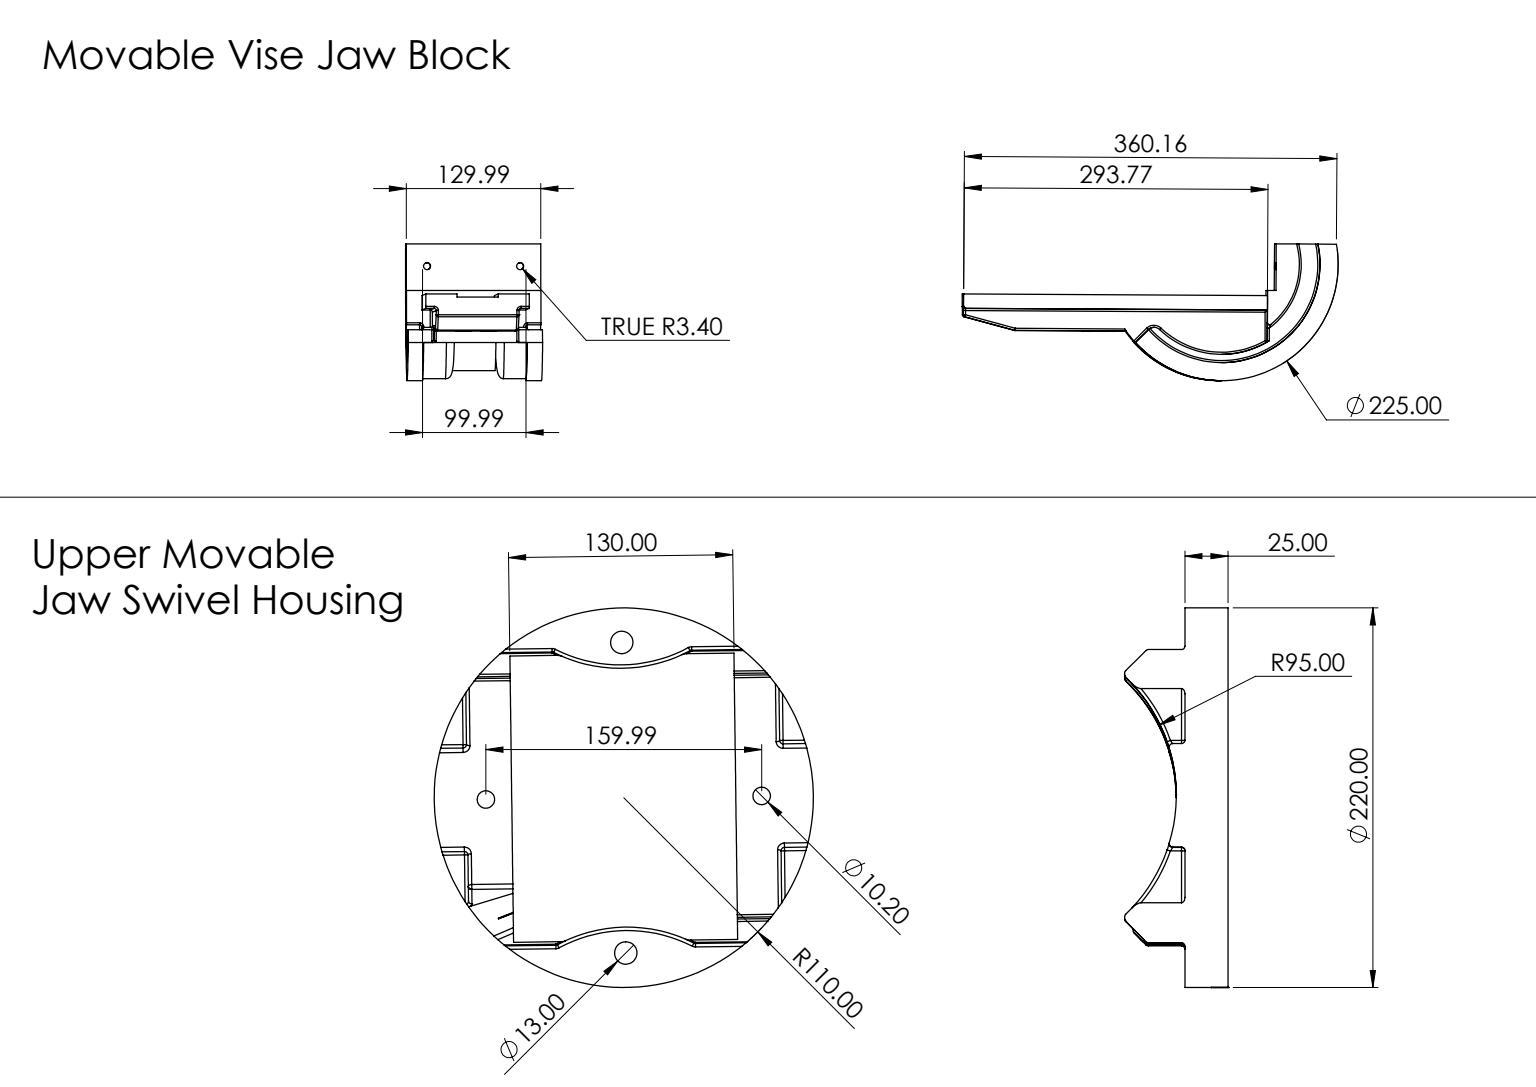
ISO-10303-21;
HEADER;
FILE_DESCRIPTION (('STEP AP214'),
    '1' );
FILE_NAME ('Upper Movable Jaw Swivel Housing.step',
    '2026-10-09T10:51:02',
    ( '' ),
    ( '' ),
    'SwSTEP 2.0',
    'SolidWorks 2026',
    '' );
FILE_SCHEMA (( 'AUTOMOTIVE_DESIGN' ));
ENDSEC;

DATA;
#10=CARTESIAN_POINT ( 'NONE',  ( -89.78468759032787716, 88.98018858692468314, 52.07678711320818365 ) ) ;
#12=VERTEX_POINT ( 'NONE', #2655 ) ;
#19=CARTESIAN_POINT ( 'NONE',  ( 83.88156715903123484, 75.05939835648034375, 2.283427986461537440 ) ) ;
#21=EDGE_LOOP ( 'NONE', ( #14279, #17712, #11551, #2632 ) ) ;
#25=CARTESIAN_POINT ( 'NONE',  ( -76.57490387278154742, 75.07748563434969924, 4.833641046600559044 ) ) ;
#28=CARTESIAN_POINT ( 'NONE',  ( -105.7487010638476619, 78.91327849199103639, 30.28586431387788380 ) ) ;
#37=DIRECTION ( 'NONE',  ( 6.641024085592512675E-15, -1.000000000000000000, 3.383900228611897455E-15 ) ) ;
#42=AXIS2_PLACEMENT_3D ( 'NONE', #16731, #4517, #8084 ) ;
#44=VERTEX_POINT ( 'NONE', #20325 ) ;
#50=AXIS2_PLACEMENT_3D ( 'NONE', #20682, #18849, #13474 ) ;
#51=CARTESIAN_POINT ( 'NONE',  ( -93.23587179807654479, 72.00000000000000000, -30.79757858250320979 ) ) ;
#57=CARTESIAN_POINT ( 'NONE',  ( 1.364373935098378649E-14, 105.0000000000000000, -9.836450281572198869E-15 ) ) ;
#58=EDGE_CURVE ( 'NONE', #6274, #3568, #1285, .T. ) ;
#59=CARTESIAN_POINT ( 'NONE',  ( 93.17671387018316409, 79.04398536104964990, 26.22064129356684958 ) ) ;
#65=EDGE_LOOP ( 'NONE', ( #10795, #9717, #10945, #15498 ) ) ;
#67=CARTESIAN_POINT ( 'NONE',  ( -92.91045972105430906, 79.04398536109844997, -26.22408268756080929 ) ) ;
#70=VECTOR ( 'NONE', #5389, 1000.000000000000000 ) ;
#71=CARTESIAN_POINT ( 'NONE',  ( -69.75324274910623501, 70.27959272172267902, -85.05633583411399457 ) ) ;
#84=VECTOR ( 'NONE', #2049, 1000.000000000000114 ) ;
#86=CARTESIAN_POINT ( 'NONE',  ( 70.93357090261925180, 91.46354453597338363, 84.07396062241133450 ) ) ;
#94=CARTESIAN_POINT ( 'NONE',  ( 87.98413419613014241, 100.6041916471018851, -66.02114910964037620 ) ) ;
#106=EDGE_CURVE ( 'NONE', #7605, #5654, #6985, .T. ) ;
#112=DIRECTION ( 'NONE',  ( 2.025474946048326158E-22, -1.000000000000000000, 1.876735158486679638E-22 ) ) ;
#114=DIRECTION ( 'NONE',  ( -0.9999164797902015955, -2.001050586450178695E-22, 0.01292414190464131335 ) ) ;
#133=CARTESIAN_POINT ( 'NONE',  ( -88.16866694100703228, 88.68864517119313007, 52.43947707082220688 ) ) ;
#142=CARTESIAN_POINT ( 'NONE',  ( 80.59620023633263486, 75.13519862315604314, -6.109066223056235145 ) ) ;
#146=ORIENTED_EDGE ( 'NONE', *, *, #11899, .T. ) ;
#157=PLANE ( 'NONE',  #21075 ) ;
#159=CARTESIAN_POINT ( 'NONE',  ( 105.4334892372614689, 71.72994009789539405, -31.36525700924963544 ) ) ;
#171=CARTESIAN_POINT ( 'NONE',  ( -90.06393689865117835, 72.00000000000000000, 59.85988923254397065 ) ) ;
#176=FACE_OUTER_BOUND ( 'NONE', #6477, .T. ) ;
#182=CARTESIAN_POINT ( 'NONE',  ( 92.53737097235195108, 79.85828562204582681, 28.87839056718317465 ) ) ;
#188=CARTESIAN_POINT ( 'NONE',  ( -92.67786813602107543, 77.16999450923083259, -28.87226322141232870 ) ) ;
#189=ORIENTED_EDGE ( 'NONE', *, *, #8901, .F. ) ;
#197=CARTESIAN_POINT ( 'NONE',  ( 1.163172771417732010, 44.99899999999999523, 89.99248318111813205 ) ) ;
#198=VERTEX_POINT ( 'NONE', #22578 ) ;
#202=CARTESIAN_POINT ( 'NONE',  ( -39.36913080622078809, 72.00000000000000000, 87.51612159803859470 ) ) ;
#204=CARTESIAN_POINT ( 'NONE',  ( -90.61229378181283778, 77.84360403296375353, 32.30868923918552582 ) ) ;
#214=EDGE_LOOP ( 'NONE', ( #14788, #8184, #10598, #16060, #20937 ) ) ;
#218=CARTESIAN_POINT ( 'NONE',  ( 36.24790013166018099, 94.37751527644310556, 82.16087381192814121 ) ) ;
#219=EDGE_CURVE ( 'NONE', #11742, #21224, #10193, .T. ) ;
#222=CYLINDRICAL_SURFACE ( 'NONE', #2944, 2.000000000000001776 ) ;
#226=CARTESIAN_POINT ( 'NONE',  ( -41.56623493000981284, 72.00000000000000000, -82.46967996629571473 ) ) ;
#230=CARTESIAN_POINT ( 'NONE',  ( 39.42082737383937996, 91.17157287525387233, -83.51645567887783272 ) ) ;
#231=ORIENTED_EDGE ( 'NONE', *, *, #5950, .F. ) ;
#232=CARTESIAN_POINT ( 'NONE',  ( 106.2491592972476298, 77.90302844854615216, 28.48020057081471279 ) ) ;
#235=EDGE_CURVE ( 'NONE', #9934, #22618, #12029, .T. ) ;
#236=EDGE_LOOP ( 'NONE', ( #19815, #2984, #795, #12420, #9588 ) ) ;
#240=EDGE_CURVE ( 'NONE', #22376, #21368, #5043, .T. ) ;
#243=CARTESIAN_POINT ( 'NONE',  ( -89.64611244253616462, 89.06139627483084098, 51.86061978640490366 ) ) ;
#247=EDGE_CURVE ( 'NONE', #11011, #13307, #20124, .T. ) ;
#253=CARTESIAN_POINT ( 'NONE',  ( -90.15100670864553933, 87.99029836822313655, 53.12346227685477373 ) ) ;
#265=CARTESIAN_POINT ( 'NONE',  ( 105.3069082217399597, 70.76149960027359498, -31.78775043357529739 ) ) ;
#271=EDGE_LOOP ( 'NONE', ( #6417, #19362, #17256, #12411 ) ) ;
#277=DIRECTION ( 'NONE',  ( 0.9999164797902017066, 2.001050586450178931E-22, -0.01292414190464131508 ) ) ;
#278=CARTESIAN_POINT ( 'NONE',  ( -91.88175745861167343, 69.99999999999998579, 60.48014731673399069 ) ) ;
#284=CARTESIAN_POINT ( 'NONE',  ( 90.70439626174579928, 79.29995750804924626, 27.08818539008225912 ) ) ;
#285=CARTESIAN_POINT ( 'NONE',  ( 90.15711184568685610, 79.46353706204938305, 27.61532001585838714 ) ) ;
#288=CIRCLE ( 'NONE', #22624, 0.009999999999999205705 ) ;
#289=ADVANCED_FACE ( 'NONE', ( #16063 ), #9015, .T. ) ;
#314=CARTESIAN_POINT ( 'NONE',  ( -91.08520856931303911, 77.44390114805533187, 31.69197020849769686 ) ) ;
#316=ORIENTED_EDGE ( 'NONE', *, *, #15570, .F. ) ;
#319=ADVANCED_FACE ( 'NONE', ( #17546 ), #8781, .T. ) ;
#325=DIRECTION ( 'NONE',  ( 0.01292414190464174703, 0.000000000000000000, 0.9999164797902015955 ) ) ;
#326=( BOUNDED_SURFACE ( )  B_SPLINE_SURFACE ( 3, 2, ( 
 ( #2487, #894, #11567 ),
 ( #1117, #14687, #22097 ),
 ( #11112, #18134, #9486 ),
 ( #2827, #8113, #7770 ),
 ( #14809, #13081, #4304 ),
 ( #11333, #16646, #14924 ),
 ( #998, #21864, #6160 ),
 ( #13185, #2385, #20151 ),
 ( #18461, #2723, #4540 ),
 ( #9377, #16853, #16751 ),
 ( #15145, #7985, #15025 ),
 ( #21979, #6279, #13305 ),
 ( #6398, #19810, #16411 ),
 ( #10404, #6504, #1347 ),
 ( #4752, #11794, #13518 ),
 ( #6725, #18893, #10288 ),
 ( #3156, #15697, #11911 ),
 ( #15366, #3390, #10171 ) ),
 .UNSPECIFIED., .F., .F., .T. ) 
 B_SPLINE_SURFACE_WITH_KNOTS ( ( 4, 2, 2, 2, 2, 2, 2, 2, 4 ),
 ( 3, 3 ),
 ( 0.002597246120634449582, 0.003399884678228176898, 0.004202523235821904214, 0.005005161793415631097, 0.005807800351009358847, 0.006610438908603086597, 0.007413077466196813479, 0.008215716023790540362, 0.009018354581384268112 ),
 ( 0.000000000000000000, 1.000000000000000000 ),
 .UNSPECIFIED. ) 
 GEOMETRIC_REPRESENTATION_ITEM ( )  RATIONAL_B_SPLINE_SURFACE ( (
 ( 1.000000000000000000, 0.5963808372950818448, 1.000000000000000000),
 ( 1.000000000000000000, 0.5963839598475944026, 1.000000000000000000),
 ( 1.000000000000000000, 0.5970886094881097117, 1.000000000000000000),
 ( 1.000000000000000000, 0.5998681984912884735, 1.000000000000000000),
 ( 1.000000000000000000, 0.6019790828716350406, 1.000000000000000000),
 ( 1.000000000000000000, 0.6074656362385489894, 1.000000000000000000),
 ( 1.000000000000000000, 0.6108290540004600588, 1.000000000000000000),
 ( 1.000000000000000000, 0.6188252630046860991, 1.000000000000000000),
 ( 1.000000000000000000, 0.6234423941984682527, 1.000000000000000000),
 ( 1.000000000000000000, 0.6335838931037546251, 1.000000000000000000),
 ( 1.000000000000000000, 0.6391861101558512503, 1.000000000000000000),
 ( 1.000000000000000000, 0.6512661799274815921, 1.000000000000000000),
 ( 1.000000000000000000, 0.6576333021889211317, 1.000000000000000000),
 ( 1.000000000000000000, 0.6710088154584188391, 1.000000000000000000),
 ( 1.000000000000000000, 0.6780884601156443869, 1.000000000000000000),
 ( 1.000000000000000000, 0.6924279500034885571, 1.000000000000000000),
 ( 1.000000000000000000, 0.6997125326201816264, 1.000000000000000000),
 ( 1.000000000000000000, 0.7071067811865476838, 1.000000000000000000) ) ) 
 REPRESENTATION_ITEM ( '' )  SURFACE ( )  );
#331=DIRECTION ( 'NONE',  ( 2.025474946048326158E-22, -1.000000000000000000, 1.876735158486679638E-22 ) ) ;
#334=ORIENTED_EDGE ( 'NONE', *, *, #20168, .F. ) ;
#354=CARTESIAN_POINT ( 'NONE',  ( -89.81089220510853011, 88.95379388444949598, 52.12444704693557895 ) ) ;
#356=ORIENTED_EDGE ( 'NONE', *, *, #20168, .T. ) ;
#367=VERTEX_POINT ( 'NONE', #15252 ) ;
#369=VERTEX_POINT ( 'NONE', #17174 ) ;
#371=CARTESIAN_POINT ( 'NONE',  ( -93.21002351426726307, 77.12912189496638860, -28.79774562292281104 ) ) ;
#387=ORIENTED_EDGE ( 'NONE', *, *, #12460, .T. ) ;
#390=DIRECTION ( 'NONE',  ( 0.01292414190464223969, 1.902755938799532355E-22, 0.9999164797902017066 ) ) ;
#392=CARTESIAN_POINT ( 'NONE',  ( 91.23603883849617091, 72.00000000000000000, 30.82342686631245243 ) ) ;
#393=CARTESIAN_POINT ( 'NONE',  ( -36.73936676148915126, 94.93197183469659706, -81.60001862646660697 ) ) ;
#396=EDGE_CURVE ( 'NONE', #4308, #9861, #9699, .T. ) ;
#397=CARTESIAN_POINT ( 'NONE',  ( 106.2089377515399065, 34.61572286322119396, 28.62973177816241588 ) ) ;
#400=CARTESIAN_POINT ( 'NONE',  ( 89.22767861003023881, 80.31838830481380853, 30.18953644180654550 ) ) ;
#403=CARTESIAN_POINT ( 'NONE',  ( 90.51972003054841309, 79.34791451281842001, 27.24428967784124822 ) ) ;
#405=CARTESIAN_POINT ( 'NONE',  ( -90.43474204040838060, 34.61572286322119396, 31.17139488067998343 ) ) ;
#412=CARTESIAN_POINT ( 'NONE',  ( -92.63973831233892042, 79.05196971970110553, -26.25410855708505409 ) ) ;
#419=DIRECTION ( 'NONE',  ( 0.01292414190464174703, 0.000000000000000000, 0.9999164797902015955 ) ) ;
#421=B_SPLINE_CURVE_WITH_KNOTS ( 'NONE', 3,
 ( #14409, #16130, #12222, #12679, #7032, #7150, #17960, #15907, #14177, #10490, #10589, #5523, #10835, #2094, #19205, #17501, #21045, #3916, #2196, #14060, #5402, #19548, #5298, #3815, #12338, #1753, #8731, #9199, #15785, #25, #12439, #17614, #19428, #19318, #3578, #7364, #16247, #488, #13932, #20926 ),
 .UNSPECIFIED., .F., .F.,
 ( 4, 2, 2, 2, 2, 2, 2, 2, 2, 2, 2, 2, 2, 2, 2, 2, 2, 2, 2, 4 ),
 ( 0.000000000000000000, 0.0009967370484891052360, 0.001495105572733637905, 0.001993474096978170573, 0.002990211145467237645, 0.003986948193956304717, 0.004983685242445371789, 0.005980422290934439729, 0.006977159339423508536, 0.007973896387912576475, 0.008970633436401644414, 0.009967370484890712354, 0.01046573900913524806, 0.01096410753337978203, 0.01196084458186887425, 0.01295758163035796821, 0.01345595015460251433, 0.01395431867884706391, 0.01495105572733619430, 0.01594779277582532642 ),
 .UNSPECIFIED. ) ;
#423=EDGE_CURVE ( 'NONE', #8239, #10113, #17733, .T. ) ;
#430=CARTESIAN_POINT ( 'NONE',  ( 67.52146002153375548, 70.28876377827108968, -86.83823687282567505 ) ) ;
#432=CARTESIAN_POINT ( 'NONE',  ( -91.92966151681214626, 79.05204536692272654, 28.63995821788555318 ) ) ;
#433=DIRECTION ( 'NONE',  ( -0.009138748381789112835, -0.7071067811865462405, -0.7070477234798343558 ) ) ;
#450=DIRECTION ( 'NONE',  ( 0.9999164797902015955, 2.001050586450177755E-22, -0.01292414190464177999 ) ) ;
#453=SPHERICAL_SURFACE ( 'NONE', #18447, 2.000000000000000000 ) ;
#462=CARTESIAN_POINT ( 'NONE',  ( 33.37693045445141138, 92.26126280267001789, 80.91304515629593652 ) ) ;
#464=( BOUNDED_CURVE ( )  B_SPLINE_CURVE ( 3, ( #5130, #22567, #8806, #20870 ),
 .UNSPECIFIED., .F., .T. ) 
 B_SPLINE_CURVE_WITH_KNOTS ( ( 4, 4 ),
 ( 0.4229686233981272414, 0.4841788640348457240 ),
 .UNSPECIFIED. ) 
 CURVE ( )  GEOMETRIC_REPRESENTATION_ITEM ( )  RATIONAL_B_SPLINE_CURVE ( ( 1.000000000000000000, 0.9996877999070342691, 0.9996877999070342691, 1.000000000000000000 ) ) 
 REPRESENTATION_ITEM ( '' )  );
#469=ORIENTED_EDGE ( 'NONE', *, *, #9836, .T. ) ;
#471=CARTESIAN_POINT ( 'NONE',  ( -88.41249021357108973, 88.83782181376912490, 50.51791556700484165 ) ) ;
#474=ORIENTED_EDGE ( 'NONE', *, *, #3932, .F. ) ;
#476=ORIENTED_EDGE ( 'NONE', *, *, #5316, .T. ) ;
#477=CARTESIAN_POINT ( 'NONE',  ( 1.079165849037564184, 44.99899999999999523, 83.49302606248181746 ) ) ;
#482=CARTESIAN_POINT ( 'NONE',  ( -91.45377919752192497, 96.73472523270000067, -61.12462174243600543 ) ) ;
#488=CARTESIAN_POINT ( 'NONE',  ( -79.25692431500161206, 75.13518351147564545, 6.091477897721252255 ) ) ;
#491=ORIENTED_EDGE ( 'NONE', *, *, #17530, .T. ) ;
#493=CARTESIAN_POINT ( 'NONE',  ( -14.05322407132952733, 63.29827626019820741, -14.85614898258057082 ) ) ;
#495=VERTEX_POINT ( 'NONE', #14623 ) ;
#496=EDGE_CURVE ( 'NONE', #21893, #14619, #12233, .T. ) ;
#503=CARTESIAN_POINT ( 'NONE',  ( -105.3515605809558195, 70.97896074530378030, 31.63944816216639211 ) ) ;
#507=CARTESIAN_POINT ( 'NONE',  ( 64.99457118636311748, 105.0000000000000000, -0.8400692238016954638 ) ) ;
#510=EDGE_CURVE ( 'NONE', #4157, #19786, #3544, .T. ) ;
#521=CIRCLE ( 'NONE', #1629, 1.999999999999999112 ) ;
#527=EDGE_LOOP ( 'NONE', ( #22645, #19170, #20971, #3651 ) ) ;
#529=FACE_OUTER_BOUND ( 'NONE', #7929, .T. ) ;
#531=CARTESIAN_POINT ( 'NONE',  ( -70.91392079944854743, 72.00000000000000000, -84.09052168258642723 ) ) ;
#541=EDGE_CURVE ( 'NONE', #17177, #9516, #1391, .T. ) ;
#542=ORIENTED_EDGE ( 'NONE', *, *, #423, .F. ) ;
#550=CARTESIAN_POINT ( 'NONE',  ( -90.51365344713411787, 78.00107869518899406, 32.54507930669932847 ) ) ;
#554=CIRCLE ( 'NONE', #5300, 2.000000000000001332 ) ;
#562=ORIENTED_EDGE ( 'NONE', *, *, #13386, .T. ) ;
#567=VERTEX_POINT ( 'NONE', #9777 ) ;
#571=B_SPLINE_CURVE_WITH_KNOTS ( 'NONE', 3,
 ( #10519, #14093, #4058, #7523, #13059, #2579, #6135, #8528, #22192, #20710, #11994, #22553 ),
 .UNSPECIFIED., .F., .F.,
 ( 4, 2, 2, 2, 2, 4 ),
 ( 0.000000000000000000, 0.0007983727002588449344, 0.001596745400517689869, 0.003193490801035376702, 0.004790236201553063969, 0.006386981602070762078 ),
 .UNSPECIFIED. ) ;
#572=ORIENTED_EDGE ( 'NONE', *, *, #22537, .F. ) ;
#575=DIRECTION ( 'NONE',  ( 0.01292414190464179213, 0.000000000000000000, 0.9999164797902017066 ) ) ;
#577=DIRECTION ( 'NONE',  ( 0.8585559824929073214, 0.4417096956421488474, -0.2603347262686231400 ) ) ;
#578=AXIS2_PLACEMENT_3D ( 'NONE', #9864, #20311, #8020 ) ;
#580=CARTESIAN_POINT ( 'NONE',  ( 92.43457499998882554, 79.86121811340028387, -31.19724316448930423 ) ) ;
#586=ORIENTED_EDGE ( 'NONE', *, *, #9607, .F. ) ;
#588=CARTESIAN_POINT ( 'NONE',  ( -88.17180307448359144, 88.85327758763604322, 52.12627907722180254 ) ) ;
#591=VERTEX_POINT ( 'NONE', #17124 ) ;
#600=ORIENTED_EDGE ( 'NONE', *, *, #3820, .F. ) ;
#601=CARTESIAN_POINT ( 'NONE',  ( 92.13597290369317250, 77.31823782845360427, 29.12178019517720884 ) ) ;
#602=ORIENTED_EDGE ( 'NONE', *, *, #541, .F. ) ;
#613=FACE_OUTER_BOUND ( 'NONE', #11627, .T. ) ;
#615=ORIENTED_EDGE ( 'NONE', *, *, #11170, .T. ) ;
#616=CARTESIAN_POINT ( 'NONE',  ( -84.91224671543740499, 75.00866199770878495, 2.421235374481680136 ) ) ;
#618=CARTESIAN_POINT ( 'NONE',  ( -88.16310690832857233, 88.22405785602812500, 52.94336900718522543 ) ) ;
#623=CARTESIAN_POINT ( 'NONE',  ( 41.56623493000984126, 69.99999999999998579, 82.46967996629570052 ) ) ;
#624=CARTESIAN_POINT ( 'NONE',  ( -41.01898768785987670, 92.04141378167193466, -84.43550307159648582 ) ) ;
#626=CARTESIAN_POINT ( 'NONE',  ( 93.23587179807657321, 69.99999999999998579, 30.79757858250317781 ) ) ;
#627=LINE ( 'NONE', #11303, #11518 ) ;
#629=CARTESIAN_POINT ( 'NONE',  ( 81.70668847916368804, 104.4142135623730780, -73.64792636435126383 ) ) ;
#644=CARTESIAN_POINT ( 'NONE',  ( -88.92875819446121000, 70.43566758519529003, 63.01298426280252585 ) ) ;
#647=ADVANCED_FACE ( 'NONE', ( #18837 ), #13561, .F. ) ;
#657=DIRECTION ( 'NONE',  ( 0.9999164797902015955, 2.001050586450178695E-22, -0.01292414190464131335 ) ) ;
#659=CARTESIAN_POINT ( 'NONE',  ( -90.46145803317399725, 80.27058204906346361, 32.37524683357860056 ) ) ;
#661=ORIENTED_EDGE ( 'NONE', *, *, #9836, .F. ) ;
#668=CARTESIAN_POINT ( 'NONE',  ( -90.40889375659909888, 78.43035437438882695, 33.17122784026039994 ) ) ;
#672=EDGE_CURVE ( 'NONE', #7269, #15892, #7114, .T. ) ;
#677=CARTESIAN_POINT ( 'NONE',  ( -85.63433794141032251, 105.0000000000000000, -69.04172771111927887 ) ) ;
#685=ORIENTED_EDGE ( 'NONE', *, *, #18084, .T. ) ;
#686=PLANE ( 'NONE',  #15863 ) ;
#689=CARTESIAN_POINT ( 'NONE',  ( 35.95309506732430549, 93.50464841319750064, 82.03286182426640494 ) ) ;
#692=DIRECTION ( 'NONE',  ( -0.9999164797902015955, -2.001050586450178695E-22, 0.01292414190464131335 ) ) ;
#694=ORIENTED_EDGE ( 'NONE', *, *, #2604, .T. ) ;
#696=DIRECTION ( 'NONE',  ( 0.9999164797902017066, 0.000000000000000000, -0.01292414190464174703 ) ) ;
#697=CARTESIAN_POINT ( 'NONE',  ( -88.29917401736820182, 88.77742970155978242, 50.41907810135165846 ) ) ;
#699=AXIS2_PLACEMENT_3D ( 'NONE', #1518, #3671, #16004 ) ;
#702=CARTESIAN_POINT ( 'NONE',  ( -91.00106904273528130, 70.29040131071506892, 61.79648398638329354 ) ) ;
#708=CARTESIAN_POINT ( 'NONE',  ( 69.24448582912822303, 92.41827837429551096, -85.47053766693686327 ) ) ;
#709=ORIENTED_EDGE ( 'NONE', *, *, #772, .F. ) ;
#711=DIRECTION ( 'NONE',  ( -0.01292414190464269072, 0.000000000000000000, -0.9999164797902017066 ) ) ;
#722=FACE_OUTER_BOUND ( 'NONE', #6782, .T. ) ;
#723=DIRECTION ( 'NONE',  ( 0.9999164797902015955, 2.001050586450178695E-22, -0.01292414190464131335 ) ) ;
#729=CARTESIAN_POINT ( 'NONE',  ( -85.06887357168608332, 75.00176710950381676, 0.4346775517040236680 ) ) ;
#732=ORIENTED_EDGE ( 'NONE', *, *, #9607, .T. ) ;
#733=ORIENTED_EDGE ( 'NONE', *, *, #1086, .F. ) ;
#736=DIRECTION ( 'NONE',  ( 0.01292414190463832269, 0.000000000000000000, 0.9999164797902017066 ) ) ;
#739=DIRECTION ( 'NONE',  ( -0.9999164797902017066, -2.001050586450178931E-22, 0.01292414190464131508 ) ) ;
#740=CARTESIAN_POINT ( 'NONE',  ( -38.37734285177536009, 94.19957547782772167, -82.31130495469157893 ) ) ;
#750=AXIS2_PLACEMENT_3D ( 'NONE', #20210, #20433, #18609 ) ;
#755=ORIENTED_EDGE ( 'NONE', *, *, #16128, .F. ) ;
#758=ORIENTED_EDGE ( 'NONE', *, *, #13735, .T. ) ;
#760=CARTESIAN_POINT ( 'NONE',  ( 77.23768650000880598, 75.09868225356437677, -5.328640597094168818 ) ) ;
#762=CIRCLE ( 'NONE', #16898, 109.9999999999999858 ) ;
#767=CARTESIAN_POINT ( 'NONE',  ( -68.86686855361774917, 91.87224768293378929, 85.77506393453893452 ) ) ;
#769=CARTESIAN_POINT ( 'NONE',  ( 36.55288090549195346, 94.02752048664900997, -83.45186405039071076 ) ) ;
#770=PRODUCT_DEFINITION_FORMATION_WITH_SPECIFIED_SOURCE ( 'ANY', '', #21141, .NOT_KNOWN. ) ;
#772=EDGE_CURVE ( 'NONE', #9297, #6510, #5371, .T. ) ;
#776=AXIS2_PLACEMENT_3D ( 'NONE', #10622, #7405, #14094 ) ;
#778=EDGE_LOOP ( 'NONE', ( #21060, #476, #15475, #9549 ) ) ;
#781=LINE ( 'NONE', #13421, #11777 ) ;
#784=VERTEX_POINT ( 'NONE', #16095 ) ;
#786=CARTESIAN_POINT ( 'NONE',  ( -73.02363241441464936, 95.86457595575431867, 79.19170252361408302 ) ) ;
#795=ORIENTED_EDGE ( 'NONE', *, *, #6607, .F. ) ;
#806=CARTESIAN_POINT ( 'NONE',  ( -6.720435043957357024, 86.44819594746830660, 75.42837923485861040 ) ) ;
#807=ORIENTED_EDGE ( 'NONE', *, *, #20974, .F. ) ;
#815=SPHERICAL_SURFACE ( 'NONE', #10974, 2.000000000000000000 ) ;
#817=CARTESIAN_POINT ( 'NONE',  ( -89.31453485712998486, 89.12573045752694156, 51.42325317176502608 ) ) ;
#829=CARTESIAN_POINT ( 'NONE',  ( 1.117803423002105445, 45.00000000000000000, 109.6947150755565161 ) ) ;
#831=ORIENTED_EDGE ( 'NONE', *, *, #22112, .T. ) ;
#833=CARTESIAN_POINT ( 'NONE',  ( 33.79255210837673928, 93.51775827232350480, -82.92153020431163668 ) ) ;
#836=CARTESIAN_POINT ( 'NONE',  ( -91.27111462898957939, 78.10400798472785766, -30.35002675991158938 ) ) ;
#843=CARTESIAN_POINT ( 'NONE',  ( -64.99457118636308905, 169.9999999999999716, 0.8400692238016759239 ) ) ;
#847=CIRCLE ( 'NONE', #19145, 2.000000000000004441 ) ;
#851=CARTESIAN_POINT ( 'NONE',  ( -105.3069082217399455, 70.76149960027362340, 31.78775043357526187 ) ) ;
#852=CARTESIAN_POINT ( 'NONE',  ( -90.15962223546766552, 87.22510259077962758, 51.26146238794839149 ) ) ;
#860=CARTESIAN_POINT ( 'NONE',  ( -75.37743570715805674, 94.88086180942337933, 80.20674419475355421 ) ) ;
#861=DIRECTION ( 'NONE',  ( 0.01292414190464174703, 0.000000000000000000, 0.9999164797902015955 ) ) ;
#862=CARTESIAN_POINT ( 'NONE',  ( -37.86419661077498944, 93.64690829566940522, -82.87065082828767970 ) ) ;
#873=VECTOR ( 'NONE', #11813, 1000.000000000000227 ) ;
#875=DIRECTION ( 'NONE',  ( -2.025474946048326158E-22, 1.000000000000000000, -1.876735158486679638E-22 ) ) ;
#878=EDGE_LOOP ( 'NONE', ( #10525, #21495, #15616, #936 ) ) ;
#880=EDGE_CURVE ( 'NONE', #13498, #2805, #21780, .T. ) ;
#885=CARTESIAN_POINT ( 'NONE',  ( -40.63089462960165577, 93.08398165842315564, -83.39786430079456636 ) ) ;
#886=DIRECTION ( 'NONE',  ( -0.01292414190463830014, 0.000000000000000000, -0.9999164797902017066 ) ) ;
#894=CARTESIAN_POINT ( 'NONE',  ( 92.43457499998879712, 79.82103140525723006, -31.19724316448930779 ) ) ;
#899=VERTEX_POINT ( 'NONE', #14373 ) ;
#903=ORIENTED_EDGE ( 'NONE', *, *, #7212, .F. ) ;
#906=AXIS2_PLACEMENT_3D ( 'NONE', #11247, #15610, #15544 ) ;
#913=ORIENTED_EDGE ( 'NONE', *, *, #21546, .T. ) ;
#930=CARTESIAN_POINT ( 'NONE',  ( 39.75021781620444727, 72.00000000000000000, 86.03367798009509215 ) ) ;
#931=CARTESIAN_POINT ( 'NONE',  ( -88.18132310388985218, 88.98978577205728868, 51.06603758169391227 ) ) ;
#936=ORIENTED_EDGE ( 'NONE', *, *, #3583, .F. ) ;
#943=CARTESIAN_POINT ( 'NONE',  ( -91.62437796271720458, 95.71196945526502020, -60.86849236629026905 ) ) ;
#947=ORIENTED_EDGE ( 'NONE', *, *, #2604, .F. ) ;
#949=CARTESIAN_POINT ( 'NONE',  ( 86.44937305384745230, 104.7459436402722446, 68.01917747034273987 ) ) ;
#952=EDGE_CURVE ( 'NONE', #10157, #10387, #19843, .T. ) ;
#954=CARTESIAN_POINT ( 'NONE',  ( 41.56623493000984126, 72.00000000000000000, 82.46967996629570052 ) ) ;
#959=VERTEX_POINT ( 'NONE', #18359 ) ;
#962=CARTESIAN_POINT ( 'NONE',  ( -90.17329558876596707, 87.04737729605604102, 51.36928819417873626 ) ) ;
#971=CARTESIAN_POINT ( 'NONE',  ( 40.65822637310714782, 72.00000000000000000, 84.25167897319538213 ) ) ;
#983=DIRECTION ( 'NONE',  ( 0.9999164797902017066, 0.000000000000000000, -0.01292414190464174703 ) ) ;
#984=VERTEX_POINT ( 'NONE', #6723 ) ;
#988=ORIENTED_EDGE ( 'NONE', *, *, #2448, .F. ) ;
#989=CARTESIAN_POINT ( 'NONE',  ( 75.19375158121341940, 75.01682528584527176, -2.766602073185969957 ) ) ;
#998=CARTESIAN_POINT ( 'NONE',  ( 91.40888322292899204, 77.29711350638434908, -31.45985873596572446 ) ) ;
#1008=EDGE_LOOP ( 'NONE', ( #15966, #9563, #11679, #21258, #21126, #1572 ) ) ;
#1017=EDGE_CURVE ( 'NONE', #1815, #3120, #15233, .T. ) ;
#1019=CARTESIAN_POINT ( 'NONE',  ( -106.2880716433168828, 78.18499655656300718, -28.33463432393061154 ) ) ;
#1026=EDGE_LOOP ( 'NONE', ( #2409, #12741, #5552, #13266 ) ) ;
#1033=ORIENTED_EDGE ( 'NONE', *, *, #10803, .F. ) ;
#1038=CARTESIAN_POINT ( 'NONE',  ( -110.8786557059970477, 104.3814432989690602, -67.26907703621752432 ) ) ;
#1041=DIRECTION ( 'NONE',  ( 2.025474946048326158E-22, -1.000000000000000000, 1.876735158486679638E-22 ) ) ;
#1046=CARTESIAN_POINT ( 'NONE',  ( 36.23709397917762942, 94.19957547783377549, -83.27571307199191608 ) ) ;
#1048=ORIENTED_EDGE ( 'NONE', *, *, #2448, .T. ) ;
#1049=DIRECTION ( 'NONE',  ( 1.387778780781444413E-14, -1.000000000000000000, 0.000000000000000000 ) ) ;
#1051=CARTESIAN_POINT ( 'NONE',  ( 1.364374644014609697E-14, 69.99999999999998579, -9.836443712999143722E-15 ) ) ;
#1057=AXIS2_PLACEMENT_3D ( 'NONE', #17259, #18859, #15329 ) ;
#1061=VECTOR ( 'NONE', #1259, 1000.000000000000114 ) ;
#1065=CARTESIAN_POINT ( 'NONE',  ( -88.16170457043438091, 88.05983001323437520, 53.05667506944086398 ) ) ;
#1066=( BOUNDED_CURVE ( )  B_SPLINE_CURVE ( 3, ( #22591, #1958, #12314, #3328 ),
 .UNSPECIFIED., .F., .T. ) 
 B_SPLINE_CURVE_WITH_KNOTS ( ( 4, 4 ),
 ( 5.799006443144740786, 5.860216683781459324 ),
 .UNSPECIFIED. ) 
 CURVE ( )  GEOMETRIC_REPRESENTATION_ITEM ( )  RATIONAL_B_SPLINE_CURVE ( ( 1.000000000000000000, 0.9996877999070342691, 0.9996877999070342691, 1.000000000000000000 ) ) 
 REPRESENTATION_ITEM ( '' )  );
#1070=DIRECTION ( 'NONE',  ( -0.9999164797902015955, -2.001050586450178695E-22, 0.01292414190464131335 ) ) ;
#1076=CARTESIAN_POINT ( 'NONE',  ( -91.41602376139164221, 79.08283919787463390, 28.73514828341261662 ) ) ;
#1086=EDGE_CURVE ( 'NONE', #15798, #10332, #4842, .T. ) ;
#1091=CARTESIAN_POINT ( 'NONE',  ( -63.99205529224568068, 99.43075776215394512, 78.40283286226222970 ) ) ;
#1096=EDGE_LOOP ( 'NONE', ( #20372, #6109, #189, #21429 ) ) ;
#1097=MECHANICAL_DESIGN_GEOMETRIC_PRESENTATION_REPRESENTATION('',(#11729),#3275);
#1099=LINE ( 'NONE', #8092, #15599 ) ;
#1100=CIRCLE ( 'NONE', #16873, 5.099999999999994316 ) ;
#1104=DIRECTION ( 'NONE',  ( 0.8585559824929073214, 0.4417096956421488474, -0.2603347262686231400 ) ) ;
#1105=CARTESIAN_POINT ( 'NONE',  ( 79.92740525950247843, 75.13699351169599083, -6.133505399301336425 ) ) ;
#1107=CARTESIAN_POINT ( 'NONE',  ( -109.5443584724615960, 75.69229587323862063, -10.26624083857044134 ) ) ;
#1117=CARTESIAN_POINT ( 'NONE',  ( 92.29888966083395019, 77.12912189587973444, -31.19548940143703675 ) ) ;
#1122=ORIENTED_EDGE ( 'NONE', *, *, #20034, .F. ) ;
#1127=ORIENTED_EDGE ( 'NONE', *, *, #21240, .T. ) ;
#1129=VECTOR ( 'NONE', #21193, 1000.000000000000114 ) ;
#1131=EDGE_CURVE ( 'NONE', #6487, #11658, #18763, .T. ) ;
#1141=CARTESIAN_POINT ( 'NONE',  ( 38.89810712971356566, 69.99999999999998579, -85.50986645835283184 ) ) ;
#1146=LINE ( 'NONE', #22234, #5899 ) ;
#1148=FACE_OUTER_BOUND ( 'NONE', #16881, .T. ) ;
#1149=CARTESIAN_POINT ( 'NONE',  ( -80.05923150692979107, 55.00000000000000000, -4.065642694558677661 ) ) ;
#1150=VECTOR ( 'NONE', #15189, 1000.000000000000000 ) ;
#1155=FACE_OUTER_BOUND ( 'NONE', #14073, .T. ) ;
#1156=ADVANCED_FACE ( 'NONE', ( #10257 ), #10710, .T. ) ;
#1165=CARTESIAN_POINT ( 'NONE',  ( 79.99331838321614896, 54.99999999999999289, -1.033931352371314949 ) ) ;
#1171=EDGE_LOOP ( 'NONE', ( #14955, #831, #12321, #20178 ) ) ;
#1172=CARTESIAN_POINT ( 'NONE',  ( 38.46706438352715196, 91.17157287525387233, -85.27439087629285552 ) ) ;
#1173=CARTESIAN_POINT ( 'NONE',  ( 1.079165849037564184, 45.00000000000000000, 83.49302606248181746 ) ) ;
#1175=ORIENTED_EDGE ( 'NONE', *, *, #15574, .T. ) ;
#1176=DIRECTION ( 'NONE',  ( 0.9999164797902015955, 2.001050586450178695E-22, -0.01292414190464131335 ) ) ;
#1177=CARTESIAN_POINT ( 'NONE',  ( -90.00466877033377955, 70.05991977044968166, 63.23890890537643372 ) ) ;
#1178=CYLINDRICAL_SURFACE ( 'NONE', #8706, 2.000000000000001332 ) ;
#1190=CARTESIAN_POINT ( 'NONE',  ( -88.16543564968796431, 88.44947730819713172, 52.74183542837116789 ) ) ;
#1193=ORIENTED_EDGE ( 'NONE', *, *, #10277, .F. ) ;
#1195=CARTESIAN_POINT ( 'NONE',  ( -75.01996951961029936, 95.34343679383250958, 80.44883674393967965 ) ) ;
#1197=CARTESIAN_POINT ( 'NONE',  ( -7.151472223503956727, 86.33655068423909995, -75.12481784635232884 ) ) ;
#1223=EDGE_CURVE ( 'NONE', #14542, #16639, #421, .T. ) ;
#1227=VECTOR ( 'NONE', #114, 1000.000000000000114 ) ;
#1240=DIRECTION ( 'NONE',  ( -2.025474946048326158E-22, 1.000000000000000000, -1.876735158486679638E-22 ) ) ;
#1252=AXIS2_PLACEMENT_3D ( 'NONE', #51, #5550, #19227 ) ;
#1259=DIRECTION ( 'NONE',  ( 0.9999164797902015955, 4.653667080246435885E-16, -0.01292414190464177999 ) ) ;
#1263=DIRECTION ( 'NONE',  ( 3.469446951953611033E-15, 1.000000000000000000, 0.000000000000000000 ) ) ;
#1272=DIRECTION ( 'NONE',  ( -2.025474946048326158E-22, 1.000000000000000000, -1.876735158486679638E-22 ) ) ;
#1274=DIRECTION ( 'NONE',  ( 2.025474946048326158E-22, -1.000000000000000000, 1.876735158486679638E-22 ) ) ;
#1279=PRODUCT_CONTEXT ( 'NONE', #19520, 'mechanical' ) ;
#1280=AXIS2_PLACEMENT_3D ( 'NONE', #1801, #20431, #6334 ) ;
#1283=CIRCLE ( 'NONE', #19225, 1.999999999999997780 ) ;
#1285=LINE ( 'NONE', #4679, #5607 ) ;
#1292=CARTESIAN_POINT ( 'NONE',  ( 33.82085273160093664, 93.50464841319750064, -82.93470554904388337 ) ) ;
#1293=EDGE_LOOP ( 'NONE', ( #8266, #22233 ) ) ;
#1294=DIRECTION ( 'NONE',  ( -0.01292414190464022741, 0.000000000000000000, -0.9999164797902017066 ) ) ;
#1297=CARTESIAN_POINT ( 'NONE',  ( 106.1909711380429542, 71.47214965576931434, 28.69631340039671841 ) ) ;
#1301=EDGE_CURVE ( 'NONE', #17005, #20235, #11278, .T. ) ;
#1308=CARTESIAN_POINT ( 'NONE',  ( -89.99197688737933731, 88.74347365508511132, 52.47095576274720941 ) ) ;
#1315=CARTESIAN_POINT ( 'NONE',  ( -89.22767861003021039, 80.31838830481383695, -30.18953644180660234 ) ) ;
#1332=CARTESIAN_POINT ( 'NONE',  ( -64.34562386414329183, 87.00751446224754204, 51.04789940634336887 ) ) ;
#1338=CARTESIAN_POINT ( 'NONE',  ( -106.8724933792760652, 79.04398536104956463, -26.04362031086678897 ) ) ;
#1347=CARTESIAN_POINT ( 'NONE',  ( 88.62677304471942819, 79.89796367043616954, -31.25921585370831224 ) ) ;
#1351=CARTESIAN_POINT ( 'NONE',  ( 1.364374644014609697E-14, 69.99999999999998579, -9.836443712999143722E-15 ) ) ;
#1366=DIRECTION ( 'NONE',  ( -0.01292414190464132896, 0.000000000000000000, -0.9999164797902015955 ) ) ;
#1373=VERTEX_POINT ( 'NONE', #6775 ) ;
#1383=EDGE_CURVE ( 'NONE', #3455, #12065, #5163, .T. ) ;
#1388=ORIENTED_EDGE ( 'NONE', *, *, #17750, .F. ) ;
#1390=DIRECTION ( 'NONE',  ( -0.01292414190464218071, -1.902755938799532120E-22, -0.9999164797902017066 ) ) ;
#1391=LINE ( 'NONE', #11847, #17880 ) ;
#1394=VERTEX_POINT ( 'NONE', #8043 ) ;
#1395=DIRECTION ( 'NONE',  ( 1.000000000000000000, 0.000000000000000000, 0.000000000000000000 ) ) ;
#1403=AXIS2_PLACEMENT_3D ( 'NONE', #9251, #7191, #14220 ) ;
#1410=CARTESIAN_POINT ( 'NONE',  ( -90.10913265094163194, 87.45414967491383607, 51.12188757306625320 ) ) ;
#1415=CARTESIAN_POINT ( 'NONE',  ( -73.83063990018285949, 96.00169183596570122, 81.54214722377805913 ) ) ;
#1419=CARTESIAN_POINT ( 'NONE',  ( -88.17578298076553267, 88.98131632899244892, 51.70423481999122828 ) ) ;
#1425=CARTESIAN_POINT ( 'NONE',  ( -64.03197570747913403, 99.62212517233105302, 75.31426563926737572 ) ) ;
#1426=CARTESIAN_POINT ( 'NONE',  ( -88.18368518054532501, 87.00751446224754204, 51.35601162712541168 ) ) ;
#1427=CARTESIAN_POINT ( 'NONE',  ( 90.66698955146013361, 79.16774870435551748, -29.00429242512963768 ) ) ;
#1436=ORIENTED_EDGE ( 'NONE', *, *, #18757, .T. ) ;
#1444=ADVANCED_FACE ( 'NONE', ( #3203 ), #1178, .F. ) ;
#1461=DIRECTION ( 'NONE',  ( -0.5121193912974635332, 0.6668151060996380108, -0.5413791123920870252 ) ) ;
#1465=AXIS2_PLACEMENT_3D ( 'NONE', #17677, #2257, #5695 ) ;
#1467=AXIS2_PLACEMENT_3D ( 'NONE', #15140, #20727, #11671 ) ;
#1469=DIRECTION ( 'NONE',  ( 0.008205354412248750534, -0.7726059781012502015, 0.6348327927582032570 ) ) ;
#1471=AXIS2_PLACEMENT_3D ( 'NONE', #3974, #14819, #14586 ) ;
#1476=ORIENTED_EDGE ( 'NONE', *, *, #3480, .T. ) ;
#1481=CARTESIAN_POINT ( 'NONE',  ( 68.71681667565954399, 72.00000000000000000, -85.89527988174788220 ) ) ;
#1489=EDGE_CURVE ( 'NONE', #21811, #4404, #4303, .T. ) ;
#1496=AXIS2_PLACEMENT_3D ( 'NONE', #10517, #5668, #10619 ) ;
#1499=DIRECTION ( 'NONE',  ( -0.01292414190463832269, 0.000000000000000000, -0.9999164797902017066 ) ) ;
#1506=CARTESIAN_POINT ( 'NONE',  ( -86.79222083800951282, 104.3814432989690602, -67.58039954014913064 ) ) ;
#1510=DIRECTION ( 'NONE',  ( 0.9999164797902017066, 2.001050586450178695E-22, -0.01292414190464131508 ) ) ;
#1512=AXIS2_PLACEMENT_3D ( 'NONE', #12811, #16166, #19461 ) ;
#1515=ADVANCED_FACE ( 'NONE', ( #5036 ), #19055, .T. ) ;
#1518=CARTESIAN_POINT ( 'NONE',  ( 39.42082737383937996, 91.17157287525388654, -83.51645567887783272 ) ) ;
#1520=CARTESIAN_POINT ( 'NONE',  ( -88.16443613784075239, 88.35912761021998563, 52.83007831909758067 ) ) ;
#1521=VECTOR ( 'NONE', #6569, 1000.000000000000000 ) ;
#1528=CARTESIAN_POINT ( 'NONE',  ( -20.68543912716607736, 88.27010240781663697, -77.04715649662465182 ) ) ;
#1529=ORIENTED_EDGE ( 'NONE', *, *, #21240, .F. ) ;
#1530=CARTESIAN_POINT ( 'NONE',  ( 83.79153344593285624, 75.05951099091890910, -4.453614549308245962 ) ) ;
#1531=CARTESIAN_POINT ( 'NONE',  ( -70.91392079944854743, 91.32005360614647316, -84.09052168258642723 ) ) ;
#1534=FACE_OUTER_BOUND ( 'NONE', #12231, .T. ) ;
#1542=EDGE_CURVE ( 'NONE', #8847, #14836, #288, .T. ) ;
#1543=VECTOR ( 'NONE', #20457, 1000.000000000000000 ) ;
#1553=CARTESIAN_POINT ( 'NONE',  ( -90.06393689865117835, 72.00000000000000000, 59.85988923254397776 ) ) ;
#1555=CARTESIAN_POINT ( 'NONE',  ( -91.62437796271723300, 71.80839515725416788, -60.86849236629029036 ) ) ;
#1561=LINE ( 'NONE', #13631, #6036 ) ;
#1562=DIRECTION ( 'NONE',  ( -0.01292414190464022741, 0.000000000000000000, -0.9999164797902017066 ) ) ;
#1563=AXIS2_PLACEMENT_3D ( 'NONE', #15805, #5850, #3494 ) ;
#1570=CARTESIAN_POINT ( 'NONE',  ( -89.22443767324087105, 80.23075532867244419, -29.93879111800710646 ) ) ;
#1572=ORIENTED_EDGE ( 'NONE', *, *, #3820, .T. ) ;
#1581=VERTEX_POINT ( 'NONE', #10459 ) ;
#1588=CARTESIAN_POINT ( 'NONE',  ( 39.66847363096314893, 93.56461422141673268, 82.92963109642391828 ) ) ;
#1602=VECTOR ( 'NONE', #19277, 1000.000000000000114 ) ;
#1603=AXIS2_PLACEMENT_3D ( 'NONE', #9229, #4388, #14895 ) ;
#1613=CARTESIAN_POINT ( 'NONE',  ( 91.62437796271727564, 34.61572286322119396, 60.86849236629024773 ) ) ;
#1615=CARTESIAN_POINT ( 'NONE',  ( -89.50333764702355666, 88.30151482414257202, 50.59770125036460797 ) ) ;
#1616=EDGE_LOOP ( 'NONE', ( #15461, #11092, #3428 ) ) ;
#1618=PLANE ( 'NONE',  #19237 ) ;
#1623=VECTOR ( 'NONE', #1863, 1000.000000000000114 ) ;
#1629=AXIS2_PLACEMENT_3D ( 'NONE', #3300, #13778, #10441 ) ;
#1630=CARTESIAN_POINT ( 'NONE',  ( 90.07355500607899046, 71.53834005368396731, -63.14076745314238792 ) ) ;
#1631=CARTESIAN_POINT ( 'NONE',  ( -88.16398599203232322, 88.31536494695383510, 52.86903560245924183 ) ) ;
#1638=CARTESIAN_POINT ( 'NONE',  ( 1.717753310876221295, 45.00000000000000000, 109.6869605904137330 ) ) ;
#1641=B_SPLINE_CURVE_WITH_KNOTS ( 'NONE', 3,
 ( #11508, #20333, #14964, #2985, #2774, #14862, #19984, #1292 ),
 .UNSPECIFIED., .F., .F.,
 ( 4, 2, 2, 4 ),
 ( 6.938893903907228378E-18, 0.001422831528841437491, 0.002134247293262152984, 0.002845663057682868043 ),
 .UNSPECIFIED. ) ;
#1655=DIRECTION ( 'NONE',  ( 0.01220060921879500236, -0.3298969072164960603, 0.9439381207174974975 ) ) ;
#1656=CARTESIAN_POINT ( 'NONE',  ( 105.4170939775132894, 71.46263312473240603, -31.42050039360495006 ) ) ;
#1667=FACE_OUTER_BOUND ( 'NONE', #18510, .T. ) ;
#1668=ORIENTED_EDGE ( 'NONE', *, *, #1017, .F. ) ;
#1676=VECTOR ( 'NONE', #17134, 1000.000000000000114 ) ;
#1679=CARTESIAN_POINT ( 'NONE',  ( 33.82085273160093664, 93.50464841319750064, -82.93470554904388337 ) ) ;
#1683=EDGE_CURVE ( 'NONE', #11404, #11011, #10571, .T. ) ;
#1724=CARTESIAN_POINT ( 'NONE',  ( -89.68778923927422397, 88.14345933540539590, 50.69680520791115441 ) ) ;
#1726=CARTESIAN_POINT ( 'NONE',  ( 106.6839260360358992, 79.12661604778581648, 26.80604816241556065 ) ) ;
#1728=DIRECTION ( 'NONE',  ( 0.9999164797902015955, 0.000000000000000000, -0.01292414190464174703 ) ) ;
#1729=ORIENTED_EDGE ( 'NONE', *, *, #10659, .T. ) ;
#1731=CARTESIAN_POINT ( 'NONE',  ( 91.23603883849617091, 69.99999999999998579, 30.82342686631245954 ) ) ;
#1736=ORIENTED_EDGE ( 'NONE', *, *, #10040, .F. ) ;
#1738=CARTESIAN_POINT ( 'NONE',  ( -88.17040607254148199, 88.78744216278629153, 52.26814626353031912 ) ) ;
#1739=DIRECTION ( 'NONE',  ( 0.009138748381789079875, 0.7071067811865487940, 0.7070477234798316912 ) ) ;
#1747=CARTESIAN_POINT ( 'NONE',  ( 83.41173289365072208, 75.07748563434969924, 2.765778341857892730 ) ) ;
#1751=EDGE_LOOP ( 'NONE', ( #22660, #6335, #2230, #5340 ) ) ;
#1752=CARTESIAN_POINT ( 'NONE',  ( -88.41758806590422637, 80.31838830481380853, 32.48564084813592956 ) ) ;
#1753=CARTESIAN_POINT ( 'NONE',  ( -75.54218441871489631, 75.03417954463952810, 3.529018660298018695 ) ) ;
#1755=CARTESIAN_POINT ( 'NONE',  ( 90.02055463237803679, 72.00000000000000000, -63.21629334023821656 ) ) ;
#1756=ORIENTED_EDGE ( 'NONE', *, *, #14559, .T. ) ;
#1757=CARTESIAN_POINT ( 'NONE',  ( -93.21002351426726307, 72.00000000000000000, -28.79774562292281104 ) ) ;
#1759=CARTESIAN_POINT ( 'NONE',  ( 104.9011368644396782, 70.01236949047483904, -33.10239539927077601 ) ) ;
#1766=DIRECTION ( 'NONE',  ( 0.01292414190464174703, 0.000000000000000000, 0.9999164797902015955 ) ) ;
#1768=ORIENTED_EDGE ( 'NONE', *, *, #22239, .T. ) ;
#1770=CARTESIAN_POINT ( 'NONE',  ( -90.58204872677625019, 70.40262524007013667, 62.40924858436775935 ) ) ;
#1772=CIRCLE ( 'NONE', #5048, 6.499999999999998224 ) ;
#1777=ORIENTED_EDGE ( 'NONE', *, *, #3040, .T. ) ;
#1781=CARTESIAN_POINT ( 'NONE',  ( 91.97397837737798909, 77.39048292941922114, 29.24031187446957958 ) ) ;
#1783=DIRECTION ( 'NONE',  ( 2.025474946048326158E-22, -1.000000000000000000, 1.876735158486679638E-22 ) ) ;
#1788=CARTESIAN_POINT ( 'NONE',  ( -91.61331032192597945, 77.62808270880877615, -29.62115891282511271 ) ) ;
#1789=AXIS2_PLACEMENT_3D ( 'NONE', #20008, #21607, #6011 ) ;
#1792=CYLINDRICAL_SURFACE ( 'NONE', #22008, 6.499999999999998224 ) ;
#1801=CARTESIAN_POINT ( 'NONE',  ( 2.067862704742617463, 69.99999999999998579, 159.9866367664322979 ) ) ;
#1807=CARTESIAN_POINT ( 'NONE',  ( -38.69757710431294839, 94.02752048664900997, -82.47923521851862461 ) ) ;
#1812=CARTESIAN_POINT ( 'NONE',  ( -90.42246537646651916, 78.26562148642790362, 32.93420195958645280 ) ) ;
#1815=VERTEX_POINT ( 'NONE', #7417 ) ;
#1818=LINE ( 'NONE', #531, #4187 ) ;
#1820=LINE ( 'NONE', #8809, #21334 ) ;
#1823=CARTESIAN_POINT ( 'NONE',  ( -65.91440269377939387, 103.0000000000000000, -70.32555938675406537 ) ) ;
#1847=CARTESIAN_POINT ( 'NONE',  ( -88.16594588878987793, 88.49255433320315944, 52.69555038922003121 ) ) ;
#1851=ORIENTED_EDGE ( 'NONE', *, *, #8400, .T. ) ;
#1853=VECTOR ( 'NONE', #4021, 1000.000000000000114 ) ;
#1854=CARTESIAN_POINT ( 'NONE',  ( -34.23497593041177112, 93.68146586044639434, 83.10373569841586061 ) ) ;
#1855=EDGE_LOOP ( 'NONE', ( #18541, #5060, #3702, #11003 ) ) ;
#1857=CARTESIAN_POINT ( 'NONE',  ( 84.81034445695703994, 75.01375443481772720, -2.741737533029477092 ) ) ;
#1862=EDGE_LOOP ( 'NONE', ( #12568, #13314, #10724, #19997 ) ) ;
#1863=DIRECTION ( 'NONE',  ( 0.01292414190464131335, 1.902755938799530239E-22, 0.9999164797902015955 ) ) ;
#1868=EDGE_LOOP ( 'NONE', ( #6719, #9572, #17708, #474 ) ) ;
#1869=DIRECTION ( 'NONE',  ( -0.9999164797902015955, -2.001050586450178695E-22, 0.01292414190464131335 ) ) ;
#1871=CIRCLE ( 'NONE', #2959, 1.989999999999997105 ) ;
#1883=ORIENTED_EDGE ( 'NONE', *, *, #18342, .T. ) ;
#1888=DIRECTION ( 'NONE',  ( -2.025474946048326158E-22, 1.000000000000000000, -1.876735158486678933E-22 ) ) ;
#1897=CARTESIAN_POINT ( 'NONE',  ( 84.57230515545197136, 105.0000000000000000, 70.33944174062776256 ) ) ;
#1898=CARTESIAN_POINT ( 'NONE',  ( 1.364374644014609697E-14, 69.99999999999998579, -9.836443712999143722E-15 ) ) ;
#1906=CARTESIAN_POINT ( 'NONE',  ( -92.11236706770199589, 79.08401524093159196, -26.36688770261625336 ) ) ;
#1912=CARTESIAN_POINT ( 'NONE',  ( 1.117803423002110774, 45.00000000000000000, 109.6947150755565161 ) ) ;
#1920=EDGE_CURVE ( 'NONE', #12267, #12564, #7508, .T. ) ;
#1922=DIRECTION ( 'NONE',  ( 0.01292414190463830014, 0.000000000000000000, 0.9999164797902017066 ) ) ;
#1933=VECTOR ( 'NONE', #14856, 1000.000000000000000 ) ;
#1938=EDGE_CURVE ( 'NONE', #19786, #13316, #13517, .T. ) ;
#1944=PLANE ( 'NONE',  #2313 ) ;
#1945=PLANE ( 'NONE',  #14360 ) ;
#1946=DIRECTION ( 'NONE',  ( -2.459148776294495979E-24, 1.000000000000000000, -1.902597020224326827E-22 ) ) ;
#1948=EDGE_CURVE ( 'NONE', #20716, #899, #20793, .T. ) ;
#1955=CARTESIAN_POINT ( 'NONE',  ( 106.3959516824313596, 78.65697569891375451, 27.92701496092258040 ) ) ;
#1958=CARTESIAN_POINT ( 'NONE',  ( 39.11273342774209283, 91.99797716581187501, 83.46418088055293083 ) ) ;
#1963=CARTESIAN_POINT ( 'NONE',  ( 85.01653497985981289, 104.3814432989690602, -69.80106575130697877 ) ) ;
#1964=CARTESIAN_POINT ( 'NONE',  ( 36.36981073755603688, 93.68077716319862702, 82.19051635825725555 ) ) ;
#1970=CARTESIAN_POINT ( 'NONE',  ( -88.16914282057626906, 88.71763460176525484, 52.39312110959539837 ) ) ;
#1977=CARTESIAN_POINT ( 'NONE',  ( 80.39208672325557359, 75.13699351169599083, 4.061340467186282943 ) ) ;
#1981=CARTESIAN_POINT ( 'NONE',  ( 91.23296681615025250, 78.26422321607692822, 30.58575029229923459 ) ) ;
#1995=DIRECTION ( 'NONE',  ( -0.9999164797902017066, -2.001050586450178931E-22, 0.01292414190464131508 ) ) ;
#2009=CARTESIAN_POINT ( 'NONE',  ( -64.28883878761490678, 83.29019440189556178, 55.44125366118054643 ) ) ;
#2014=CARTESIAN_POINT ( 'NONE',  ( 91.26841073957255901, 80.27011201451718136, 30.02500290034332053 ) ) ;
#2015=CARTESIAN_POINT ( 'NONE',  ( 89.40819020483024815, 79.89452498912716294, 28.94780723987645388 ) ) ;
#2018=CARTESIAN_POINT ( 'NONE',  ( 64.99457118636311748, 177.0000000000003695, -0.8400692238016915780 ) ) ;
#2020=ORIENTED_EDGE ( 'NONE', *, *, #235, .T. ) ;
#2021=CARTESIAN_POINT ( 'NONE',  ( -92.18978923775263468, 77.29775901949990669, -29.08785173819802594 ) ) ;
#2023=EDGE_LOOP ( 'NONE', ( #2142, #11774, #15367, #15903 ) ) ;
#2029=DIRECTION ( 'NONE',  ( -2.025474946048326158E-22, 1.000000000000000000, -1.876735158486678933E-22 ) ) ;
#2035=CARTESIAN_POINT ( 'NONE',  ( 71.51920288841776596, 92.50622980579329635, 83.57642618781942190 ) ) ;
#2037=CARTESIAN_POINT ( 'NONE',  ( -92.27487665212996149, 79.82259189700857860, 31.19759217298344822 ) ) ;
#2039=CARTESIAN_POINT ( 'NONE',  ( 396.0414077195426898, 177.0000000000003695, -5.118922886994747401 ) ) ;
#2045=VECTOR ( 'NONE', #16778, 1000.000000000000227 ) ;
#2049=DIRECTION ( 'NONE',  ( 0.01292414190464131335, 1.902755938799530239E-22, 0.9999164797902015955 ) ) ;
#2051=FACE_OUTER_BOUND ( 'NONE', #14958, .T. ) ;
#2053=FACE_OUTER_BOUND ( 'NONE', #8199, .T. ) ;
#2055=AXIS2_PLACEMENT_3D ( 'NONE', #10342, #14142, #5029 ) ;
#2062=CARTESIAN_POINT ( 'NONE',  ( 39.42082737383937996, 72.00000000000000000, -83.51645567887783272 ) ) ;
#2071=EDGE_LOOP ( 'NONE', ( #21343, #20643, #4649 ) ) ;
#2073=( BOUNDED_CURVE ( )  B_SPLINE_CURVE ( 3, ( #15853, #13880, #22563, #20867 ),
 .UNSPECIFIED., .F., .T. ) 
 B_SPLINE_CURVE_WITH_KNOTS ( ( 4, 4 ),
 ( 5.433035758877964305, 5.587168164874065646 ),
 .UNSPECIFIED. ) 
 CURVE ( )  GEOMETRIC_REPRESENTATION_ITEM ( )  RATIONAL_B_SPLINE_CURVE ( ( 1.000000000000000000, 0.9980212464270939998, 0.9980212464270939998, 1.000000000000000000 ) ) 
 REPRESENTATION_ITEM ( '' )  );
#2075=ADVANCED_FACE ( 'NONE', ( #17761 ), #10508, .F. ) ;
#2077=ORIENTED_EDGE ( 'NONE', *, *, #16606, .T. ) ;
#2078=DIRECTION ( 'NONE',  ( -0.01292414190464044946, -1.902755938799528593E-22, -0.9999164797902015955 ) ) ;
#2079=CARTESIAN_POINT ( 'NONE',  ( -88.16613847108702373, 88.50822752828271689, 52.67809515463711989 ) ) ;
#2083=EDGE_LOOP ( 'NONE', ( #11750, #18115, #4859, #7474 ) ) ;
#2084=DIRECTION ( 'NONE',  ( 0.01292414190464131508, 0.000000000000000000, 0.9999164797902017066 ) ) ;
#2085=CARTESIAN_POINT ( 'NONE',  ( 88.40906079701872500, 78.43035437438885538, -33.14537955645114664 ) ) ;
#2087=DIRECTION ( 'NONE',  ( -0.9999164797902015955, -2.001050586450180341E-22, 0.01292414190464038874 ) ) ;
#2090=CARTESIAN_POINT ( 'NONE',  ( 92.50752184771765485, 77.20349362929610493, 28.92971669647237576 ) ) ;
#2094=CARTESIAN_POINT ( 'NONE',  ( -75.60071948563958699, 75.03398072390713480, -1.579025930907502318 ) ) ;
#2104=CARTESIAN_POINT ( 'NONE',  ( -41.56623493000981284, 91.17157287525390075, -82.46967996629571473 ) ) ;
#2107=VECTOR ( 'NONE', #22509, 1000.000000000000000 ) ;
#2108=DIRECTION ( 'NONE',  ( 0.9999164797902015955, 2.001050586450177050E-22, -0.01292414190464223796 ) ) ;
#2117=CARTESIAN_POINT ( 'NONE',  ( 91.38403781951994631, 79.16811561863680424, 26.65243986599108794 ) ) ;
#2127=AXIS2_PLACEMENT_3D ( 'NONE', #22218, #2941, #10413 ) ;
#2132=ORIENTED_EDGE ( 'NONE', *, *, #423, .T. ) ;
#2138=CARTESIAN_POINT ( 'NONE',  ( 67.13053572995309537, 70.13637825286164684, -87.14080137989780894 ) ) ;
#2141=CARTESIAN_POINT ( 'NONE',  ( -80.05923150692979107, 54.99999999999999289, -4.065642694558677661 ) ) ;
#2142=ORIENTED_EDGE ( 'NONE', *, *, #6607, .T. ) ;
#2149=ORIENTED_EDGE ( 'NONE', *, *, #18426, .T. ) ;
#2154=DIRECTION ( 'NONE',  ( -2.025474946048326158E-22, 1.000000000000000000, -1.876735158486678933E-22 ) ) ;
#2159=AXIS2_PLACEMENT_3D ( 'NONE', #8263, #9869, #18495 ) ;
#2169=CARTESIAN_POINT ( 'NONE',  ( 4.092765588129412713, 86.14799269895429745, 74.95397050060127242 ) ) ;
#2177=EDGE_CURVE ( 'NONE', #4506, #8789, #15389, .T. ) ;
#2179=EDGE_CURVE ( 'NONE', #15481, #22379, #18418, .T. ) ;
#2187=DIRECTION ( 'NONE',  ( -0.01292414190463827932, 0.000000000000000000, -0.9999164797902018176 ) ) ;
#2193=ORIENTED_EDGE ( 'NONE', *, *, #8950, .F. ) ;
#2196=CARTESIAN_POINT ( 'NONE',  ( -74.89818681777818199, 75.00000638978997358, 0.6335213639023836718 ) ) ;
#2201=FACE_OUTER_BOUND ( 'NONE', #15350, .T. ) ;
#2205=CYLINDRICAL_SURFACE ( 'NONE', #10574, 2.000000000000001776 ) ;
#2210=CARTESIAN_POINT ( 'NONE',  ( -105.1935855565139946, 70.39579207655377502, 32.16088115703475125 ) ) ;
#2211=TOROIDAL_SURFACE ( 'NONE', #5860, 97.00000000000004263, 2.000000000000000000 ) ;
#2222=PLANE ( 'NONE',  #9686 ) ;
#2226=CARTESIAN_POINT ( 'NONE',  ( 83.58290648752347352, 104.4142135623730638, 71.51152175067952044 ) ) ;
#2230=ORIENTED_EDGE ( 'NONE', *, *, #2786, .F. ) ;
#2236=CARTESIAN_POINT ( 'NONE',  ( -93.07689643980960170, 77.12912189501443549, -28.79946631983742833 ) ) ;
#2245=DIRECTION ( 'NONE',  ( 0.01292414190464486780, 0.000000000000000000, 0.9999164797902014845 ) ) ;
#2250=FACE_OUTER_BOUND ( 'NONE', #15518, .T. ) ;
#2251=AXIS2_PLACEMENT_3D ( 'NONE', #18922, #20754, #18816 ) ;
#2257=DIRECTION ( 'NONE',  ( 2.025474946048326158E-22, -1.000000000000000000, 1.876735158486679638E-22 ) ) ;
#2258=EDGE_CURVE ( 'NONE', #20198, #11876, #3388, .T. ) ;
#2259=EDGE_CURVE ( 'NONE', #16639, #14542, #2295, .T. ) ;
#2260=CARTESIAN_POINT ( 'NONE',  ( -90.90343663577488087, 80.03933989046798558, 31.72203358726061495 ) ) ;
#2278=CARTESIAN_POINT ( 'NONE',  ( 83.58290648752347352, 104.4142135623730638, 71.51152175067952044 ) ) ;
#2280=AXIS2_PLACEMENT_3D ( 'NONE', #10183, #2943, #9965 ) ;
#2294=LINE ( 'NONE', #580, #18421 ) ;
#2295=B_SPLINE_CURVE_WITH_KNOTS ( 'NONE', 3,
 ( #21718, #12692, #20000, #21598, #10946, #4039, #21823, #9439, #9566, #9092, #16262, #19660, #16600, #14534, #616, #18199, #14645, #16144, #729, #6004, #5880, #11066, #13137, #4266, #21496, #3927, #18091, #6111, #5760, #11288, #20106, #7725, #2337, #16377, #12918, #19888, #4159, #14763 ),
 .UNSPECIFIED., .F., .F.,
 ( 4, 2, 2, 2, 2, 2, 2, 2, 2, 2, 2, 2, 2, 2, 2, 2, 2, 2, 4 ),
 ( 0.01594779277582532642, 0.01694430233486377002, 0.01794081189390221015, 0.01893732145294065375, 0.01993383101197909388, 0.02093034057101753748, 0.02192685013005597761, 0.02292335968909442120, 0.02391986924813286480, 0.02491637880717130493, 0.02541463358669052500, 0.02591288836620974159, 0.02690939792524816090, 0.02790590748428658369, 0.02890241704332500300, 0.02940067182284419878, 0.02989892660236338762, 0.03089543616140177917, 0.03189194572044016379 ),
 .UNSPECIFIED. ) ;
#2301=VERTEX_POINT ( 'NONE', #13701 ) ;
#2303=CARTESIAN_POINT ( 'NONE',  ( -88.63691684753834465, 88.68770448415855867, 50.34781501682353877 ) ) ;
#2313=AXIS2_PLACEMENT_3D ( 'NONE', #5602, #8936, #450 ) ;
#2314=CARTESIAN_POINT ( 'NONE',  ( -105.8297815006158089, 70.09865364193532855, -30.00121230636252889 ) ) ;
#2319=CARTESIAN_POINT ( 'NONE',  ( 92.63999567227413934, 77.17622496481537553, 28.88303657775549738 ) ) ;
#2325=EDGE_CURVE ( 'NONE', #2805, #1815, #22272, .T. ) ;
#2332=DIRECTION ( 'NONE',  ( 0.000000000000000000, -1.000000000000000000, 0.000000000000000000 ) ) ;
#2333=CARTESIAN_POINT ( 'NONE',  ( -79.92740525950245001, 75.13699351169597662, 6.133505399301365735 ) ) ;
#2337=CARTESIAN_POINT ( 'NONE',  ( -82.16334690560557874, 75.11365078037778176, -3.584353236733231807 ) ) ;
#2339=CARTESIAN_POINT ( 'NONE',  ( -90.16740408589069489, 87.15736368158233915, 51.30261084162481922 ) ) ;
#2340=VERTEX_POINT ( 'NONE', #16922 ) ;
#2344=CARTESIAN_POINT ( 'NONE',  ( -92.11907261954638670, 79.08352528315394636, -26.36518256425475570 ) ) ;
#2349=VECTOR ( 'NONE', #2087, 1000.000000000000114 ) ;
#2355=ORIENTED_EDGE ( 'NONE', *, *, #10784, .T. ) ;
#2364=ORIENTED_EDGE ( 'NONE', *, *, #7835, .F. ) ;
#2367=AXIS2_PLACEMENT_3D ( 'NONE', #9258, #17674, #1922 ) ;
#2371=CARTESIAN_POINT ( 'NONE',  ( 77.79560129287671089, 75.11063986505354251, 3.580215209361726103 ) ) ;
#2372=CARTESIAN_POINT ( 'NONE',  ( -90.10530173132328002, 71.17149643761379707, 62.61299491375256565 ) ) ;
#2379=EDGE_LOOP ( 'NONE', ( #11678, #14418, #11240, #21916 ) ) ;
#2385=CARTESIAN_POINT ( 'NONE',  ( 91.57356387979847057, 79.88289403010834633, -31.31484984389050297 ) ) ;
#2387=CARTESIAN_POINT ( 'NONE',  ( -88.62677304472126139, 79.89796367043616954, 31.25921585370828382 ) ) ;
#2392=ORIENTED_EDGE ( 'NONE', *, *, #22130, .F. ) ;
#2395=ORIENTED_EDGE ( 'NONE', *, *, #11338, .F. ) ;
#2404=LINE ( 'NONE', #9393, #8791 ) ;
#2406=CARTESIAN_POINT ( 'NONE',  ( 81.70668847916368804, 104.4142135623730780, -73.64792636435126383 ) ) ;
#2409=ORIENTED_EDGE ( 'NONE', *, *, #5411, .F. ) ;
#2410=DIRECTION ( 'NONE',  ( 0.01292414190464085018, 1.902755938799529534E-22, 0.9999164797902017066 ) ) ;
#2414=DIRECTION ( 'NONE',  ( 0.01292414190464131335, 1.902755938799530239E-22, 0.9999164797902015955 ) ) ;
#2421=CARTESIAN_POINT ( 'NONE',  ( -89.66172535072847438, 88.16874122514732903, 50.68101772321399778 ) ) ;
#2434=CARTESIAN_POINT ( 'NONE',  ( 91.65137210734579298, 77.59584042966187667, 29.57018005965448637 ) ) ;
#2438=DIRECTION ( 'NONE',  ( -0.9999164797902015955, -2.001050586450176109E-22, 0.01292414190464270113 ) ) ;
#2440=DIRECTION ( 'NONE',  ( -2.459148776293844314E-24, 1.000000000000000000, -1.902597020224326827E-22 ) ) ;
#2445=B_SPLINE_CURVE_WITH_KNOTS ( 'NONE', 3,
 ( #21074, #14320, #5327, #16050, #7280, #21291 ),
 .UNSPECIFIED., .F., .F.,
 ( 4, 2, 4 ),
 ( 0.000000000000000000, 0.0009922935535326105842, 0.001984587107065221168 ),
 .UNSPECIFIED. ) ;
#2448=EDGE_CURVE ( 'NONE', #6510, #14770, #19800, .T. ) ;
#2449=CARTESIAN_POINT ( 'NONE',  ( -90.12718263878197433, 88.36484941033451435, 52.86583380306038293 ) ) ;
#2450=ADVANCED_FACE ( 'NONE', ( #3340 ), #8714, .F. ) ;
#2451=EDGE_LOOP ( 'NONE', ( #6970, #1193, #8517, #6199 ) ) ;
#2454=CARTESIAN_POINT ( 'NONE',  ( -90.39518254297831845, 70.66155102244781006, 61.37085238946110621 ) ) ;
#2459=CARTESIAN_POINT ( 'NONE',  ( 24.46733851482524713, 89.80213272332517249, -79.22137216471709564 ) ) ;
#2460=EDGE_CURVE ( 'NONE', #12053, #5608, #15014, .T. ) ;
#2462=ORIENTED_EDGE ( 'NONE', *, *, #21109, .T. ) ;
#2476=CARTESIAN_POINT ( 'NONE',  ( 75.53224276191924957, 75.03386225069934312, -3.527861427633645075 ) ) ;
#2487=CARTESIAN_POINT ( 'NONE',  ( 92.43457499998881133, 77.12912189496640281, -31.19724316448931134 ) ) ;
#2490=DIRECTION ( 'NONE',  ( 0.9999164797902017066, 0.000000000000000000, -0.01292414190463832269 ) ) ;
#2493=EDGE_CURVE ( 'NONE', #44, #9371, #10596, .T. ) ;
#2500=CARTESIAN_POINT ( 'NONE',  ( -40.65822637310711940, 91.17157287525390075, -84.25167897319539634 ) ) ;
#2509=EDGE_LOOP ( 'NONE', ( #11803, #11301, #10423, #14602 ) ) ;
#2517=CARTESIAN_POINT ( 'NONE',  ( 1.079165849037564184, 69.99999999999998579, 83.49302606248181746 ) ) ;
#2523=ORIENTED_EDGE ( 'NONE', *, *, #6144, .F. ) ;
#2524=AXIS2_PLACEMENT_3D ( 'NONE', #3123, #22606, #2896 ) ;
#2527=CARTESIAN_POINT ( 'NONE',  ( -89.41589774379013988, 89.12196685564443044, 51.54718285326051586 ) ) ;
#2541=CARTESIAN_POINT ( 'NONE',  ( 68.71681667565954399, 91.17157287525390075, -85.89527988174788220 ) ) ;
#2543=FACE_OUTER_BOUND ( 'NONE', #1026, .T. ) ;
#2554=CARTESIAN_POINT ( 'NONE',  ( 1.364373935098378649E-14, 105.0000000000000000, -9.836450281572198869E-15 ) ) ;
#2559=CARTESIAN_POINT ( 'NONE',  ( -105.4170939775132325, 71.46263312473237761, 31.42050039360489677 ) ) ;
#2560=CARTESIAN_POINT ( 'NONE',  ( -90.16191779797397032, 87.20776688749543837, 51.27200115743783471 ) ) ;
#2561=CARTESIAN_POINT ( 'NONE',  ( 41.01898768785991933, 92.04141378167193466, 84.43550307159648582 ) ) ;
#2563=ORIENTED_EDGE ( 'NONE', *, *, #14323, .F. ) ;
#2579=CARTESIAN_POINT ( 'NONE',  ( 91.26258897903525735, 97.45270810253440175, 61.41003422490156538 ) ) ;
#2587=ORIENTED_EDGE ( 'NONE', *, *, #5950, .T. ) ;
#2588=CARTESIAN_POINT ( 'NONE',  ( 105.4334892372614405, 34.61572286322119396, -31.36525700924962834 ) ) ;
#2590=ORIENTED_EDGE ( 'NONE', *, *, #13450, .T. ) ;
#2600=ORIENTED_EDGE ( 'NONE', *, *, #22300, .F. ) ;
#2604=EDGE_CURVE ( 'NONE', #21164, #9279, #14390, .T. ) ;
#2607=DIRECTION ( 'NONE',  ( 2.025474946048326158E-22, -1.000000000000000000, 1.876735158486679638E-22 ) ) ;
#2612=CARTESIAN_POINT ( 'NONE',  ( -110.3452273899772962, 79.04398536104956463, -25.99873445483930823 ) ) ;
#2615=ORIENTED_EDGE ( 'NONE', *, *, #14765, .T. ) ;
#2617=CARTESIAN_POINT ( 'NONE',  ( -66.64819547803482180, 98.52889235517193356, 76.44243005894450960 ) ) ;
#2625=EDGE_CURVE ( 'NONE', #12598, #3397, #14729, .T. ) ;
#2626=CARTESIAN_POINT ( 'NONE',  ( -2.067862704742604141, 72.00000000000000000, -159.9866367664322979 ) ) ;
#2629=AXIS2_PLACEMENT_3D ( 'NONE', #8985, #37, #17512 ) ;
#2632=ORIENTED_EDGE ( 'NONE', *, *, #20291, .F. ) ;
#2635=AXIS2_PLACEMENT_3D ( 'NONE', #10926, #21244, #2084 ) ;
#2636=CARTESIAN_POINT ( 'NONE',  ( -20.87382170032465822, 88.79701099988842827, 78.13772802898489545 ) ) ;
#2639=ADVANCED_FACE ( 'NONE', ( #9302 ), #815, .F. ) ;
#2647=CARTESIAN_POINT ( 'NONE',  ( -88.82223701108780745, 89.02496384438940424, 50.89451478405366203 ) ) ;
#2655=CARTESIAN_POINT ( 'NONE',  ( -36.55288090549052527, 94.02752048664899576, 83.45186405039063970 ) ) ;
#2660=CARTESIAN_POINT ( 'NONE',  ( 88.72067713466825012, 101.8298110126635976, 65.04826529396210333 ) ) ;
#2664=CARTESIAN_POINT ( 'NONE',  ( 39.40254987707580625, 92.58578643762696458, -84.93055112583746791 ) ) ;
#2666=CYLINDRICAL_SURFACE ( 'NONE', #4070, 2.000000000000004885 ) ;
#2667=FACE_OUTER_BOUND ( 'NONE', #9097, .T. ) ;
#2671=AXIS2_PLACEMENT_3D ( 'NONE', #6063, #20058, #4320 ) ;
#2680=ORIENTED_EDGE ( 'NONE', *, *, #16991, .F. ) ;
#2682=CARTESIAN_POINT ( 'NONE',  ( -90.17347746657063112, 87.02151967056039439, 51.38494212375915993 ) ) ;
#2686=EDGE_LOOP ( 'NONE', ( #15685, #2775, #7795, #11862 ) ) ;
#2691=CARTESIAN_POINT ( 'NONE',  ( -91.00106904273528130, 70.29040131071506892, 61.79648398638329354 ) ) ;
#2692=CARTESIAN_POINT ( 'NONE',  ( -88.63197286364696481, 79.89291707602599502, 31.24418567530317503 ) ) ;
#2703=LINE ( 'NONE', #13277, #3699 ) ;
#2706=ORIENTED_EDGE ( 'NONE', *, *, #20034, .T. ) ;
#2709=ORIENTED_EDGE ( 'NONE', *, *, #7404, .F. ) ;
#2713=CARTESIAN_POINT ( 'NONE',  ( 80.05923150692980528, 75.13699351169597662, 4.065642694558706083 ) ) ;
#2716=VECTOR ( 'NONE', #15104, 1000.000000000000000 ) ;
#2722=CARTESIAN_POINT ( 'NONE',  ( 1.717753310876221295, 45.00000000000000000, 109.6869605904137330 ) ) ;
#2723=CARTESIAN_POINT ( 'NONE',  ( 91.47655718793819801, 79.89818662653911474, -31.35069918968699199 ) ) ;
#2732=ORIENTED_EDGE ( 'NONE', *, *, #17846, .F. ) ;
#2738=ADVANCED_FACE ( 'NONE', ( #4673 ), #18378, .F. ) ;
#2753=CARTESIAN_POINT ( 'NONE',  ( -64.33646993259900171, 89.82223348669205620, 51.75612182246453585 ) ) ;
#2754=DIRECTION ( 'NONE',  ( 2.025474946048326158E-22, -1.000000000000000000, 1.876735158486679638E-22 ) ) ;
#2755=ADVANCED_FACE ( 'NONE', ( #2757, #16781 ), #8151, .F. ) ;
#2756=ORIENTED_EDGE ( 'NONE', *, *, #14504, .F. ) ;
#2757=FACE_BOUND ( 'NONE', #2975, .T. ) ;
#2758=CARTESIAN_POINT ( 'NONE',  ( 92.40872671617952960, 72.00000000000000000, -33.19707612406970298 ) ) ;
#2769=DIRECTION ( 'NONE',  ( 0.01292414190464179213, 0.000000000000000000, 0.9999164797902017066 ) ) ;
#2774=CARTESIAN_POINT ( 'NONE',  ( 34.67902741341890760, 93.81357993601811529, -83.23127688097689258 ) ) ;
#2775=ORIENTED_EDGE ( 'NONE', *, *, #22047, .F. ) ;
#2777=CARTESIAN_POINT ( 'NONE',  ( 86.79222083800954124, 104.3814432989690602, 67.58039954014910222 ) ) ;
#2782=CARTESIAN_POINT ( 'NONE',  ( 84.03923162725097029, 104.9999999999999858, -70.97549463945256321 ) ) ;
#2784=ORIENTED_EDGE ( 'NONE', *, *, #18556, .F. ) ;
#2786=EDGE_CURVE ( 'NONE', #22376, #17867, #11350, .T. ) ;
#2791=CARTESIAN_POINT ( 'NONE',  ( -90.12564631705923546, 88.34868647126225483, 52.87392178893500727 ) ) ;
#2800=ORIENTED_EDGE ( 'NONE', *, *, #15005, .F. ) ;
#2801=DIRECTION ( 'NONE',  ( 0.01292414190464044946, 1.902755938799528593E-22, 0.9999164797902015955 ) ) ;
#2805=VERTEX_POINT ( 'NONE', #4793 ) ;
#2809=( BOUNDED_SURFACE ( )  B_SPLINE_SURFACE ( 3, 2, ( 
 ( #6226, #16378, #11402 ),
 ( #9568, #6005, #2682 ),
 ( #1065, #4267, #18414 ),
 ( #11067, #18092, #962 ),
 ( #6113, #11290, #4495 ),
 ( #13138, #7948, #21824 ),
 ( #13255, #5882, #11526 ),
 ( #14979, #13044, #9690 ),
 ( #19889, #20107, #20231 ),
 ( #4374, #7727, #8055 ),
 ( #16714, #4160, #21599 ),
 ( #18529, #5761, #21931 ),
 ( #12792, #21497, #2339 ),
 ( #12919, #2791, #11184 ),
 ( #18200, #2449, #9440 ),
 ( #618, #16481, #20002 ),
 ( #18298, #7609, #2560 ),
 ( #9796, #16601, #852 ),
 ( #16812, #14880, #17371 ),
 ( #15095, #6354, #20565 ),
 ( #3342, #18738, #15323 ),
 ( #22273, #8500, #13703 ),
 ( #20350, #10022, #4940 ),
 ( #1631, #22495, #18957 ),
 ( #5050, #13477, #20451 ),
 ( #4608, #17251, #20794 ),
 ( #4825, #12081, #11740 ),
 ( #1520, #15433, #11863 ),
 ( #22171, #19069, #10362 ),
 ( #8291, #3216, #17142 ),
 ( #22383, #6784, #11633 ),
 ( #18626, #4706, #6566 ),
 ( #22052, #6465, #13582 ),
 ( #18854, #13374, #6676 ),
 ( #10241, #1308, #3117 ),
 ( #16924, #2888, #9902 ),
 ( #1190, #8186, #1410 ),
 ( #15217, #10135, #3001 ),
 ( #17045, #8389, #20687 ),
 ( #11976, #15543, #13809 ),
 ( #5282, #10920, #17941 ),
 ( #9059, #21139, #8960 ),
 ( #1847, #12662, #19301 ),
 ( #2079, #7237, #19531 ),
 ( #16006, #8614, #3797 ),
 ( #10576, #17600, #8843 ),
 ( #15889, #14043, #12424 ),
 ( #8716, #5385, #16112 ),
 ( #10473, #354, #19188 ),
 ( #10693, #10, #7015 ),
 ( #14266, #21028, #3672 ),
 ( #19633, #3565, #14392 ),
 ( #3460, #12536, #12324 ),
 ( #15655, #17722, #3900 ),
 ( #133, #7345, #21241 ),
 ( #13915, #243, #22600 ),
 ( #1970, #7134, #14160 ),
 ( #20907, #19410, #5506 ),
 ( #10822, #15769, #17841 ),
 ( #6893, #17487, #21356 ),
 ( #5628, #5164, #12204 ),
 ( #1738, #16449, #5845 ),
 ( #7470, #13222, #19852 ),
 ( #18379, #9531, #11152 ),
 ( #13109, #14953, #9656 ),
 ( #14845, #2527, #13006 ),
 ( #6083, #4004, #21902 ),
 ( #588, #18270, #4343 ),
 ( #4465, #16566, #12875 ),
 ( #6194, #20079, #19971 ),
 ( #18170, #817, #4237 ),
 ( #20195, #11370, #2421 ),
 ( #11261, #7581, #7813 ),
 ( #21468, #21793, #9410 ),
 ( #21567, #2647, #14613 ),
 ( #18056, #5969, #16682 ),
 ( #931, #4121, #9179 ),
 ( #16232, #471, #2303 ),
 ( #9303, #697, #7691 ),
 ( #14730, #19734, #12762 ) ),
 .UNSPECIFIED., .F., .F., .T. ) 
 B_SPLINE_SURFACE_WITH_KNOTS ( ( 4, 2, 2, 2, 2, 2, 2, 2, 2, 2, 2, 2, 2, 2, 2, 2, 2, 2, 2, 2, 2, 2, 2, 2, 2, 2, 2, 2, 2, 2, 2, 2, 2, 2, 2, 2, 2, 2, 2, 4 ),
 ( 3, 3 ),
 ( 1.949022811632145080E-18, 1.486245462785398132E-07, 2.972490925551306036E-07, 4.458736388317213675E-07, 5.944981851083121843E-07, 7.431227313849028953E-07, 8.917472776614937121E-07, 1.040371823938084529E-06, 1.188996370214675346E-06, 1.337620916491266163E-06, 1.486245462767856768E-06, 1.634870009044447585E-06, 1.783494555321038401E-06, 1.932119101597629430E-06, 2.080743647874220035E-06, 2.229368194150810640E-06, 2.377992740427401669E-06, 2.526617286703992697E-06, 2.675241832980583302E-06, 2.823866379257173908E-06, 2.898178652395469210E-06, 2.972490925533764513E-06, 3.269740018086946146E-06, 3.566989110640127780E-06, 3.864238203193308990E-06, 4.161487295746491047E-06, 4.458736388299673105E-06, 4.755985480852854315E-06, 5.053234573406035525E-06, 5.350483665959217582E-06, 5.647732758512399639E-06, 5.944981851065580850E-06, 6.242230943618762060E-06, 6.539480036171944117E-06, 6.836729128725126174E-06, 7.133978221278307384E-06, 9.511970961703760454E-06, 1.188996370212921352E-05, 1.426795644255466659E-05, 1.902394192340557273E-05 ),
 ( 0.000000000000000000, 1.000000000000000000 ),
 .UNSPECIFIED. ) 
 GEOMETRIC_REPRESENTATION_ITEM ( )  RATIONAL_B_SPLINE_SURFACE ( (
 ( 1.000000000000000000, 0.7071067811865135999, 1.000000000000000000),
 ( 1.000000000000000000, 0.7072381281680633069, 1.000000000000000000),
 ( 1.000000000000000000, 0.7069585476545049429, 1.000000000000000000),
 ( 1.000000000000000000, 0.7074155413819450677, 1.000000000000000000),
 ( 1.000000000000000000, 0.7071390384860228862, 1.000000000000000000),
 ( 1.000000000000000000, 0.7077150574724885290, 1.000000000000000000),
 ( 1.000000000000000000, 0.7074786063547826576, 1.000000000000000000),
 ( 1.000000000000000000, 0.7081708585959944902, 1.000000000000000000),
 ( 1.000000000000000000, 0.7079751951990761460, 1.000000000000000000),
 ( 1.000000000000000000, 0.7087807454553832764, 1.000000000000000000),
 ( 1.000000000000000000, 0.7086266733915456140, 1.000000000000000000),
 ( 1.000000000000000000, 0.7095424613801466496, 1.000000000000000000),
 ( 1.000000000000000000, 0.7094308370090658400, 1.000000000000000000),
 ( 1.000000000000000000, 0.7104536936552536819, 1.000000000000000000),
 ( 1.000000000000000000, 0.7103854132845832670, 1.000000000000000000),
 ( 1.000000000000000000, 0.7115120753684263111, 1.000000000000000000),
 ( 1.000000000000000000, 0.7114880643480506750, 1.000000000000000000),
 ( 1.000000000000000000, 0.7127151874304157309, 1.000000000000000000),
 ( 1.000000000000000000, 0.7127363908997321751, 1.000000000000000000),
 ( 1.000000000000000000, 0.7140605608518137970, 1.000000000000000000),
 ( 1.000000000000000000, 0.7141279362315575696, 1.000000000000000000),
 ( 1.000000000000000000, 0.7155456793979033669, 1.000000000000000000),
 ( 1.000000000000000000, 0.7156601900754941958, 1.000000000000000000),
 ( 1.000000000000000000, 0.7171679822068535159, 1.000000000000000000),
 ( 1.000000000000000000, 0.7173305926685255018, 1.000000000000000000),
 ( 1.000000000000000000, 0.7189248667156663553, 1.000000000000000000),
 ( 1.000000000000000000, 0.7191365387466063241, 1.000000000000000000),
 ( 1.000000000000000000, 0.7208136916140887029, 1.000000000000000000),
 ( 1.000000000000000000, 0.7210753815884107798, 1.000000000000000000),
 ( 1.000000000000000000, 0.7228317799310683966, 1.000000000000000000),
 ( 1.000000000000000000, 0.7231444369243380521, 1.000000000000000000),
 ( 1.000000000000000000, 0.7249764221348216076, 1.000000000000000000),
 ( 1.000000000000000000, 0.7253410135264871661, 1.000000000000000000),
 ( 1.000000000000000000, 0.7272448526125560031, 1.000000000000000000),
 ( 1.000000000000000000, 0.7276627513310924833, 1.000000000000000000),
 ( 1.000000000000000000, 0.7296339184630242780, 1.000000000000000000),
 ( 1.000000000000000000, 0.7301067830575730389, 1.000000000000000000),
 ( 1.000000000000000000, 0.7321408070295029047, 1.000000000000000000),
 ( 1.000000000000000000, 0.7326585513427095187, 1.000000000000000000),
 ( 1.000000000000000000, 0.7342303961178014982, 1.000000000000000000),
 ( 1.000000000000000000, 0.7345026836460134545, 1.000000000000000000),
 ( 1.000000000000000000, 0.7355652195318463926, 1.000000000000000000),
 ( 1.000000000000000000, 0.7359821834485184011, 1.000000000000000000),
 ( 1.000000000000000000, 0.7379952682253708707, 1.000000000000000000),
 ( 1.000000000000000000, 0.7402826106793318761, 1.000000000000000000),
 ( 1.000000000000000000, 0.7437381524183488413, 1.000000000000000000),
 ( 1.000000000000000000, 0.7461303745155040135, 1.000000000000000000),
 ( 1.000000000000000000, 0.7498005034201070673, 1.000000000000000000),
 ( 1.000000000000000000, 0.7522845452621365059, 1.000000000000000000),
 ( 1.000000000000000000, 0.7561493072734657428, 1.000000000000000000),
 ( 1.000000000000000000, 0.7587139551311251617, 1.000000000000000000),
 ( 1.000000000000000000, 0.7627534639691019303, 1.000000000000000000),
 ( 1.000000000000000000, 0.7653892180658008471, 1.000000000000000000),
 ( 1.000000000000000000, 0.7695836597282257330, 1.000000000000000000),
 ( 1.000000000000000000, 0.7722826061538781151, 1.000000000000000000),
 ( 1.000000000000000000, 0.7766122452106001273, 1.000000000000000000),
 ( 1.000000000000000000, 0.7793679326086000447, 1.000000000000000000),
 ( 1.000000000000000000, 0.7838131199424147599, 1.000000000000000000),
 ( 1.000000000000000000, 0.7866200293621847806, 1.000000000000000000),
 ( 1.000000000000000000, 0.7911602176995968794, 1.000000000000000000),
 ( 1.000000000000000000, 0.7939709014748255189, 1.000000000000000000),
 ( 1.000000000000000000, 0.7985820451014939980, 1.000000000000000000),
 ( 1.000000000000000000, 0.8013687969964130575, 1.000000000000000000),
 ( 1.000000000000000000, 0.8060341433133167977, 1.000000000000000000),
 ( 1.000000000000000000, 0.8087928835127498051, 1.000000000000000000),
 ( 1.000000000000000000, 0.8134970145047152323, 1.000000000000000000),
 ( 1.000000000000000000, 0.8162250625491064282, 1.000000000000000000),
 ( 1.000000000000000000, 0.8209521604033785946, 1.000000000000000000),
 ( 1.000000000000000000, 0.8236482853497503198, 1.000000000000000000),
 ( 1.000000000000000000, 0.8283833078820742601, 1.000000000000000000),
 ( 1.000000000000000000, 0.8309614497935257083, 1.000000000000000000),
 ( 1.000000000000000000, 0.8530099714809558087, 1.000000000000000000),
 ( 1.000000000000000000, 0.8723999263078645594, 1.000000000000000000),
 ( 1.000000000000000000, 0.9074054958599828691, 1.000000000000000000),
 ( 1.000000000000000000, 0.9231958273998440712, 1.000000000000000000),
 ( 1.000000000000000000, 0.9505426722021091956, 1.000000000000000000),
 ( 1.000000000000000000, 0.9622396665221361056, 1.000000000000000000),
 ( 1.000000000000000000, 0.9904446952675073357, 1.000000000000000000),
 ( 1.000000000000000000, 1.000033919101930513, 1.000000000000000000),
 ( 1.000000000000000000, 1.000000000000000000, 1.000000000000000000) ) ) 
 REPRESENTATION_ITEM ( '' )  SURFACE ( )  );
#2814=FACE_OUTER_BOUND ( 'NONE', #11527, .T. ) ;
#2816=ADVANCED_FACE ( 'NONE', ( #10210 ), #6577, .F. ) ;
#2819=CARTESIAN_POINT ( 'NONE',  ( 105.5195728421876140, 78.18109283220586292, -31.07451122637847973 ) ) ;
#2827=CARTESIAN_POINT ( 'NONE',  ( 91.90296438722727146, 77.16966923688237046, -31.25747399733695175 ) ) ;
#2828=CARTESIAN_POINT ( 'NONE',  ( 92.21925947168416826, 70.54513337289785113, 59.96440893983636755 ) ) ;
#2836=VERTEX_POINT ( 'NONE', #10327 ) ;
#2838=CARTESIAN_POINT ( 'NONE',  ( -67.52146002153369864, 70.28876377827108968, 86.83823687282564663 ) ) ;
#2841=VECTOR ( 'NONE', #2438, 1000.000000000000114 ) ;
#2847=CARTESIAN_POINT ( 'NONE',  ( -106.2089377515398780, 34.61572286322119396, -28.62973177816246206 ) ) ;
#2853=FACE_BOUND ( 'NONE', #15218, .T. ) ;
#2857=VERTEX_POINT ( 'NONE', #3537 ) ;
#2861=VECTOR ( 'NONE', #13577, 1000.000000000000114 ) ;
#2866=DIRECTION ( 'NONE',  ( 5.257943380984030796E-16, -1.000000000000000000, -6.795817950787834712E-18 ) ) ;
#2867=CARTESIAN_POINT ( 'NONE',  ( -1.421655609510530827, 69.99999999999998579, -109.9908127769221693 ) ) ;
#2868=FACE_OUTER_BOUND ( 'NONE', #7162, .T. ) ;
#2872=EDGE_LOOP ( 'NONE', ( #21707, #2149, #8412 ) ) ;
#2876=CARTESIAN_POINT ( 'NONE',  ( 86.63143169152132828, 104.5954341936825642, 67.78689798060398175 ) ) ;
#2877=CARTESIAN_POINT ( 'NONE',  ( 105.7217631510340965, 70.01235472379877933, 30.37969943364865699 ) ) ;
#2888=CARTESIAN_POINT ( 'NONE',  ( -89.97698801024371562, 88.76047946969235625, 52.44252181446705663 ) ) ;
#2889=CARTESIAN_POINT ( 'NONE',  ( 41.58451242677342918, 92.58578643762696458, 83.88377541325536413 ) ) ;
#2891=ORIENTED_EDGE ( 'NONE', *, *, #10175, .F. ) ;
#2895=CARTESIAN_POINT ( 'NONE',  ( -62.91398989571944611, 99.88146403284555674, 77.93815471138678674 ) ) ;
#2896=DIRECTION ( 'NONE',  ( -0.009138748381789079875, -0.7071067811865487940, -0.7070477234798316912 ) ) ;
#2914=CARTESIAN_POINT ( 'NONE',  ( -64.01352119751047098, 100.1860183968354931, 76.74205626399758273 ) ) ;
#2923=LINE ( 'NONE', #22202, #8150 ) ;
#2930=FACE_OUTER_BOUND ( 'NONE', #20042, .T. ) ;
#2934=CARTESIAN_POINT ( 'NONE',  ( 92.03665420188173130, 70.73625599351603910, 60.24390366714256118 ) ) ;
#2935=EDGE_CURVE ( 'NONE', #14542, #9306, #20648, .T. ) ;
#2938=AXIS2_PLACEMENT_3D ( 'NONE', #2626, #13203, #15166 ) ;
#2941=DIRECTION ( 'NONE',  ( -2.025474946048326158E-22, 1.000000000000000000, -1.876735158486679638E-22 ) ) ;
#2943=DIRECTION ( 'NONE',  ( 2.025474946048326158E-22, -1.000000000000000000, 1.876735158486679638E-22 ) ) ;
#2944=AXIS2_PLACEMENT_3D ( 'NONE', #14138, #17819, #21116 ) ;
#2959=AXIS2_PLACEMENT_3D ( 'NONE', #9201, #11699, #17963 ) ;
#2967=DIRECTION ( 'NONE',  ( 0.01292414190464131335, 0.000000000000000000, 0.9999164797902017066 ) ) ;
#2975=EDGE_LOOP ( 'NONE', ( #4485, #13627 ) ) ;
#2984=ORIENTED_EDGE ( 'NONE', *, *, #11262, .F. ) ;
#2985=CARTESIAN_POINT ( 'NONE',  ( 34.90859880014114935, 93.86605675683669858, -83.28248650840920675 ) ) ;
#2989=CARTESIAN_POINT ( 'NONE',  ( 106.2089377515399065, 72.00000000000000000, 28.62973177816241588 ) ) ;
#2993=AXIS2_PLACEMENT_3D ( 'NONE', #14151, #10570, #1728 ) ;
#2994=ORIENTED_EDGE ( 'NONE', *, *, #12455, .F. ) ;
#3001=CARTESIAN_POINT ( 'NONE',  ( -90.10407258434753430, 87.47042737825177028, 51.11193766723834386 ) ) ;
#3006=CARTESIAN_POINT ( 'NONE',  ( -74.75841872729287729, 95.60624342341641579, 80.69196661707292151 ) ) ;
#3010=DIRECTION ( 'NONE',  ( 0.9999164797902015955, 2.001050586450178695E-22, -0.01292414190464131335 ) ) ;
#3012=CARTESIAN_POINT ( 'NONE',  ( -92.19968689859017275, 79.04398536104956463, 28.61667231988787563 ) ) ;
#3018=CARTESIAN_POINT ( 'NONE',  ( 1.364374644014609697E-14, 69.99999999999998579, -9.836443712999143722E-15 ) ) ;
#3034=CARTESIAN_POINT ( 'NONE',  ( -0.9693106428480922077, 69.99999999999998579, -74.99373598426512899 ) ) ;
#3039=EDGE_CURVE ( 'NONE', #10639, #11300, #2073, .T. ) ;
#3040=EDGE_CURVE ( 'NONE', #495, #6274, #5477, .T. ) ;
#3041=CARTESIAN_POINT ( 'NONE',  ( 105.4334892372614405, 77.12912189496645965, -31.36525700924962834 ) ) ;
#3050=EDGE_CURVE ( 'NONE', #13705, #9861, #5097, .T. ) ;
#3060=AXIS2_PLACEMENT_3D ( 'NONE', #3257, #9946, #9831 ) ;
#3061=EDGE_CURVE ( 'NONE', #13946, #3588, #8681, .T. ) ;
#3065=AXIS2_PLACEMENT_3D ( 'NONE', #6930, #3841, #7054 ) ;
#3067=CARTESIAN_POINT ( 'NONE',  ( -68.01573619543681559, 70.58429683895616336, 86.45204278734176739 ) ) ;
#3078=ORIENTED_EDGE ( 'NONE', *, *, #5726, .F. ) ;
#3080=VECTOR ( 'NONE', #1739, 1000.000000000000000 ) ;
#3082=CARTESIAN_POINT ( 'NONE',  ( 86.02081024124220221, 103.0873963570200118, -68.57787521732684866 ) ) ;
#3088=LINE ( 'NONE', #13551, #19969 ) ;
#3098=CARTESIAN_POINT ( 'NONE',  ( 92.40872671617952960, 34.61572286322119396, -33.19707612406970298 ) ) ;
#3100=CARTESIAN_POINT ( 'NONE',  ( -89.76989948563728205, 88.05754991457587266, 50.75033462167537834 ) ) ;
#3101=ORIENTED_EDGE ( 'NONE', *, *, #20324, .F. ) ;
#3102=CARTESIAN_POINT ( 'NONE',  ( 0.000000000000000000, 0.000000000000000000, 0.000000000000000000 ) ) ;
#3103=CARTESIAN_POINT ( 'NONE',  ( -91.21019055468684655, 72.00000000000000000, -28.82359390673209631 ) ) ;
#3107=ORIENTED_EDGE ( 'NONE', *, *, #9033, .F. ) ;
#3110=ORIENTED_EDGE ( 'NONE', *, *, #12999, .T. ) ;
#3116=DIRECTION ( 'NONE',  ( -0.009985269297354625040, -0.6348858185549794975, -0.7725414498878574454 ) ) ;
#3117=CARTESIAN_POINT ( 'NONE',  ( -90.11629072746302427, 87.42992512273923467, 51.13668368328682590 ) ) ;
#3120=VERTEX_POINT ( 'NONE', #14725 ) ;
#3122=CARTESIAN_POINT ( 'NONE',  ( -34.90911429189236515, 93.86615990965727008, 83.28258796055321511 ) ) ;
#3123=CARTESIAN_POINT ( 'NONE',  ( 394.6585245357460963, 69.99999999999997158, -112.1099862245463896 ) ) ;
#3124=EDGE_LOOP ( 'NONE', ( #3780, #13835, #15612, #7870 ) ) ;
#3133=DIRECTION ( 'NONE',  ( 0.01292414190464131335, 1.902755938799530239E-22, 0.9999164797902015955 ) ) ;
#3134=CARTESIAN_POINT ( 'NONE',  ( -70.88807251563926570, 91.17157287525390075, -82.09068872300603914 ) ) ;
#3136=CARTESIAN_POINT ( 'NONE',  ( -38.46706438352712354, 72.00000000000000000, 85.27439087629284131 ) ) ;
#3144=ORIENTED_EDGE ( 'NONE', *, *, #4857, .F. ) ;
#3146=CARTESIAN_POINT ( 'NONE',  ( -88.05170339851980543, 72.97786998644572520, 61.56719313945617245 ) ) ;
#3147=VECTOR ( 'NONE', #4925, 1000.000000000000000 ) ;
#3156=CARTESIAN_POINT ( 'NONE',  ( 90.41053243085600855, 78.34173690304720594, -33.04444670410838825 ) ) ;
#3160=ORIENTED_EDGE ( 'NONE', *, *, #8301, .F. ) ;
#3162=EDGE_CURVE ( 'NONE', #17867, #12773, #9174, .T. ) ;
#3165=CARTESIAN_POINT ( 'NONE',  ( -67.13053572995303853, 70.13637825286163263, 87.14080137989778052 ) ) ;
#3167=CARTESIAN_POINT ( 'NONE',  ( 70.90635001240286783, 92.58578643762697880, 83.50478416996566011 ) ) ;
#3171=CARTESIAN_POINT ( 'NONE',  ( -39.40254987707573520, 92.58578643762697880, 84.93055112583743949 ) ) ;
#3184=EDGE_CURVE ( 'NONE', #22618, #21849, #21353, .T. ) ;
#3189=ORIENTED_EDGE ( 'NONE', *, *, #18250, .F. ) ;
#3197=ORIENTED_EDGE ( 'NONE', *, *, #16325, .T. ) ;
#3199=CARTESIAN_POINT ( 'NONE',  ( -88.71179014270776975, 88.67509488062695766, 50.35684176716525684 ) ) ;
#3203=FACE_OUTER_BOUND ( 'NONE', #2686, .T. ) ;
#3215=CARTESIAN_POINT ( 'NONE',  ( 91.02819465875460025, 70.25795030837511490, -61.75749006523108164 ) ) ;
#3216=CARTESIAN_POINT ( 'NONE',  ( -90.02893273579236677, 88.66443490277293904, 52.56386379439879875 ) ) ;
#3220=CARTESIAN_POINT ( 'NONE',  ( -75.17435380461473926, 95.13881385111719169, 80.30459320758008346 ) ) ;
#3238=AXIS2_PLACEMENT_3D ( 'NONE', #10361, #17370, #21138 ) ;
#3244=CARTESIAN_POINT ( 'NONE',  ( -90.04240250630805065, 70.00863645477431874, 63.19825073092409440 ) ) ;
#3249=CARTESIAN_POINT ( 'NONE',  ( -90.16402721638407058, 71.32383232314188604, 60.62233968236869686 ) ) ;
#3257=CARTESIAN_POINT ( 'NONE',  ( 91.62437796271727564, 34.61572286322119396, 60.86849236629024773 ) ) ;
#3261=CARTESIAN_POINT ( 'NONE',  ( 79.99331838321614896, 55.00000000000000000, -1.033931352371314949 ) ) ;
#3264=DIRECTION ( 'NONE',  ( 0.01292414190464131335, 1.902755938799530239E-22, 0.9999164797902015955 ) ) ;
#3265=DIRECTION ( 'NONE',  ( -2.025474946048326158E-22, 1.000000000000000000, -1.876735158486679638E-22 ) ) ;
#3266=AXIS2_PLACEMENT_3D ( 'NONE', #930, #22242, #11707 ) ;
#3268=CARTESIAN_POINT ( 'NONE',  ( -91.26841073957253059, 80.27011201452100408, -30.02500290034050323 ) ) ;
#3269=ORIENTED_EDGE ( 'NONE', *, *, #6493, .F. ) ;
#3270=CARTESIAN_POINT ( 'NONE',  ( -70.91392079944854743, 91.17157287525390075, -84.09052168258642723 ) ) ;
#3275=( GEOMETRIC_REPRESENTATION_CONTEXT ( 3 ) GLOBAL_UNCERTAINTY_ASSIGNED_CONTEXT ( ( #20316 ) ) GLOBAL_UNIT_ASSIGNED_CONTEXT ( ( #12330, #3354, #22394 ) ) REPRESENTATION_CONTEXT ( 'NONE', 'WORKASPACE' ) );
#3282=DIRECTION ( 'NONE',  ( 0.9999164797902017066, 2.001050586450178931E-22, -0.01292414190464131508 ) ) ;
#3286=CARTESIAN_POINT ( 'NONE',  ( 108.7507233931858082, 76.71731347669783929, 17.16766896971239120 ) ) ;
#3291=ORIENTED_EDGE ( 'NONE', *, *, #17774, .T. ) ;
#3300=CARTESIAN_POINT ( 'NONE',  ( -88.40906079701869658, 78.43035437438882695, 33.14537955645111822 ) ) ;
#3304=EDGE_CURVE ( 'NONE', #44, #19786, #15293, .T. ) ;
#3315=EDGE_CURVE ( 'NONE', #13764, #19083, #1100, .T. ) ;
#3324=( LENGTH_UNIT ( ) NAMED_UNIT ( * ) SI_UNIT ( .MILLI., .METRE. ) );
#3328=CARTESIAN_POINT ( 'NONE',  ( 35.95309506732430549, 93.50464841319750064, 82.03286182426640494 ) ) ;
#3335=ORIENTED_EDGE ( 'NONE', *, *, #10260, .T. ) ;
#3339=B_SPLINE_CURVE_WITH_KNOTS ( 'NONE', 3,
 ( #18520, #2782, #10463, #10352, #7124, #1963 ),
 .UNSPECIFIED., .F., .F.,
 ( 4, 2, 4 ),
 ( 0.000000000000000000, 0.0009977625019781909133, 0.001995525003956381827 ),
 .UNSPECIFIED. ) ;
#3340=FACE_OUTER_BOUND ( 'NONE', #8742, .T. ) ;
#3342=CARTESIAN_POINT ( 'NONE',  ( -88.16361364164851011, 88.27739129944409058, 52.90104011961382469 ) ) ;
#3351=CARTESIAN_POINT ( 'NONE',  ( -36.07200259421443889, 94.02752048664967788, 83.44564859173975435 ) ) ;
#3354=( NAMED_UNIT ( * ) PLANE_ANGLE_UNIT ( ) SI_UNIT ( $, .RADIAN. ) );
#3367=CARTESIAN_POINT ( 'NONE',  ( 105.0923722050658711, 70.19488773545521099, -32.49013605942705851 ) ) ;
#3369=CARTESIAN_POINT ( 'NONE',  ( -63.99768274785666478, 99.80253851968858214, 77.96744723695394441 ) ) ;
#3372=ORIENTED_EDGE ( 'NONE', *, *, #16567, .F. ) ;
#3375=ADVANCED_FACE ( 'NONE', ( #5128 ), #19379, .F. ) ;
#3380=CARTESIAN_POINT ( 'NONE',  ( -90.03465221005033925, 70.01281497139055432, 63.19621350536183968 ) ) ;
#3387=DIRECTION ( 'NONE',  ( 0.01292414190464131335, 1.902755938799530239E-22, 0.9999164797902015955 ) ) ;
#3388=B_SPLINE_CURVE_WITH_KNOTS ( 'NONE', 3,
 ( #8565, #6842, #20849, #5106, #19765, #7506, #12790, #2210, #14423, #7849, #851, #503, #9336, #2559, #21386, #14879 ),
 .UNSPECIFIED., .F., .F.,
 ( 4, 2, 2, 2, 2, 2, 2, 4 ),
 ( 0.000000000000000000, 0.0003989366781685712302, 0.0007978733563371424604, 0.001196810034505713582, 0.001595746712674284921, 0.001994683390842856476, 0.002393620069011427164, 0.003191493425348539484 ),
 .UNSPECIFIED. ) ;
#3390=CARTESIAN_POINT ( 'NONE',  ( 90.41742102548467130, 80.31838830481380853, -32.51148913194525392 ) ) ;
#3391=ORIENTED_EDGE ( 'NONE', *, *, #20902, .T. ) ;
#3397=VERTEX_POINT ( 'NONE', #15856 ) ;
#3398=CARTESIAN_POINT ( 'NONE',  ( -91.28977804672278751, 78.08428866167092508, -30.31923231637458471 ) ) ;
#3412=CARTESIAN_POINT ( 'NONE',  ( -89.66113247980429435, 100.6041916471018709, -63.72504470331098503 ) ) ;
#3414=DIRECTION ( 'NONE',  ( 0.9999164797902015955, 2.001050586450178695E-22, -0.01292414190464131335 ) ) ;
#3417=CARTESIAN_POINT ( 'NONE',  ( 85.01653497985981289, 104.3814432989690602, -69.80106575130697877 ) ) ;
#3419=CARTESIAN_POINT ( 'NONE',  ( -72.51438462527775641, 87.23323244114081376, 69.92599951943640235 ) ) ;
#3420=DIRECTION ( 'NONE',  ( -0.9999164797902017066, 1.387778780781447253E-14, 0.01292414190463832269 ) ) ;
#3427=LINE ( 'NONE', #12291, #3440 ) ;
#3428=ORIENTED_EDGE ( 'NONE', *, *, #6225, .T. ) ;
#3440=VECTOR ( 'NONE', #22463, 1000.000000000000000 ) ;
#3442=EDGE_CURVE ( 'NONE', #17368, #4929, #12632, .T. ) ;
#3446=CARTESIAN_POINT ( 'NONE',  ( 106.7989984338461653, 79.11557862755608994, 26.34385626240403511 ) ) ;
#3455=VERTEX_POINT ( 'NONE', #14698 ) ;
#3460=CARTESIAN_POINT ( 'NONE',  ( -88.16819192123389826, 88.65820917459086559, 52.48530130829333729 ) ) ;
#3461=EDGE_CURVE ( 'NONE', #15089, #19786, #21253, .T. ) ;
#3463=ORIENTED_EDGE ( 'NONE', *, *, #3461, .F. ) ;
#3464=VERTEX_POINT ( 'NONE', #18028 ) ;
#3466=CYLINDRICAL_SURFACE ( 'NONE', #18780, 2.000000000000001332 ) ;
#3470=CARTESIAN_POINT ( 'NONE',  ( 84.44445234771735898, 75.03417954463949968, 1.461155955555357044 ) ) ;
#3476=DIRECTION ( 'NONE',  ( 0.9999164797902017066, 2.001050586450178931E-22, -0.01292414190464131508 ) ) ;
#3479=CARTESIAN_POINT ( 'NONE',  ( -106.0833544754548114, 79.13355406794943292, 29.09322962842180615 ) ) ;
#3480=EDGE_CURVE ( 'NONE', #5690, #12459, #4380, .T. ) ;
#3481=VERTEX_POINT ( 'NONE', #668 ) ;
#3482=CARTESIAN_POINT ( 'NONE',  ( -110.8786557059970477, 104.3814432989690602, -67.26907703621752432 ) ) ;
#3494=DIRECTION ( 'NONE',  ( 0.01292414190464131508, 0.000000000000000000, 0.9999164797902017066 ) ) ;
#3498=CIRCLE ( 'NONE', #8987, 112.5000000000000284 ) ;
#3501=CARTESIAN_POINT ( 'NONE',  ( 91.23438425464441082, 78.34087653192547407, 30.69541483481418709 ) ) ;
#3502=CARTESIAN_POINT ( 'NONE',  ( 91.86780221137911440, 79.10677575599459033, 26.44518439498796880 ) ) ;
#3507=ORIENTED_EDGE ( 'NONE', *, *, #11084, .T. ) ;
#3508=CARTESIAN_POINT ( 'NONE',  ( -90.50635355031123197, 79.35163122866377705, -27.25632624756008937 ) ) ;
#3523=CARTESIAN_POINT ( 'NONE',  ( 70.91392079944854743, 91.17157287525388654, 84.09052168258639881 ) ) ;
#3537=CARTESIAN_POINT ( 'NONE',  ( 87.98413419613014241, 100.6041916471018851, -66.02114910964037620 ) ) ;
#3544=CIRCLE ( 'NONE', #6124, 1.999999999999997335 ) ;
#3550=EDGE_LOOP ( 'NONE', ( #12061, #4150, #15674, #19616 ) ) ;
#3555=DIRECTION ( 'NONE',  ( -0.01292414190463992904, -1.902755938799528123E-22, -0.9999164797902017066 ) ) ;
#3558=ORIENTED_EDGE ( 'NONE', *, *, #12537, .F. ) ;
#3564=EDGE_CURVE ( 'NONE', #9861, #17867, #21980, .T. ) ;
#3565=CARTESIAN_POINT ( 'NONE',  ( -89.73902452844515665, 89.01173883974765033, 52.00261209584472510 ) ) ;
#3568=VERTEX_POINT ( 'NONE', #2500 ) ;
#3573=CARTESIAN_POINT ( 'NONE',  ( -104.8202145123291018, 69.99999999999998579, 33.35749735200943178 ) ) ;
#3578=CARTESIAN_POINT ( 'NONE',  ( -77.82735487582385758, 75.11374352463818127, 5.654166264129496078 ) ) ;
#3579=B_SPLINE_CURVE_WITH_KNOTS ( 'NONE', 3,
 ( #6238, #15331, #9805, #8397, #2692, #20461, #4618, #6574, #22181, #9698, #18862, #13593, #11536, #15443, #1076, #22060, #3012, #20576 ),
 .UNSPECIFIED., .F., .F.,
 ( 4, 2, 2, 2, 2, 2, 2, 2, 4 ),
 ( 0.000000000000000000, 0.0007972436847030672444, 0.001594487369406134489, 0.002391731054109201733, 0.003188974738812268978, 0.003986218423515336222, 0.004783462108218403466, 0.005580705792921470711, 0.006377949477624537955 ),
 .UNSPECIFIED. ) ;
#3583=EDGE_CURVE ( 'NONE', #7781, #17835, #10471, .T. ) ;
#3585=CARTESIAN_POINT ( 'NONE',  ( -38.69757710431294839, 94.02752048664900997, -82.47923521851862461 ) ) ;
#3586=CARTESIAN_POINT ( 'NONE',  ( 89.23620587891578282, 78.43035437438882695, 30.84927515012174482 ) ) ;
#3587=CARTESIAN_POINT ( 'NONE',  ( 105.2816027134186498, 70.66149885336976411, -31.87151722101071272 ) ) ;
#3588=VERTEX_POINT ( 'NONE', #16655 ) ;
#3590=EDGE_LOOP ( 'NONE', ( #17791, #3335, #7224, #12989 ) ) ;
#3601=PLANE ( 'NONE',  #6733 ) ;
#3605=CARTESIAN_POINT ( 'NONE',  ( 91.69412133380886587, 80.03889463955920291, 29.36066737363380241 ) ) ;
#3606=ADVANCED_FACE ( 'NONE', ( #613 ), #2205, .T. ) ;
#3609=CARTESIAN_POINT ( 'NONE',  ( 89.99332827845005056, 79.52815953299851515, 27.82019389467122750 ) ) ;
#3614=CARTESIAN_POINT ( 'NONE',  ( -92.94153934368371495, 77.13727434530990479, -28.81475843614325782 ) ) ;
#3616=ORIENTED_EDGE ( 'NONE', *, *, #22300, .T. ) ;
#3619=CARTESIAN_POINT ( 'NONE',  ( -70.22615711568091967, 70.59893530615325119, -84.66585046671893622 ) ) ;
#3624=ORIENTED_EDGE ( 'NONE', *, *, #7185, .T. ) ;
#3625=CARTESIAN_POINT ( 'NONE',  ( 1.364374644014609697E-14, 69.99999999999998579, -9.836443712999143722E-15 ) ) ;
#3626=ORIENTED_EDGE ( 'NONE', *, *, #18645, .F. ) ;
#3638=DIRECTION ( 'NONE',  ( -0.01292414190464131508, -1.902755938799530474E-22, -0.9999164797902017066 ) ) ;
#3649=DIRECTION ( 'NONE',  ( -0.01292414190464131335, -1.902755938799530239E-22, -0.9999164797902015955 ) ) ;
#3650=AXIS2_PLACEMENT_3D ( 'NONE', #17809, #10436, #17913 ) ;
#3651=ORIENTED_EDGE ( 'NONE', *, *, #18976, .F. ) ;
#3663=VECTOR ( 'NONE', #3414, 1000.000000000000114 ) ;
#3665=ORIENTED_EDGE ( 'NONE', *, *, #4286, .T. ) ;
#3671=DIRECTION ( 'NONE',  ( 0.7968670734554454960, -0.4220031449644340849, -0.4323380770677970331 ) ) ;
#3672=CARTESIAN_POINT ( 'NONE',  ( -90.02167563947240581, 87.67692088304698927, 50.98541494077212377 ) ) ;
#3673=ORIENTED_EDGE ( 'NONE', *, *, #10099, .T. ) ;
#3678=VECTOR ( 'NONE', #22146, 1000.000000000000000 ) ;
#3681=CARTESIAN_POINT ( 'NONE',  ( 82.60421184180059129, 75.10273324658503213, 3.350270875632189505 ) ) ;
#3683=ORIENTED_EDGE ( 'NONE', *, *, #16815, .F. ) ;
#3687=DIRECTION ( 'NONE',  ( -0.9999164797902015955, -4.653667080246434899E-16, 0.01292414190464084844 ) ) ;
#3692=CARTESIAN_POINT ( 'NONE',  ( -105.6047345086702336, 78.54962563481552706, 30.78394349069507996 ) ) ;
#3694=CARTESIAN_POINT ( 'NONE',  ( 91.62437796271728985, 71.80839515725416788, 60.86849236629024062 ) ) ;
#3697=ORIENTED_EDGE ( 'NONE', *, *, #21017, .F. ) ;
#3699=VECTOR ( 'NONE', #875, 1000.000000000000000 ) ;
#3701=LINE ( 'NONE', #10722, #17684 ) ;
#3702=ORIENTED_EDGE ( 'NONE', *, *, #9562, .F. ) ;
#3711=CARTESIAN_POINT ( 'NONE',  ( -88.74294073166163344, 70.70905333810220839, 62.85632276041776123 ) ) ;
#3713=CARTESIAN_POINT ( 'NONE',  ( 395.1215762121263992, 103.0000000000000000, -76.28455149755049547 ) ) ;
#3717=ORIENTED_EDGE ( 'NONE', *, *, #8400, .F. ) ;
#3722=CARTESIAN_POINT ( 'NONE',  ( 92.67786813602299389, 77.16999450923081838, 28.87226322141187040 ) ) ;
#3727=B_SPLINE_CURVE_WITH_KNOTS ( 'NONE', 3,
 ( #8680, #3082, #20866, #94 ),
 .UNSPECIFIED., .F., .F.,
 ( 4, 4 ),
 ( 0.0009630630797684288464, 0.007033511846324326695 ),
 .UNSPECIFIED. ) ;
#3728=EDGE_CURVE ( 'NONE', #19631, #5033, #9561, .T. ) ;
#3733=CARTESIAN_POINT ( 'NONE',  ( -89.40485731804325553, 79.89806915697583634, -28.95844815008361905 ) ) ;
#3740=DIRECTION ( 'NONE',  ( -0.01292414190464131335, -1.902755938799530239E-22, -0.9999164797902015955 ) ) ;
#3752=AXIS2_PLACEMENT_3D ( 'NONE', #8932, #12492, #7213 ) ;
#3754=EDGE_CURVE ( 'NONE', #19631, #4929, #17172, .T. ) ;
#3757=CARTESIAN_POINT ( 'NONE',  ( -88.55041925572842842, 79.97987315375630146, 31.50236046386196165 ) ) ;
#3767=DIRECTION ( 'NONE',  ( -2.025474946048326393E-22, 1.000000000000000000, -1.876735158486679873E-22 ) ) ;
#3777=ORIENTED_EDGE ( 'NONE', *, *, #14978, .T. ) ;
#3780=ORIENTED_EDGE ( 'NONE', *, *, #17199, .T. ) ;
#3787=CARTESIAN_POINT ( 'NONE',  ( 88.82263333796723259, 169.9999999999999716, -1.148052203164690033 ) ) ;
#3792=CARTESIAN_POINT ( 'NONE',  ( 37.74318974735589904, 93.98903733564172569, 82.45639132626887147 ) ) ;
#3795=AXIS2_PLACEMENT_3D ( 'NONE', #226, #9614, #22431 ) ;
#3797=CARTESIAN_POINT ( 'NONE',  ( -90.07961787348274640, 87.54157812894763424, 51.06841591324713647 ) ) ;
#3799=B_SPLINE_CURVE_WITH_KNOTS ( 'NONE', 3,
 ( #6965, #5005, #15388, #10311, #12034, #20404, #15613, #6522, #6850, #19023, #13539, #3286, #13872, #11823 ),
 .UNSPECIFIED., .F., .F.,
 ( 4, 2, 2, 2, 2, 2, 4 ),
 ( 0.05403846203490970945, 0.06102746434071360665, 0.06801646664651750385, 0.08199447125812529824, 0.08898347356392918850, 0.09597247586973307876, 0.1099504804813408732 ),
 .UNSPECIFIED. ) ;
#3805=FACE_OUTER_BOUND ( 'NONE', #17227, .T. ) ;
#3806=ORIENTED_EDGE ( 'NONE', *, *, #15296, .F. ) ;
#3812=CYLINDRICAL_SURFACE ( 'NONE', #21633, 2.000000000000004885 ) ;
#3815=CARTESIAN_POINT ( 'NONE',  ( -75.31779428286061773, 75.02317907734844482, 3.077797884313373977 ) ) ;
#3819=ORIENTED_EDGE ( 'NONE', *, *, #16193, .F. ) ;
#3820=EDGE_CURVE ( 'NONE', #12, #3588, #6460, .T. ) ;
#3821=CARTESIAN_POINT ( 'NONE',  ( -73.00030478232707765, 95.66452290628956234, 82.28581592040848136 ) ) ;
#3823=AXIS2_PLACEMENT_3D ( 'NONE', #13459, #3282, #15074 ) ;
#3833=AXIS2_PLACEMENT_3D ( 'NONE', #14116, #20862, #17680 ) ;
#3838=CARTESIAN_POINT ( 'NONE',  ( -91.70242328196546566, 70.02268785600074352, 60.75168657352403301 ) ) ;
#3839=AXIS2_PLACEMENT_3D ( 'NONE', #2722, #6603, #10070 ) ;
#3840=CARTESIAN_POINT ( 'NONE',  ( 1.364374644014609697E-14, 69.99999999999998579, -9.836443712999143722E-15 ) ) ;
#3841=DIRECTION ( 'NONE',  ( -2.025474946048326158E-22, 1.000000000000000000, -1.876735158486679638E-22 ) ) ;
#3859=ORIENTED_EDGE ( 'NONE', *, *, #8501, .T. ) ;
#3867=CARTESIAN_POINT ( 'NONE',  ( -91.28310237474858013, 79.93543901797764306, 31.44354501024113446 ) ) ;
#3868=CARTESIAN_POINT ( 'NONE',  ( 1.247179693797900502, 69.99999999999998579, 96.49194029975444664 ) ) ;
#3874=CARTESIAN_POINT ( 'NONE',  ( 92.82229925712805141, 72.00000000000000000, -1.199748770783255924 ) ) ;
#3879=PLANE ( 'NONE',  #17324 ) ;
#3883=EDGE_CURVE ( 'NONE', #5147, #14492, #21904, .T. ) ;
#3886=ORIENTED_EDGE ( 'NONE', *, *, #12455, .T. ) ;
#3894=CARTESIAN_POINT ( 'NONE',  ( -5.193835686285779296, 86.33565059398134167, 75.28338189912726364 ) ) ;
#3895=EDGE_CURVE ( 'NONE', #9274, #18312, #1772, .T. ) ;
#3900=CARTESIAN_POINT ( 'NONE',  ( -89.98474239258742102, 87.74831365670060279, 50.94151585748681299 ) ) ;
#3904=EDGE_CURVE ( 'NONE', #13498, #10132, #10180, .T. ) ;
#3912=DIRECTION ( 'NONE',  ( -0.01292414190464131508, 0.000000000000000000, -0.9999164797902017066 ) ) ;
#3915=CARTESIAN_POINT ( 'NONE',  ( -92.91906646248267521, 77.13883058002311088, -28.81763569833110239 ) ) ;
#3916=CARTESIAN_POINT ( 'NONE',  ( -74.93482218714731857, 75.00176059250013338, 0.3029847661794342062 ) ) ;
#3927=CARTESIAN_POINT ( 'NONE',  ( -84.09223301484821889, 75.05036917497851334, -2.018900408767783983 ) ) ;
#3931=CARTESIAN_POINT ( 'NONE',  ( 93.23587179807657321, 72.00000000000000000, 30.79757858250317071 ) ) ;
#3932=EDGE_CURVE ( 'NONE', #10181, #14619, #17188, .T. ) ;
#3941=CARTESIAN_POINT ( 'NONE',  ( 91.47552206421229926, 77.76803451549852753, 29.83954006679655535 ) ) ;
#3942=DIRECTION ( 'NONE',  ( 2.025474946048326158E-22, -1.000000000000000000, 1.876735158486679638E-22 ) ) ;
#3947=CARTESIAN_POINT ( 'NONE',  ( -90.70439626174763248, 79.29995750804913257, -27.08818539008188964 ) ) ;
#3949=VECTOR ( 'NONE', #5099, 1000.000000000000114 ) ;
#3963=CARTESIAN_POINT ( 'NONE',  ( -91.57356387979842793, 79.88289403011208378, 31.31484984389048876 ) ) ;
#3968=ORIENTED_EDGE ( 'NONE', *, *, #2935, .T. ) ;
#3974=CARTESIAN_POINT ( 'NONE',  ( 39.42082737383937996, 72.00000000000000000, -83.51645567887783272 ) ) ;
#3976=ADVANCED_FACE ( 'NONE', ( #6730 ), #9095, .T. ) ;
#3986=EDGE_LOOP ( 'NONE', ( #2523, #7255, #6886, #20344, #9961, #387, #15871, #9783, #1127, #16837, #6587, #7019, #22448, #19886, #11056, #14840, #15036, #16890, #18983, #21776, #10606, #17366, #8330, #18255, #14892, #13139, #7663, #4579, #2706, #13194, #16010, #2732, #10375, #5309, #14590, #13641 ) ) ;
#3993=ADVANCED_FACE ( 'NONE', ( #529 ), #9240, .F. ) ;
#4003=DIRECTION ( 'NONE',  ( -2.025474946048326158E-22, 1.000000000000000000, -1.876735158486679638E-22 ) ) ;
#4004=CARTESIAN_POINT ( 'NONE',  ( -89.40021307249486426, 89.12052993720315897, 51.52924698431865380 ) ) ;
#4015=CARTESIAN_POINT ( 'NONE',  ( -105.9930786687657189, 70.38870405239201489, -29.41946405304836887 ) ) ;
#4021=DIRECTION ( 'NONE',  ( 0.9999164797902015955, 2.001050586450178695E-22, -0.01292414190464131335 ) ) ;
#4028=CARTESIAN_POINT ( 'NONE',  ( -37.51330139321489554, 72.00000000000000000, 87.03232607370787832 ) ) ;
#4034=EDGE_LOOP ( 'NONE', ( #12480, #18041, #19764, #20158 ) ) ;
#4036=ORIENTED_EDGE ( 'NONE', *, *, #10468, .T. ) ;
#4039=CARTESIAN_POINT ( 'NONE',  ( -82.19103547355555861, 75.11063986505352830, 5.648077914104375985 ) ) ;
#4041=FACE_OUTER_BOUND ( 'NONE', #14264, .T. ) ;
#4046=VECTOR ( 'NONE', #5440, 1000.000000000000114 ) ;
#4050=CARTESIAN_POINT ( 'NONE',  ( 70.71197882986199090, 71.18508886668922742, 84.26048200481866957 ) ) ;
#4055=AXIS2_PLACEMENT_3D ( 'NONE', #6914, #17746, #19651 ) ;
#4058=CARTESIAN_POINT ( 'NONE',  ( 91.59502366432090525, 95.97275144416938986, 60.91270374391774567 ) ) ;
#4060=ADVANCED_FACE ( 'NONE', ( #7869 ), #21620, .F. ) ;
#4066=DIRECTION ( 'NONE',  ( -0.01292414190464023262, 0.000000000000000000, -0.9999164797902017066 ) ) ;
#4070=AXIS2_PLACEMENT_3D ( 'NONE', #20213, #13240, #18720 ) ;
#4071=CARTESIAN_POINT ( 'NONE',  ( -39.66847363096314893, 93.56461422141673268, -82.92963109642393249 ) ) ;
#4072=CARTESIAN_POINT ( 'NONE',  ( -90.35604405134509420, 70.78363085573803914, 62.83509160642692848 ) ) ;
#4074=FACE_OUTER_BOUND ( 'NONE', #20360, .T. ) ;
#4076=DIRECTION ( 'NONE',  ( -0.9999164797902017066, -2.001050586450178931E-22, 0.01292414190464131508 ) ) ;
#4077=VECTOR ( 'NONE', #17450, 999.9999999999998863 ) ;
#4082=CARTESIAN_POINT ( 'NONE',  ( -92.35396912051191975, 79.82103140542292863, 31.19620131593478618 ) ) ;
#4108=CIRCLE ( 'NONE', #11476, 102.4713510550357398 ) ;
#4121=CARTESIAN_POINT ( 'NONE',  ( -88.60388113770839880, 88.93104369895573313, 50.69025205339234930 ) ) ;
#4123=ORIENTED_EDGE ( 'NONE', *, *, #10099, .F. ) ;
#4126=CARTESIAN_POINT ( 'NONE',  ( -90.33062630657602199, 70.31405425862645586, 62.77257892026059949 ) ) ;
#4132=CARTESIAN_POINT ( 'NONE',  ( 82.94572876491719171, 105.0000000000000000, -72.24960954674284608 ) ) ;
#4133=CIRCLE ( 'NONE', #18471, 2.000000000000004885 ) ;
#4134=CARTESIAN_POINT ( 'NONE',  ( 68.86686855361776338, 91.87224768293377508, -85.77506393453894873 ) ) ;
#4136=EDGE_CURVE ( 'NONE', #7130, #10247, #11091, .T. ) ;
#4139=LINE ( 'NONE', #14630, #1853 ) ;
#4150=ORIENTED_EDGE ( 'NONE', *, *, #7212, .T. ) ;
#4152=EDGE_CURVE ( 'NONE', #18705, #8847, #13279, .T. ) ;
#4157=VERTEX_POINT ( 'NONE', #21739 ) ;
#4159=CARTESIAN_POINT ( 'NONE',  ( -80.39616048656512248, 75.13699351169601925, -4.061287812893456639 ) ) ;
#4160=CARTESIAN_POINT ( 'NONE',  ( -90.14105734218799171, 88.27340299027098069, 52.93867176097701588 ) ) ;
#4164=CARTESIAN_POINT ( 'NONE',  ( -90.03465221005033925, 70.01281497139055432, 63.19621350536183968 ) ) ;
#4167=CARTESIAN_POINT ( 'NONE',  ( -89.59766859896278390, 79.73843791202820341, -28.47398564242251240 ) ) ;
#4170=PLANE ( 'NONE',  #20897 ) ;
#4174=CARTESIAN_POINT ( 'NONE',  ( 77.91909412299041549, 100.1635695855007668, -77.84996988984397603 ) ) ;
#4181=ORIENTED_EDGE ( 'NONE', *, *, #6263, .F. ) ;
#4186=AXIS2_PLACEMENT_3D ( 'NONE', #18068, #5741, #7704 ) ;
#4187=VECTOR ( 'NONE', #11318, 1000.000000000000114 ) ;
#4188=CARTESIAN_POINT ( 'NONE',  ( -41.58451242677338655, 92.58578643762699301, -83.88377541325537834 ) ) ;
#4189=CARTESIAN_POINT ( 'NONE',  ( -88.38923523735466858, 71.30869604672952278, 62.51339856172231890 ) ) ;
#4192=ADVANCED_FACE ( 'NONE', ( #11192 ), #13145, .T. ) ;
#4193=VERTEX_POINT ( 'NONE', #2691 ) ;
#4194=CARTESIAN_POINT ( 'NONE',  ( -68.81222610331992939, 91.74143318381844381, 85.81887827424428394 ) ) ;
#4200=DIRECTION ( 'NONE',  ( 0.01292414190464131508, 1.902755938799530474E-22, 0.9999164797902017066 ) ) ;
#4201=CARTESIAN_POINT ( 'NONE',  ( -92.46788464407291031, 79.04398536104956463, 28.62013883513307633 ) ) ;
#4211=DIRECTION ( 'NONE',  ( 0.01292414190463830014, 0.000000000000000000, 0.9999164797902017066 ) ) ;
#4228=AXIS2_PLACEMENT_3D ( 'NONE', #18067, #14515, #2187 ) ;
#4237=CARTESIAN_POINT ( 'NONE',  ( -89.75533239802831531, 88.06778622492817021, 50.74386735540385018 ) ) ;
#4246=CARTESIAN_POINT ( 'NONE',  ( -64.99457118636308905, 169.9999999999999716, 0.8400692238016759239 ) ) ;
#4248=DIRECTION ( 'NONE',  ( -0.8789675987075231678, -8.853465811791729457E-23, 0.4768814951561137772 ) ) ;
#4254=FACE_OUTER_BOUND ( 'NONE', #16883, .T. ) ;
#4262=EDGE_CURVE ( 'NONE', #591, #10951, #13537, .T. ) ;
#4266=CARTESIAN_POINT ( 'NONE',  ( -84.60707546407849122, 75.02634323965497742, -1.164978116754957771 ) ) ;
#4267=CARTESIAN_POINT ( 'NONE',  ( -90.15346953873444136, 88.07696337361356598, 53.07426884559318125 ) ) ;
#4269=EDGE_LOOP ( 'NONE', ( #231, #6753, #21787, #6223 ) ) ;
#4273=CARTESIAN_POINT ( 'NONE',  ( -37.52478479851671977, 92.78536193177781399, -82.71535724525422495 ) ) ;
#4274=CARTESIAN_POINT ( 'NONE',  ( 70.91392079944854743, 72.00000000000000000, 84.09052168258639881 ) ) ;
#4286=EDGE_CURVE ( 'NONE', #1373, #10917, #15948, .T. ) ;
#4303=CIRCLE ( 'NONE', #17165, 6.499999999999998224 ) ;
#4304=CARTESIAN_POINT ( 'NONE',  ( 91.14374963600242552, 79.10773180776112667, -28.81380175419844747 ) ) ;
#4308=VERTEX_POINT ( 'NONE', #8621 ) ;
#4310=CYLINDRICAL_SURFACE ( 'NONE', #15803, 2.000000000000001332 ) ;
#4312=ADVANCED_FACE ( 'NONE', ( #13589 ), #12441, .T. ) ;
#4314=EDGE_CURVE ( 'NONE', #784, #7249, #17383, .T. ) ;
#4316=ORIENTED_EDGE ( 'NONE', *, *, #11636, .T. ) ;
#4320=DIRECTION ( 'NONE',  ( -0.01292414190463832269, 0.000000000000000000, -0.9999164797902017066 ) ) ;
#4321=CARTESIAN_POINT ( 'NONE',  ( 79.92740525950247843, 54.99999999999999289, -6.133505399301337313 ) ) ;
#4322=ADVANCED_FACE ( 'NONE', ( #22280 ), #15662, .F. ) ;
#4326=CARTESIAN_POINT ( 'NONE',  ( 82.08478915011154697, 104.7581306074484502, -73.22697298855671022 ) ) ;
#4343=CARTESIAN_POINT ( 'NONE',  ( -89.79597934609442689, 88.02156722422921575, 50.77260141037600505 ) ) ;
#4349=B_SPLINE_CURVE_WITH_KNOTS ( 'NONE', 3,
 ( #10496, #14067, #1759, #14291, #15791, #3367, #9084, #10384, #15914, #3587, #265, #21162, #17401, #1656, #159, #21051 ),
 .UNSPECIFIED., .F., .F.,
 ( 4, 2, 2, 2, 2, 2, 2, 4 ),
 ( 0.000000000000000000, 0.0003989366781685740491, 0.0007978733563371480982, 0.001196810034505722256, 0.001595746712674296196, 0.001994683390842870354, 0.002393620069011444512, 0.003191493425348546423 ),
 .UNSPECIFIED. ) ;
#4355=CARTESIAN_POINT ( 'NONE',  ( 69.43142427201327394, 92.58578643762697880, -85.31868097644085935 ) ) ;
#4360=CARTESIAN_POINT ( 'NONE',  ( -91.44886093103750113, 77.80125034018028884, -29.89077835665236194 ) ) ;
#4363=AXIS2_PLACEMENT_3D ( 'NONE', #16513, #14681, #21635 ) ;
#4364=ORIENTED_EDGE ( 'NONE', *, *, #9061, .T. ) ;
#4374=CARTESIAN_POINT ( 'NONE',  ( -88.16246648193536828, 88.15220846790596454, 52.99592978592204418 ) ) ;
#4376=CIRCLE ( 'NONE', #9152, 1.999999999999997780 ) ;
#4380=CIRCLE ( 'NONE', #16168, 2.000000000000001332 ) ;
#4381=CARTESIAN_POINT ( 'NONE',  ( -63.96886132962884375, 101.1306801061894589, 76.70246874139444060 ) ) ;
#4384=CARTESIAN_POINT ( 'NONE',  ( 69.75324274910624922, 70.27959272172267902, 85.05633583411396614 ) ) ;
#4388=DIRECTION ( 'NONE',  ( -0.9999164797902017066, -2.001050586450178931E-22, 0.01292414190464131508 ) ) ;
#4390=DIRECTION ( 'NONE',  ( -2.025474946048326158E-22, 1.000000000000000000, -1.876735158486679638E-22 ) ) ;
#4395=AXIS2_PLACEMENT_3D ( 'NONE', #11758, #18751, #13598 ) ;
#4396=B_SPLINE_CURVE_WITH_KNOTS ( 'NONE', 3,
 ( #13532, #6409, #8128, #3165, #13197, #2838, #15038, #3067, #18472, #15273, #13426, #11810, #18909, #15158 ),
 .UNSPECIFIED., .F., .F.,
 ( 4, 2, 2, 2, 2, 2, 4 ),
 ( 0.000000000000000000, 0.001026194940722953983, 0.001539292411084414169, 0.002052389881445874573, 0.003078584822168784537, 0.003591682292530240170, 0.004104779762891694501 ),
 .UNSPECIFIED. ) ;
#4404=VERTEX_POINT ( 'NONE', #1173 ) ;
#4409=CARTESIAN_POINT ( 'NONE',  ( 75.44114733820232743, 75.02649460866172149, 1.289693752222738299 ) ) ;
#4415=CIRCLE ( 'NONE', #14723, 85.00000000000001421 ) ;
#4418=CARTESIAN_POINT ( 'NONE',  ( -72.65963751957909267, 87.42236182341126494, 69.77244766351077487 ) ) ;
#4419=FACE_OUTER_BOUND ( 'NONE', #17597, .T. ) ;
#4421=CARTESIAN_POINT ( 'NONE',  ( 68.58360120290730322, 71.33040186743643574, -86.00170974875821628 ) ) ;
#4423=CIRCLE ( 'NONE', #20190, 1.999999999999997780 ) ;
#4428=CARTESIAN_POINT ( 'NONE',  ( 65.93268019054301021, 104.4142135623730638, 71.73965483371370055 ) ) ;
#4447=B_SPLINE_CURVE_WITH_KNOTS ( 'NONE', 3,
 ( #2777, #2876, #949, #20548, #21920, #11851 ),
 .UNSPECIFIED., .F., .F.,
 ( 4, 2, 4 ),
 ( 2.403703357979454770E-17, 0.0009937831915592853973, 0.001987566383118546508 ),
 .UNSPECIFIED. ) ;
#4456=VERTEX_POINT ( 'NONE', #17763 ) ;
#4463=AXIS2_PLACEMENT_3D ( 'NONE', #16763, #10084, #11580 ) ;
#4465=CARTESIAN_POINT ( 'NONE',  ( -88.17195568186734533, 88.85982347399621517, 52.11040125407321000 ) ) ;
#4476=EDGE_CURVE ( 'NONE', #4193, #21164, #14557, .T. ) ;
#4479=CARTESIAN_POINT ( 'NONE',  ( -72.65712060336477407, 87.67824255507785836, 70.07990617929104360 ) ) ;
#4480=CARTESIAN_POINT ( 'NONE',  ( -75.30975508861040169, 94.90914755154933857, 80.17755788556743823 ) ) ;
#4485=ORIENTED_EDGE ( 'NONE', *, *, #1223, .T. ) ;
#4495=CARTESIAN_POINT ( 'NONE',  ( -90.17314623510533522, 87.05539508966613482, 51.36443554363990671 ) ) ;
#4498=ORIENTED_EDGE ( 'NONE', *, *, #18557, .F. ) ;
#4504=CARTESIAN_POINT ( 'NONE',  ( 70.91392079944856164, 71.82437938702648239, 84.09052168258639881 ) ) ;
#4506=VERTEX_POINT ( 'NONE', #392 ) ;
#4517=DIRECTION ( 'NONE',  ( -0.9999164797902017066, -2.001050586450178931E-22, 0.01292414190464131508 ) ) ;
#4518=DIRECTION ( 'NONE',  ( -0.01292414190464131335, 0.000000000000000000, -0.9999164797902015955 ) ) ;
#4528=DIRECTION ( 'NONE',  ( 2.025474946048326158E-22, -1.000000000000000000, 1.876735158486679638E-22 ) ) ;
#4529=DIRECTION ( 'NONE',  ( 2.025474946048326158E-22, -1.000000000000000000, 1.876735158486679638E-22 ) ) ;
#4531=VECTOR ( 'NONE', #12580, 1000.000000000000000 ) ;
#4532=CARTESIAN_POINT ( 'NONE',  ( -107.9412751340845773, 77.72595396897818887, -21.65777188997713765 ) ) ;
#4539=DIRECTION ( 'NONE',  ( -0.9999164797902015955, -2.001050586450178695E-22, 0.01292414190464131335 ) ) ;
#4540=CARTESIAN_POINT ( 'NONE',  ( 89.76942472236373760, 79.35227432041557449, -29.58847612530787075 ) ) ;
#4541=CARTESIAN_POINT ( 'NONE',  ( 93.18852247616533191, 70.03011042807717956, 58.44685241948164389 ) ) ;
#4550=CIRCLE ( 'NONE', #12259, 5.099999999999992539 ) ;
#4558=ORIENTED_EDGE ( 'NONE', *, *, #8262, .T. ) ;
#4559=VECTOR ( 'NONE', #21959, 1000.000000000000000 ) ;
#4579=ORIENTED_EDGE ( 'NONE', *, *, #3039, .T. ) ;
#4590=ORIENTED_EDGE ( 'NONE', *, *, #17530, .F. ) ;
#4594=CYLINDRICAL_SURFACE ( 'NONE', #12526, 5.099999999999994316 ) ;
#4595=CARTESIAN_POINT ( 'NONE',  ( -77.73934989822751618, 90.41888789451962793, 77.89547054214936850 ) ) ;
#4608=CARTESIAN_POINT ( 'NONE',  ( -88.16421018802580534, 88.33740264743815374, 52.84970504259129598 ) ) ;
#4611=ORIENTED_EDGE ( 'NONE', *, *, #1301, .F. ) ;
#4618=CARTESIAN_POINT ( 'NONE',  ( -88.95538863342423497, 79.66477516473727860, 30.55627054544664034 ) ) ;
#4623=CARTESIAN_POINT ( 'NONE',  ( -88.82263333796721838, 169.9999999999999716, 1.148052203164671159 ) ) ;
#4637=VERTEX_POINT ( 'NONE', #14617 ) ;
#4649=ORIENTED_EDGE ( 'NONE', *, *, #14599, .F. ) ;
#4664=LINE ( 'NONE', #9978, #7034 ) ;
#4667=CARTESIAN_POINT ( 'NONE',  ( -72.65623182917823897, 87.80665977804258659, 70.23323934248251987 ) ) ;
#4668=LINE ( 'NONE', #11703, #10657 ) ;
#4673=FACE_OUTER_BOUND ( 'NONE', #21738, .T. ) ;
#4676=ORIENTED_EDGE ( 'NONE', *, *, #7112, .T. ) ;
#4678=CARTESIAN_POINT ( 'NONE',  ( 90.64608739977012419, 77.80075968338644543, -32.24365086765053690 ) ) ;
#4679=CARTESIAN_POINT ( 'NONE',  ( -40.65822637310711940, 69.99999999999998579, -84.25167897319538213 ) ) ;
#4688=CARTESIAN_POINT ( 'NONE',  ( 35.70966224000307676, 93.64690829573217457, -83.82160924484935549 ) ) ;
#4690=ORIENTED_EDGE ( 'NONE', *, *, #18087, .T. ) ;
#4691=PLANE ( 'NONE',  #5915 ) ;
#4695=ADVANCED_FACE ( 'NONE', ( #18706 ), #8828, .T. ) ;
#4706=CARTESIAN_POINT ( 'NONE',  ( -90.01244464125365141, 88.69783294518954619, 52.52355859850199238 ) ) ;
#4708=ADVANCED_FACE ( 'NONE', ( #722 ), #11705, .T. ) ;
#4709=EDGE_LOOP ( 'NONE', ( #12134, #6691, #10533, #3291 ) ) ;
#4711=CARTESIAN_POINT ( 'NONE',  ( -74.32951741256083267, 95.10877321710717069, 82.85879239736101454 ) ) ;
#4714=CARTESIAN_POINT ( 'NONE',  ( 41.12105953731187924, 72.00000000000000000, 86.47576806556189410 ) ) ;
#4716=CARTESIAN_POINT ( 'NONE',  ( -88.16990797496626442, 88.76523295132392377, 52.31899320048508883 ) ) ;
#4722=SPHERICAL_SURFACE ( 'NONE', #4395, 2.000000000000000000 ) ;
#4724=CARTESIAN_POINT ( 'NONE',  ( 88.44888535621197434, 80.14369956782289250, -31.98268552584476154 ) ) ;
#4728=EDGE_LOOP ( 'NONE', ( #615, #8980, #21413 ) ) ;
#4732=CARTESIAN_POINT ( 'NONE',  ( -64.00981946984995830, 100.1573520573350464, 77.02845195036117332 ) ) ;
#4736=CARTESIAN_POINT ( 'NONE',  ( -88.73563860332647835, 70.69168859156255280, 62.81961162809064803 ) ) ;
#4739=ORIENTED_EDGE ( 'NONE', *, *, #7083, .F. ) ;
#4743=CARTESIAN_POINT ( 'NONE',  ( -106.1636641531658398, 79.04398536104955042, 28.79715981783285628 ) ) ;
#4751=AXIS2_PLACEMENT_3D ( 'NONE', #15611, #17000, #1263 ) ;
#4752=CARTESIAN_POINT ( 'NONE',  ( 90.47544334248004816, 78.08471258854567054, -32.66922098773476790 ) ) ;
#4776=CARTESIAN_POINT ( 'NONE',  ( 106.2089377515399065, 77.12912189496647386, 28.62973177816241588 ) ) ;
#4780=CIRCLE ( 'NONE', #4055, 2.000000000000001332 ) ;
#4781=ORIENTED_EDGE ( 'NONE', *, *, #13973, .F. ) ;
#4783=ORIENTED_EDGE ( 'NONE', *, *, #8641, .F. ) ;
#4789=CARTESIAN_POINT ( 'NONE',  ( -89.18698784711349958, 88.49522953700143546, 50.47455866862448204 ) ) ;
#4792=AXIS2_PLACEMENT_3D ( 'NONE', #9380, #7645, #2490 ) ;
#4793=CARTESIAN_POINT ( 'NONE',  ( -64.13742787616538976, 91.41757367590341232, 67.15563026703152616 ) ) ;
#4794=DIRECTION ( 'NONE',  ( 0.9999164797902017066, 2.001050586450178931E-22, -0.01292414190464131508 ) ) ;
#4799=FACE_OUTER_BOUND ( 'NONE', #7841, .T. ) ;
#4806=CARTESIAN_POINT ( 'NONE',  ( -89.97609184686128003, 87.77209961377428726, 50.92695616138752257 ) ) ;
#4817=VECTOR ( 'NONE', #14915, 1000.000000000000114 ) ;
#4822=AXIS2_PLACEMENT_3D ( 'NONE', #18602, #8595, #2866 ) ;
#4824=EDGE_CURVE ( 'NONE', #6959, #19631, #5802, .T. ) ;
#4825=CARTESIAN_POINT ( 'NONE',  ( -88.16428333377376703, 88.34422939329346036, 52.84359960540316337 ) ) ;
#4827=ORIENTED_EDGE ( 'NONE', *, *, #21735, .F. ) ;
#4830=CARTESIAN_POINT ( 'NONE',  ( -19.94685613197333751, 88.10794472606065142, -76.88480816673754248 ) ) ;
#4835=CIRCLE ( 'NONE', #3752, 1.999999999999997335 ) ;
#4836=CIRCLE ( 'NONE', #19525, 102.4713510550357398 ) ;
#4840=DIRECTION ( 'NONE',  ( -2.025474946048326158E-22, 1.000000000000000000, -1.876735158486679638E-22 ) ) ;
#4841=FACE_OUTER_BOUND ( 'NONE', #19750, .T. ) ;
#4842=LINE ( 'NONE', #6480, #6143 ) ;
#4853=VECTOR ( 'NONE', #14488, 1000.000000000000114 ) ;
#4857=EDGE_CURVE ( 'NONE', #15892, #21893, #571, .T. ) ;
#4859=ORIENTED_EDGE ( 'NONE', *, *, #12599, .F. ) ;
#4863=CARTESIAN_POINT ( 'NONE',  ( -108.6051929143322781, 76.36431273661725072, 17.61389195241277150 ) ) ;
#4874=ORIENTED_EDGE ( 'NONE', *, *, #1920, .F. ) ;
#4875=CARTESIAN_POINT ( 'NONE',  ( 91.62437796271727564, 72.00000000000000000, 60.86849236629024773 ) ) ;
#4887=CARTESIAN_POINT ( 'NONE',  ( -70.78416300399055672, 71.33159407511109862, -84.19980244608493081 ) ) ;
#4895=AXIS2_PLACEMENT_3D ( 'NONE', #1426, #20701, #8405 ) ;
#4911=CIRCLE ( 'NONE', #3833, 95.00000000000004263 ) ;
#4921=CARTESIAN_POINT ( 'NONE',  ( 84.52636712416138209, 105.0000000000000000, -71.24109250138926086 ) ) ;
#4923=DIRECTION ( 'NONE',  ( -0.9999164797902017066, -2.001050586450178931E-22, 0.01292414190464131508 ) ) ;
#4925=DIRECTION ( 'NONE',  ( 2.025474946048326158E-22, -1.000000000000000000, 1.876735158486679638E-22 ) ) ;
#4927=ORIENTED_EDGE ( 'NONE', *, *, #13849, .F. ) ;
#4929=VERTEX_POINT ( 'NONE', #3171 ) ;
#4937=DIRECTION ( 'NONE',  ( 0.9999164797902017066, 2.001050586450180811E-22, -0.01292414190464045119 ) ) ;
#4940=CARTESIAN_POINT ( 'NONE',  ( -90.15048749786897986, 87.28265959684701158, 51.22645766322034433 ) ) ;
#4942=VERTEX_POINT ( 'NONE', #15607 ) ;
#4944=ORIENTED_EDGE ( 'NONE', *, *, #18250, .T. ) ;
#4947=CARTESIAN_POINT ( 'NONE',  ( -4.071909468699204560, 86.19497019983103314, -75.00673844656712674 ) ) ;
#4952=ORIENTED_EDGE ( 'NONE', *, *, #1542, .F. ) ;
#4957=CARTESIAN_POINT ( 'NONE',  ( 91.93574473583117879, 79.05185923607193388, -28.63941780214908661 ) ) ;
#4959=FACE_OUTER_BOUND ( 'NONE', #18652, .T. ) ;
#4969=EDGE_CURVE ( 'NONE', #17515, #7720, #7301, .T. ) ;
#4979=LINE ( 'NONE', #20382, #8104 ) ;
#4987=CYLINDRICAL_SURFACE ( 'NONE', #16916, 2.000000000000004885 ) ;
#4990=CARTESIAN_POINT ( 'NONE',  ( -91.22751156961061270, 80.31838830481380853, -30.16368815799732417 ) ) ;
#4991=ORIENTED_EDGE ( 'NONE', *, *, #14311, .F. ) ;
#5005=CARTESIAN_POINT ( 'NONE',  ( 106.7514472241618790, 78.38843585434908334, -26.63023763040614966 ) ) ;
#5012=LINE ( 'NONE', #8798, #20530 ) ;
#5022=ORIENTED_EDGE ( 'NONE', *, *, #9061, .F. ) ;
#5023=ORIENTED_EDGE ( 'NONE', *, *, #2460, .F. ) ;
#5026=LINE ( 'NONE', #12057, #3678 ) ;
#5028=ORIENTED_EDGE ( 'NONE', *, *, #3184, .T. ) ;
#5029=DIRECTION ( 'NONE',  ( 0.01125613334114018010, 0.4913919529878011949, 0.8708658036695671179 ) ) ;
#5033=VERTEX_POINT ( 'NONE', #18231 ) ;
#5034=( NAMED_UNIT ( * ) PLANE_ANGLE_UNIT ( ) SI_UNIT ( $, .RADIAN. ) );
#5035=CARTESIAN_POINT ( 'NONE',  ( 106.8361484267443871, 79.08880628745905028, 26.19276530885263199 ) ) ;
#5036=FACE_OUTER_BOUND ( 'NONE', #1616, .T. ) ;
#5043=CIRCLE ( 'NONE', #17920, 83.00000000000004263 ) ;
#5048=AXIS2_PLACEMENT_3D ( 'NONE', #17307, #8557, #6511 ) ;
#5050=CARTESIAN_POINT ( 'NONE',  ( -88.16405828868519734, 88.32225945592601590, 52.86304920464149859 ) ) ;
#5051=LINE ( 'NONE', #17374, #13739 ) ;
#5056=CARTESIAN_POINT ( 'NONE',  ( -13.23978740117499164, 86.89928506224384819, -75.66871549674861797 ) ) ;
#5058=CARTESIAN_POINT ( 'NONE',  ( 104.8202145123290876, 69.99999999999998579, -33.35749735200946731 ) ) ;
#5060=ORIENTED_EDGE ( 'NONE', *, *, #11604, .F. ) ;
#5061=ORIENTED_EDGE ( 'NONE', *, *, #3904, .F. ) ;
#5064=CARTESIAN_POINT ( 'NONE',  ( 88.63197286364696481, 79.89291707602599502, -31.24418567530321766 ) ) ;
#5073=AXIS2_PLACEMENT_3D ( 'NONE', #12203, #8612, #15888 ) ;
#5086=CARTESIAN_POINT ( 'NONE',  ( -91.62437796271721879, 72.00000000000000000, -60.86849236629028326 ) ) ;
#5097=CIRCLE ( 'NONE', #18684, 2.000000000000004885 ) ;
#5099=DIRECTION ( 'NONE',  ( 0.9999164797902015955, 2.001050586450178695E-22, -0.01292414190464131335 ) ) ;
#5106=CARTESIAN_POINT ( 'NONE',  ( -104.9795361740883521, 70.06102247219405399, 32.85291587203226271 ) ) ;
#5108=EDGE_CURVE ( 'NONE', #21164, #20198, #21235, .T. ) ;
#5119=ORIENTED_EDGE ( 'NONE', *, *, #14300, .F. ) ;
#5120=EDGE_CURVE ( 'NONE', #5033, #17368, #10950, .T. ) ;
#5126=AXIS2_PLACEMENT_3D ( 'NONE', #17087, #20615, #8230 ) ;
#5128=FACE_OUTER_BOUND ( 'NONE', #19466, .T. ) ;
#5129=( BOUNDED_CURVE ( )  B_SPLINE_CURVE ( 3, ( #7292, #14331, #7533, #5785 ),
 .UNSPECIFIED., .F., .T. ) 
 B_SPLINE_CURVE_WITH_KNOTS ( ( 4, 4 ),
 ( 5.799006443144740786, 5.835910511159155156 ),
 .UNSPECIFIED. ) 
 CURVE ( )  GEOMETRIC_REPRESENTATION_ITEM ( )  RATIONAL_B_SPLINE_CURVE ( ( 1.000000000000000000, 0.9998865107004336616, 0.9998865107004336616, 1.000000000000000000 ) ) 
 REPRESENTATION_ITEM ( '' )  );
#5130=CARTESIAN_POINT ( 'NONE',  ( 33.82085273160093664, 93.50464841319750064, -82.93470554904388337 ) ) ;
#5132=EDGE_LOOP ( 'NONE', ( #12174, #17019, #6661, #19560, #16084, #19536, #15385, #491, #18766, #6770, #14536 ) ) ;
#5133=DIRECTION ( 'NONE',  ( 0.01292414190464177652, 1.902755938799532355E-22, 0.9999164797902015955 ) ) ;
#5136=VECTOR ( 'NONE', #14814, 1000.000000000000114 ) ;
#5144=CARTESIAN_POINT ( 'NONE',  ( 90.40889375659912730, 69.99999999999998579, -33.17122784026042837 ) ) ;
#5147=VERTEX_POINT ( 'NONE', #17611 ) ;
#5151=CARTESIAN_POINT ( 'NONE',  ( 106.4939345422100985, 78.92840590577354476, 27.55192737125488023 ) ) ;
#5153=CARTESIAN_POINT ( 'NONE',  ( -41.56623493000980574, 91.17157287525390075, -82.46967996629571473 ) ) ;
#5160=ORIENTED_EDGE ( 'NONE', *, *, #22642, .T. ) ;
#5161=CARTESIAN_POINT ( 'NONE',  ( 90.02055463237803679, 71.90407553649232852, -63.21629334023821656 ) ) ;
#5163=B_SPLINE_CURVE_WITH_KNOTS ( 'NONE', 3,
 ( #2989, #22160, #8170, #1297, #15530, #22261, #15420, #8485, #18842, #11726, #10008, #6551, #9888, #2877, #13361, #10230 ),
 .UNSPECIFIED., .F., .F.,
 ( 4, 2, 2, 2, 2, 2, 2, 4 ),
 ( 0.000000000000000000, 0.0003989315947993842177, 0.0007978631895987684354, 0.001196794784398152707, 0.001595726379197536871, 0.002393589568796304547, 0.002792521163595683073, 0.003191452758395061599 ),
 .UNSPECIFIED. ) ;
#5164=CARTESIAN_POINT ( 'NONE',  ( -89.53501783834650496, 89.09639617097565178, 51.70581852932981803 ) ) ;
#5166=AXIS2_PLACEMENT_3D ( 'NONE', #18975, #10258, #10380 ) ;
#5170=CARTESIAN_POINT ( 'NONE',  ( -73.39659566742001573, 95.91349339596638401, 81.93264795988667970 ) ) ;
#5173=FILL_AREA_STYLE_COLOUR ( '', #7318 ) ;
#5174=CARTESIAN_POINT ( 'NONE',  ( 84.00592537107472424, 75.05062594699531076, -4.199599686265332643 ) ) ;
#5182=AXIS2_PLACEMENT_3D ( 'NONE', #3787, #10810, #15878 ) ;
#5186=EDGE_LOOP ( 'NONE', ( #15307, #16621, #12909, #13205, #12894, #11757, #12518, #2587, #6055, #8761, #2462, #21349, #19656, #6379, #13919, #17760, #2891, #1048, #9357, #1175, #21767, #9151, #21144, #12115, #6958, #12185, #2395, #3886, #20657, #11933, #22332, #4316, #19658, #8375, #17898, #7556, #12749, #20871 ) ) ;
#5204=CARTESIAN_POINT ( 'NONE',  ( 92.14659905926313854, 77.13858430795839638, -31.20924108170689593 ) ) ;
#5208=VECTOR ( 'NONE', #16897, 1000.000000000000114 ) ;
#5213=CARTESIAN_POINT ( 'NONE',  ( 92.64101326278361626, 79.05197601643139649, 26.25411123107249267 ) ) ;
#5214=VECTOR ( 'NONE', #1869, 1000.000000000000114 ) ;
#5217=CARTESIAN_POINT ( 'NONE',  ( -91.45164190239951552, 80.14421549785515708, -29.66212192225370359 ) ) ;
#5220=LINE ( 'NONE', #12260, #15884 ) ;
#5223=AXIS2_PLACEMENT_3D ( 'NONE', #18844, #10126, #6458 ) ;
#5231=CARTESIAN_POINT ( 'NONE',  ( 93.23587179807657321, 72.00000000000000000, 30.79757858250317071 ) ) ;
#5237=CARTESIAN_POINT ( 'NONE',  ( 40.63089462960166287, 93.08398165842314143, 83.39786430079456636 ) ) ;
#5238=CARTESIAN_POINT ( 'NONE',  ( -90.77986998051284218, 77.66088650200015309, 32.02971036561880425 ) ) ;
#5239=DIRECTION ( 'NONE',  ( 0.9999164797902017066, 2.001050586450178931E-22, -0.01292414190464131508 ) ) ;
#5252=ADVANCED_FACE ( 'NONE', ( #16463 ), #5744, .T. ) ;
#5254=CARTESIAN_POINT ( 'NONE',  ( 1.364373935098378649E-14, 105.0000000000000000, -9.836450281572198869E-15 ) ) ;
#5257=CIRCLE ( 'NONE', #3065, 110.0000000000000000 ) ;
#5258=ORIENTED_EDGE ( 'NONE', *, *, #15315, .F. ) ;
#5264=ORIENTED_EDGE ( 'NONE', *, *, #8417, .T. ) ;
#5268=FACE_OUTER_BOUND ( 'NONE', #5437, .T. ) ;
#5270=ORIENTED_EDGE ( 'NONE', *, *, #672, .F. ) ;
#5282=CARTESIAN_POINT ( 'NONE',  ( -88.16582745102967067, 88.48269947768268651, 52.70639469617027117 ) ) ;
#5283=B_SPLINE_CURVE_WITH_KNOTS ( 'NONE', 3,
 ( #19115, #1897, #5772, #14440, #7279, #2226 ),
 .UNSPECIFIED., .F., .F.,
 ( 4, 2, 4 ),
 ( 0.000000000000000000, 0.0009922935535326162220, 0.001984587107065232444 ),
 .UNSPECIFIED. ) ;
#5289=AXIS2_PLACEMENT_3D ( 'NONE', #9894, #18728, #21813 ) ;
#5298=CARTESIAN_POINT ( 'NONE',  ( -75.13217090412312871, 75.01367125662450519, 2.612192813631355914 ) ) ;
#5300=AXIS2_PLACEMENT_3D ( 'NONE', #2758, #9767, #15295 ) ;
#5304=DIRECTION ( 'NONE',  ( -0.004263634442766563518, -0.9440169652124856814, -0.3298693541575922761 ) ) ;
#5309=ORIENTED_EDGE ( 'NONE', *, *, #18645, .T. ) ;
#5315=EDGE_LOOP ( 'NONE', ( #2364, #11460 ) ) ;
#5316=EDGE_CURVE ( 'NONE', #5956, #20235, #15108, .T. ) ;
#5326=CARTESIAN_POINT ( 'NONE',  ( 92.55117574443833917, 77.19412514573775752, 28.91372802644201911 ) ) ;
#5327=CARTESIAN_POINT ( 'NONE',  ( -84.36252974213540767, 104.9530375760216856, -70.59083440939244269 ) ) ;
#5328=ORIENTED_EDGE ( 'NONE', *, *, #3442, .F. ) ;
#5331=FACE_OUTER_BOUND ( 'NONE', #6608, .T. ) ;
#5333=ADVANCED_FACE ( 'NONE', ( #14405 ), #18182, .F. ) ;
#5335=CARTESIAN_POINT ( 'NONE',  ( -91.97397837737942439, 77.39048292941923535, -29.24031187446860258 ) ) ;
#5340=ORIENTED_EDGE ( 'NONE', *, *, #5568, .T. ) ;
#5363=CARTESIAN_POINT ( 'NONE',  ( -33.79255210837673218, 93.51775827232349059, 82.92153020431163668 ) ) ;
#5366=LINE ( 'NONE', #21221, #10660 ) ;
#5371=LINE ( 'NONE', #12410, #13963 ) ;
#5373=CARTESIAN_POINT ( 'NONE',  ( -106.2089377515398780, 77.12912189496638860, -28.62973177816246206 ) ) ;
#5379=EDGE_CURVE ( 'NONE', #13946, #11196, #5753, .T. ) ;
#5380=VECTOR ( 'NONE', #14711, 1000.000000000000000 ) ;
#5385=CARTESIAN_POINT ( 'NONE',  ( -89.82946945839044872, 88.94369713871104466, 52.15294112658025938 ) ) ;
#5389=DIRECTION ( 'NONE',  ( -2.025474946048326158E-22, 1.000000000000000000, -1.876735158486679638E-22 ) ) ;
#5390=ADVANCED_FACE ( 'NONE', ( #2543 ), #18515, .T. ) ;
#5392=CARTESIAN_POINT ( 'NONE',  ( 85.09728723043602372, 74.99999364505980282, -0.7689863871492244041 ) ) ;
#5400=AXIS2_PLACEMENT_3D ( 'NONE', #5254, #12299, #22355 ) ;
#5402=CARTESIAN_POINT ( 'NONE',  ( -74.91815584878337120, 75.00179123396262071, 1.637215763915028210 ) ) ;
#5404=ORIENTED_EDGE ( 'NONE', *, *, #10803, .T. ) ;
#5411=EDGE_CURVE ( 'NONE', #4637, #20879, #1641, .T. ) ;
#5416=VERTEX_POINT ( 'NONE', #13462 ) ;
#5425=EDGE_CURVE ( 'NONE', #7368, #4157, #17990, .T. ) ;
#5427=CARTESIAN_POINT ( 'NONE',  ( -92.05960170301050027, 69.99999999999998579, 60.20821982323565180 ) ) ;
#5435=CARTESIAN_POINT ( 'NONE',  ( 92.06552853299285744, 79.93537922958523723, 29.07356135706681499 ) ) ;
#5437=EDGE_LOOP ( 'NONE', ( #11343, #3616, #3819, #21581 ) ) ;
#5440=DIRECTION ( 'NONE',  ( 0.01292414190464131335, 1.902755938799530239E-22, 0.9999164797902015955 ) ) ;
#5449=VERTEX_POINT ( 'NONE', #18512 ) ;
#5450=DIRECTION ( 'NONE',  ( -0.01292414190464131335, -1.902755938799530239E-22, -0.9999164797902015955 ) ) ;
#5462=ORIENTED_EDGE ( 'NONE', *, *, #11680, .F. ) ;
#5465=EDGE_CURVE ( 'NONE', #14836, #11011, #7669, .T. ) ;
#5472=AXIS2_PLACEMENT_3D ( 'NONE', #9423, #16243, #711 ) ;
#5476=CARTESIAN_POINT ( 'NONE',  ( 39.45590449612061690, 92.86731729162988813, 83.62973377252751561 ) ) ;
#5477=CIRCLE ( 'NONE', #3650, 2.000000000000002665 ) ;
#5478=ORIENTED_EDGE ( 'NONE', *, *, #3039, .F. ) ;
#5481=DIRECTION ( 'NONE',  ( 0.9999164797902015955, 2.001050586450178695E-22, -0.01292414190464131335 ) ) ;
#5491=CARTESIAN_POINT ( 'NONE',  ( 106.5693380255448091, 79.05027630924989523, 27.25937202119029124 ) ) ;
#5494=CIRCLE ( 'NONE', #20525, 3.999999999999995559 ) ;
#5506=CARTESIAN_POINT ( 'NONE',  ( -89.93579087582143927, 87.83132640396426893, 50.89035702524756033 ) ) ;
#5509=AXIS2_PLACEMENT_3D ( 'NONE', #10719, #1995, #15677 ) ;
#5515=CARTESIAN_POINT ( 'NONE',  ( -106.1347175484142582, 70.98259407754899541, -28.90376667366510333 ) ) ;
#5516=CARTESIAN_POINT ( 'NONE',  ( 93.21002351426729149, 77.12912189496647386, 28.79774562292276840 ) ) ;
#5519=CIRCLE ( 'NONE', #21296, 97.00000000000005684 ) ;
#5523=CARTESIAN_POINT ( 'NONE',  ( -76.19510332049942747, 75.05951099091890910, -2.385751844565587199 ) ) ;
#5535=ORIENTED_EDGE ( 'NONE', *, *, #20290, .T. ) ;
#5545=CARTESIAN_POINT ( 'NONE',  ( -89.17419594629882340, 70.48718124881995095, 62.98708966501553874 ) ) ;
#5550=DIRECTION ( 'NONE',  ( 2.025474946048326158E-22, -1.000000000000000000, 1.876735158486679638E-22 ) ) ;
#5552=ORIENTED_EDGE ( 'NONE', *, *, #2493, .F. ) ;
#5559=VECTOR ( 'NONE', #20280, 1000.000000000000114 ) ;
#5564=AXIS2_PLACEMENT_3D ( 'NONE', #405, #3555, #19519 ) ;
#5565=CARTESIAN_POINT ( 'NONE',  ( -93.05058556066501296, 79.82257531472973255, -28.80218916741304014 ) ) ;
#5568=EDGE_CURVE ( 'NONE', #22376, #13705, #5494, .T. ) ;
#5572=PRODUCT_DEFINITION_CONTEXT ( 'detailed design', #17627, 'design' ) ;
#5573=ORIENTED_EDGE ( 'NONE', *, *, #14869, .T. ) ;
#5576=CARTESIAN_POINT ( 'NONE',  ( 93.17671387018316409, 79.04398536104964990, 26.22064129356684958 ) ) ;
#5580=VERTEX_POINT ( 'NONE', #5373 ) ;
#5581=AXIS2_PLACEMENT_3D ( 'NONE', #15250, #13737, #11781 ) ;
#5584=CARTESIAN_POINT ( 'NONE',  ( 66.73173682738227797, 70.03297899285537653, -87.44705638319801722 ) ) ;
#5591=CARTESIAN_POINT ( 'NONE',  ( -66.06691928577359363, 94.02752048664900997, -82.12548041065298321 ) ) ;
#5596=DIRECTION ( 'NONE',  ( -0.9999164797902017066, -2.001050586450178931E-22, 0.01292414190464131508 ) ) ;
#5597=ADVANCED_FACE ( 'NONE', ( #12412 ), #15052, .F. ) ;
#5599=VECTOR ( 'NONE', #20292, 1000.000000000000114 ) ;
#5602=CARTESIAN_POINT ( 'NONE',  ( 41.09521125350259041, 69.99999999999998579, 84.47593510598149180 ) ) ;
#5603=EDGE_CURVE ( 'NONE', #959, #44, #4376, .T. ) ;
#5607=VECTOR ( 'NONE', #20536, 1000.000000000000000 ) ;
#5608=VERTEX_POINT ( 'NONE', #16098 ) ;
#5609=CARTESIAN_POINT ( 'NONE',  ( 89.47454773680249218, 97.89961987228680584, -63.98691110171232310 ) ) ;
#5626=CIRCLE ( 'NONE', #1603, 1.999999999999997780 ) ;
#5628=CARTESIAN_POINT ( 'NONE',  ( -88.17009401808903135, 88.77120466299882651, 52.29915554423978818 ) ) ;
#5634=LINE ( 'NONE', #477, #12180 ) ;
#5637=DIRECTION ( 'NONE',  ( 0.01292414190464131335, 0.000000000000000000, 0.9999164797902017066 ) ) ;
#5638=ORIENTED_EDGE ( 'NONE', *, *, #15278, .F. ) ;
#5648=CARTESIAN_POINT ( 'NONE',  ( -36.15575339682945355, 93.60246143706251587, -82.12095408908095351 ) ) ;
#5654=VERTEX_POINT ( 'NONE', #16664 ) ;
#5659=DIRECTION ( 'NONE',  ( -2.025474946048326158E-22, 1.000000000000000000, -1.876735158486679638E-22 ) ) ;
#5668=DIRECTION ( 'NONE',  ( 0.9999164797902017066, 2.001050586450178931E-22, -0.01292414190464131508 ) ) ;
#5670=AXIS2_PLACEMENT_3D ( 'NONE', #20814, #1655, #5304 ) ;
#5671=CARTESIAN_POINT ( 'NONE',  ( 39.42082737383938706, 91.17157287525387233, -83.51645567887783272 ) ) ;
#5683=DIRECTION ( 'NONE',  ( -0.9999164797902017066, -2.001050586450177990E-22, 0.01292414190464177999 ) ) ;
#5690=VERTEX_POINT ( 'NONE', #6420 ) ;
#5695=DIRECTION ( 'NONE',  ( 0.01292414190464131508, 0.000000000000000000, 0.9999164797902017066 ) ) ;
#5697=CARTESIAN_POINT ( 'NONE',  ( -91.90296438722893413, 77.16966923688050883, 31.25747399733658938 ) ) ;
#5705=EDGE_CURVE ( 'NONE', #2340, #12564, #20896, .T. ) ;
#5713=VERTEX_POINT ( 'NONE', #8253 ) ;
#5722=CARTESIAN_POINT ( 'NONE',  ( -28.61234839824397369, 91.18282421267417703, 80.66236699840530378 ) ) ;
#5723=ORIENTED_EDGE ( 'NONE', *, *, #13617, .T. ) ;
#5726=EDGE_CURVE ( 'NONE', #19075, #9610, #22335, .T. ) ;
#5727=ORIENTED_EDGE ( 'NONE', *, *, #22223, .T. ) ;
#5733=CARTESIAN_POINT ( 'NONE',  ( -90.17421880070757823, 70.18950621168607995, 62.99705530356752803 ) ) ;
#5741=DIRECTION ( 'NONE',  ( 0.9999164797902017066, 2.001050586450178931E-22, -0.01292414190464131508 ) ) ;
#5743=ADVANCED_FACE ( 'NONE', ( #15280 ), #13538, .F. ) ;
#5744=CYLINDRICAL_SURFACE ( 'NONE', #12830, 110.0000000000000000 ) ;
#5745=ORIENTED_EDGE ( 'NONE', *, *, #22642, .F. ) ;
#5752=DIRECTION ( 'NONE',  ( 0.5121193912974630891, -0.6668151060996335699, 0.5413791123920929094 ) ) ;
#5753=B_SPLINE_CURVE_WITH_KNOTS ( 'NONE', 3,
 ( #9194, #13122, #11618, #20092, #16582, #18284, #10004 ),
 .UNSPECIFIED., .F., .F.,
 ( 4, 3, 4 ),
 ( 0.000000000000000000, 0.004771063351880659026, 0.01050764680140206173 ),
 .UNSPECIFIED. ) ;
#5758=ORIENTED_EDGE ( 'NONE', *, *, #11338, .T. ) ;
#5760=CARTESIAN_POINT ( 'NONE',  ( -83.16258572756845524, 75.08619966718656258, -2.975792177979545983 ) ) ;
#5761=CARTESIAN_POINT ( 'NONE',  ( -90.13276696777731445, 88.30345154740933822, 52.91026065720622285 ) ) ;
#5772=CARTESIAN_POINT ( 'NONE',  ( 84.36252974213543609, 104.9530375760216714, 70.59083440939240006 ) ) ;
#5777=LINE ( 'NONE', #12475, #4046 ) ;
#5785=CARTESIAN_POINT ( 'NONE',  ( -36.55288090549052527, 94.02752048664899576, 83.45186405039063970 ) ) ;
#5788=CARTESIAN_POINT ( 'NONE',  ( -90.51228951533471445, 70.60983096564289951, 62.93517888374829994 ) ) ;
#5801=CARTESIAN_POINT ( 'NONE',  ( -90.65403358069494288, 80.14440291447093045, 32.01641220276452771 ) ) ;
#5802=LINE ( 'NONE', #12836, #8382 ) ;
#5815=CARTESIAN_POINT ( 'NONE',  ( 39.39497909003009823, 72.00000000000000000, -85.51628863845822082 ) ) ;
#5822=EDGE_CURVE ( 'NONE', #4506, #17671, #19782, .T. ) ;
#5824=EDGE_CURVE ( 'NONE', #22379, #18446, #7387, .T. ) ;
#5830=CARTESIAN_POINT ( 'NONE',  ( -72.65623182917823897, 87.80665977804258659, 70.23323934248251987 ) ) ;
#5835=CARTESIAN_POINT ( 'NONE',  ( -31.27192067738528181, 92.26000739851428989, 81.74748161169398486 ) ) ;
#5842=VECTOR ( 'NONE', #1274, 1000.000000000000000 ) ;
#5845=CARTESIAN_POINT ( 'NONE',  ( -89.88240203325172217, 87.91076060644846280, 50.84128159929887403 ) ) ;
#5848=ORIENTED_EDGE ( 'NONE', *, *, #4824, .T. ) ;
#5850=DIRECTION ( 'NONE',  ( -2.025474946048326158E-22, 1.000000000000000000, -1.876735158486679638E-22 ) ) ;
#5856=AXIS2_PLACEMENT_3D ( 'NONE', #202, #9021, #18014 ) ;
#5859=CARTESIAN_POINT ( 'NONE',  ( 87.76353177753586010, 103.0887459898907821, 66.33296338796031932 ) ) ;
#5860=AXIS2_PLACEMENT_3D ( 'NONE', #4623, #13716, #18640 ) ;
#5866=DIRECTION ( 'NONE',  ( -0.01292414190464077212, 0.000000000000000000, -0.9999164797902015955 ) ) ;
#5868=CARTESIAN_POINT ( 'NONE',  ( 91.21019055468690340, 77.12912189496647386, 28.82359390673205723 ) ) ;
#5880=CARTESIAN_POINT ( 'NONE',  ( -84.94025445842608235, 75.00896870829117802, -0.2173801658002265935 ) ) ;
#5882=CARTESIAN_POINT ( 'NONE',  ( -90.14989025201742834, 88.17731219746620752, 53.00831397183212346 ) ) ;
#5885=( BOUNDED_SURFACE ( )  B_SPLINE_SURFACE ( 3, 2, ( 
 ( #16742, #21520, #15013 ),
 ( #21965, #5788, #6266 ),
 ( #19797, #4072, #18122 ),
 ( #644, #2372, #7631 ),
 ( #21627, #12954, #19918 ),
 ( #4189, #11218, #22423 ),
 ( #10276, #22530, #3249 ),
 ( #17291, #8423, #18991 ),
 ( #20605, #10162, #18658 ),
 ( #3146, #6597, #1553 ) ),
 .UNSPECIFIED., .F., .F., .T. ) 
 B_SPLINE_SURFACE_WITH_KNOTS ( ( 4, 2, 2, 2, 4 ),
 ( 3, 3 ),
 ( 0.5394812760223721693, 0.7973100387155035440, 1.055138801408634919, 1.312967564101766182, 1.570796326794897668 ),
 ( 0.000000000000000000, 1.000000000000000000 ),
 .UNSPECIFIED. ) 
 GEOMETRIC_REPRESENTATION_ITEM ( )  RATIONAL_B_SPLINE_SURFACE ( (
 ( 1.000000000000000000, 0.8430901905886449832, 1.000000000000000000),
 ( 1.000000000000000000, 0.8366591603533565236, 1.000000000000000000),
 ( 1.000000000000000000, 0.8287607763626427815, 1.000000000000000000),
 ( 1.000000000000000000, 0.8103261952457585515, 1.000000000000000000),
 ( 1.000000000000000000, 0.7997876793901601555, 1.000000000000000000),
 ( 1.000000000000000000, 0.7764793049479934428, 1.000000000000000000),
 ( 1.000000000000000000, 0.7637087627022125513, 1.000000000000000000),
 ( 1.000000000000000000, 0.7364885232972262497, 1.000000000000000000),
 ( 1.000000000000000000, 0.7220407509482392738, 1.000000000000000000),
 ( 1.000000000000000000, 0.7071067811865463515, 1.000000000000000000) ) ) 
 REPRESENTATION_ITEM ( '' )  SURFACE ( )  );
#5889=CIRCLE ( 'NONE', #776, 97.00000000000005684 ) ;
#5893=FACE_OUTER_BOUND ( 'NONE', #1008, .T. ) ;
#5894=EDGE_CURVE ( 'NONE', #6959, #13713, #8431, .T. ) ;
#5898=CARTESIAN_POINT ( 'NONE',  ( 18.70469657817222853, 88.26328955574699364, -77.54996127225918201 ) ) ;
#5899=VECTOR ( 'NONE', #8144, 1000.000000000000114 ) ;
#5912=EDGE_CURVE ( 'NONE', #9437, #17867, #18697, .T. ) ;
#5915=AXIS2_PLACEMENT_3D ( 'NONE', #13025, #16465, #1176 ) ;
#5916=CARTESIAN_POINT ( 'NONE',  ( 75.00823711914057412, 75.00686501439010101, -2.123222951424176941 ) ) ;
#5920=CARTESIAN_POINT ( 'NONE',  ( 65.90110554552376243, 103.0000000000000000, 69.29678410920483600 ) ) ;
#5927=CARTESIAN_POINT ( 'NONE',  ( -88.42079784105915508, 80.23159800265108288, 32.23730667790417215 ) ) ;
#5950=EDGE_CURVE ( 'NONE', #17515, #15796, #20522, .T. ) ;
#5955=FACE_OUTER_BOUND ( 'NONE', #3550, .T. ) ;
#5956=VERTEX_POINT ( 'NONE', #7885 ) ;
#5959=CARTESIAN_POINT ( 'NONE',  ( -14.25982594500669975, 87.34594711659762822, 76.51465384614120069 ) ) ;
#5962=CARTESIAN_POINT ( 'NONE',  ( 35.95309506732430549, 93.50464841319750064, 82.03286182426640494 ) ) ;
#5969=CARTESIAN_POINT ( 'NONE',  ( -88.67226694823077082, 88.96335391310392993, 50.75244397949245467 ) ) ;
#5970=ADVANCED_FACE ( 'NONE', ( #20047 ), #16520, .F. ) ;
#5982=CYLINDRICAL_SURFACE ( 'NONE', #4186, 2.000000000000004885 ) ;
#5984=ORIENTED_EDGE ( 'NONE', *, *, #12021, .F. ) ;
#5988=ADVANCED_FACE ( 'NONE', ( #11227 ), #326, .T. ) ;
#6002=ADVANCED_FACE ( 'NONE', ( #20493 ), #13850, .F. ) ;
#6004=CARTESIAN_POINT ( 'NONE',  ( -84.97839964729169537, 75.00686501439008680, -0.05536024668152433881 ) ) ;
#6005=CARTESIAN_POINT ( 'NONE',  ( -90.14962381271330116, 88.05998628382424442, 53.08008600111026709 ) ) ;
#6011=DIRECTION ( 'NONE',  ( 0.01292414190464131335, 1.902755938799530239E-22, 0.9999164797902015955 ) ) ;
#6020=CARTESIAN_POINT ( 'NONE',  ( 14.26922013821070934, 87.34719917405588774, -76.51617212798838352 ) ) ;
#6023=EDGE_CURVE ( 'NONE', #4506, #5956, #20833, .T. ) ;
#6035=ADVANCED_FACE ( 'NONE', ( #19116 ), #6247, .F. ) ;
#6036=VECTOR ( 'NONE', #15260, 1000.000000000000114 ) ;
#6037=AXIS2_PLACEMENT_3D ( 'NONE', #19101, #22625, #22299 ) ;
#6039=CARTESIAN_POINT ( 'NONE',  ( 75.97949114995992659, 75.05057272691708192, 2.129988415395909218 ) ) ;
#6051=CARTESIAN_POINT ( 'NONE',  ( -70.91392079944854743, 69.99999999999998579, -84.09052168258642723 ) ) ;
#6053=ADVANCED_FACE ( 'NONE', ( #15261 ), #19001, .F. ) ;
#6054=DIRECTION ( 'NONE',  ( 0.01292414190464131335, 0.000000000000000000, 0.9999164797902017066 ) ) ;
#6055=ORIENTED_EDGE ( 'NONE', *, *, #14323, .T. ) ;
#6059=ORIENTED_EDGE ( 'NONE', *, *, #13849, .T. ) ;
#6063=CARTESIAN_POINT ( 'NONE',  ( -109.3418654547023721, 87.00751446224754204, 51.62948579205222899 ) ) ;
#6067=CARTESIAN_POINT ( 'NONE',  ( -63.91983116576977153, 91.51644034066822542, 67.07156771589210109 ) ) ;
#6076=CARTESIAN_POINT ( 'NONE',  ( 13.24479188061246759, 86.89994116914630240, 75.66937141396037703 ) ) ;
#6081=ORIENTED_EDGE ( 'NONE', *, *, #10213, .F. ) ;
#6083=CARTESIAN_POINT ( 'NONE',  ( -88.17149547474421922, 88.83987025360480061, 52.15764617096433398 ) ) ;
#6094=CARTESIAN_POINT ( 'NONE',  ( 68.71681667565952978, 91.32006346413032816, -85.89527988174788220 ) ) ;
#6096=CARTESIAN_POINT ( 'NONE',  ( 37.83293359763302988, 93.41702043944185618, -84.07896005542636431 ) ) ;
#6099=CARTESIAN_POINT ( 'NONE',  ( -109.6289368035921683, 77.12912189496647386, 29.41931704363643618 ) ) ;
#6105=DIRECTION ( 'NONE',  ( 2.025474946048326158E-22, -1.000000000000000000, 1.876735158486679638E-22 ) ) ;
#6109=ORIENTED_EDGE ( 'NONE', *, *, #6225, .F. ) ;
#6111=CARTESIAN_POINT ( 'NONE',  ( -83.41629690720331780, 75.07731437015503673, -2.761324039041341827 ) ) ;
#6112=EDGE_CURVE ( 'NONE', #19328, #6852, #15357, .T. ) ;
#6113=CARTESIAN_POINT ( 'NONE',  ( -88.16190907930861442, 88.08529935286561852, 53.04065179493614579 ) ) ;
#6114=ADVANCED_FACE ( 'NONE', ( #19573 ), #12367, .T. ) ;
#6118=EDGE_CURVE ( 'NONE', #198, #11245, #20539, .T. ) ;
#6121=CARTESIAN_POINT ( 'NONE',  ( -93.17671387018313567, 79.04398536104955042, -26.22064129356660800 ) ) ;
#6122=CARTESIAN_POINT ( 'NONE',  ( 70.78416300399058514, 71.33159407511109862, 84.19980244608490239 ) ) ;
#6124=AXIS2_PLACEMENT_3D ( 'NONE', #14744, #4248, #11270 ) ;
#6129=CARTESIAN_POINT ( 'NONE',  ( 11.27395757585026637, 86.89847835976068779, -75.98467626014961240 ) ) ;
#6135=CARTESIAN_POINT ( 'NONE',  ( 91.10494378670944116, 97.90071567704912070, 61.64404307423180995 ) ) ;
#6140=DIRECTION ( 'NONE',  ( -2.459148776294495979E-24, 1.000000000000000000, -1.902597020224326827E-22 ) ) ;
#6143=VECTOR ( 'NONE', #13600, 1000.000000000000000 ) ;
#6144=EDGE_CURVE ( 'NONE', #11245, #11382, #19347, .T. ) ;
#6160=CARTESIAN_POINT ( 'NONE',  ( 90.41664810497508142, 79.20851322806770156, -29.13399567714613525 ) ) ;
#6162=DIRECTION ( 'NONE',  ( 0.01292414190464270286, 1.902755938799533530E-22, 0.9999164797902017066 ) ) ;
#6167=FACE_OUTER_BOUND ( 'NONE', #16034, .T. ) ;
#6175=EDGE_CURVE ( 'NONE', #21849, #10639, #2445, .T. ) ;
#6179=ORIENTED_EDGE ( 'NONE', *, *, #16567, .T. ) ;
#6184=CARTESIAN_POINT ( 'NONE',  ( -106.6839260360359987, 79.12661604778574542, -26.80604816241528709 ) ) ;
#6186=CARTESIAN_POINT ( 'NONE',  ( 105.6473595942261738, 69.99999999999998579, 30.63715735456338862 ) ) ;
#6187=DIRECTION ( 'NONE',  ( -2.025474946048326158E-22, 1.000000000000000000, -1.876735158486679638E-22 ) ) ;
#6194=CARTESIAN_POINT ( 'NONE',  ( -88.17226140160809678, 88.87231815780248212, 52.07896878194610935 ) ) ;
#6198=ORIENTED_EDGE ( 'NONE', *, *, #7756, .T. ) ;
#6199=ORIENTED_EDGE ( 'NONE', *, *, #7835, .T. ) ;
#6213=CARTESIAN_POINT ( 'NONE',  ( 84.78539177974978713, 105.0000000000000000, 70.08164767436862519 ) ) ;
#6219=FACE_OUTER_BOUND ( 'NONE', #11180, .T. ) ;
#6223=ORIENTED_EDGE ( 'NONE', *, *, #19213, .F. ) ;
#6225=EDGE_CURVE ( 'NONE', #5690, #19747, #7863, .T. ) ;
#6226=CARTESIAN_POINT ( 'NONE',  ( -88.16157026904535599, 88.04290212818546024, 53.06700061362209908 ) ) ;
#6238=CARTESIAN_POINT ( 'NONE',  ( -88.41758806590422637, 80.31838830481380853, 32.48564084813592956 ) ) ;
#6239=CARTESIAN_POINT ( 'NONE',  ( 70.88639693877763648, 71.65513756697318115, 84.11375151051876742 ) ) ;
#6247=TOROIDAL_SURFACE ( 'NONE', #5126, 83.00000000000001421, 2.000000000000000000 ) ;
#6249=CIRCLE ( 'NONE', #7337, 95.00000000000004263 ) ;
#6250=CARTESIAN_POINT ( 'NONE',  ( -39.42082737383935154, 72.00000000000000000, 83.51645567887779009 ) ) ;
#6251=CARTESIAN_POINT ( 'NONE',  ( -91.23603883849614249, 78.43035437438885538, -30.82342686631250217 ) ) ;
#6263=EDGE_CURVE ( 'NONE', #11245, #2836, #762, .T. ) ;
#6265=CARTESIAN_POINT ( 'NONE',  ( 76.82405103886378583, 75.08619966718657679, -5.043654882722200306 ) ) ;
#6266=CARTESIAN_POINT ( 'NONE',  ( -90.86534537526709698, 70.37233884329080524, 61.70249327685399976 ) ) ;
#6269=AXIS2_PLACEMENT_3D ( 'NONE', #20101, #10942, #2967 ) ;
#6272=EDGE_LOOP ( 'NONE', ( #21034, #13219, #16625, #15937 ) ) ;
#6274=VERTEX_POINT ( 'NONE', #7962 ) ;
#6276=CARTESIAN_POINT ( 'NONE',  ( 90.02055463237803679, 95.44063823554751025, -63.21629334023821656 ) ) ;
#6279=CARTESIAN_POINT ( 'NONE',  ( 90.99469209931193348, 80.00980328568967082, -31.64094806796699544 ) ) ;
#6282=DIRECTION ( 'NONE',  ( 0.01125613334114014194, 0.4913919529878064685, 0.8708658036695641202 ) ) ;
#6286=VERTEX_POINT ( 'NONE', #21948 ) ;
#6287=CARTESIAN_POINT ( 'NONE',  ( -2.067862704742604141, 72.00000000000000000, -159.9866367664322979 ) ) ;
#6292=AXIS2_PLACEMENT_3D ( 'NONE', #3102, #12069, #1395 ) ;
#6295=VECTOR ( 'NONE', #20521, 1000.000000000000000 ) ;
#6305=DIRECTION ( 'NONE',  ( 2.025474946048326158E-22, -1.000000000000000000, 1.876735158486679638E-22 ) ) ;
#6331=CARTESIAN_POINT ( 'NONE',  ( -33.82085273160089400, 93.50464841319747222, 82.93470554904384073 ) ) ;
#6334=DIRECTION ( 'NONE',  ( 0.01292414190464131508, 0.000000000000000000, 0.9999164797902017066 ) ) ;
#6335=ORIENTED_EDGE ( 'NONE', *, *, #3564, .T. ) ;
#6339=FACE_OUTER_BOUND ( 'NONE', #2451, .T. ) ;
#6341=DIRECTION ( 'NONE',  ( 0.01292414190464131335, 1.902755938799530239E-22, 0.9999164797902015955 ) ) ;
#6354=CARTESIAN_POINT ( 'NONE',  ( -90.09729892282578589, 88.47696219913342475, 52.76108841404412431 ) ) ;
#6365=CARTESIAN_POINT ( 'NONE',  ( -63.92582232734818604, 91.13550884953522768, 66.60804284595937474 ) ) ;
#6370=CARTESIAN_POINT ( 'NONE',  ( -90.00466877033377955, 70.05991977044968166, 63.23890890537643372 ) ) ;
#6378=CARTESIAN_POINT ( 'NONE',  ( -64.02441888546434257, 100.0345687961148826, 75.89892270379247918 ) ) ;
#6379=ORIENTED_EDGE ( 'NONE', *, *, #12796, .T. ) ;
#6383=CARTESIAN_POINT ( 'NONE',  ( 0.6170534444071897884, 95.45144721132757581, 47.74026101898994767 ) ) ;
#6386=CARTESIAN_POINT ( 'NONE',  ( -64.28883878761490678, 83.29019440189556178, 55.44125366118054643 ) ) ;
#6396=CARTESIAN_POINT ( 'NONE',  ( -68.69096839185023384, 69.99999999999998579, 87.89511284132827029 ) ) ;
#6397=ADVANCED_FACE ( 'NONE', ( #20365 ), #6804, .T. ) ;
#6398=CARTESIAN_POINT ( 'NONE',  ( 90.61229378181252514, 77.84360403296375353, -32.30868923918635005 ) ) ;
#6409=CARTESIAN_POINT ( 'NONE',  ( -66.45999312048353147, 70.00000000000000000, 87.65380681892987980 ) ) ;
#6413=CARTESIAN_POINT ( 'NONE',  ( -1.163172771417704698, 45.00000000000000000, -89.99248318111816047 ) ) ;
#6417=ORIENTED_EDGE ( 'NONE', *, *, #2258, .F. ) ;
#6418=ORIENTED_EDGE ( 'NONE', *, *, #7525, .F. ) ;
#6420=CARTESIAN_POINT ( 'NONE',  ( -93.23587179807654479, 69.99999999999998579, -30.79757858250321689 ) ) ;
#6422=LINE ( 'NONE', #17106, #21771 ) ;
#6423=FACE_OUTER_BOUND ( 'NONE', #1868, .T. ) ;
#6428=ADVANCED_FACE ( 'NONE', ( #4959 ), #15452, .F. ) ;
#6429=DIRECTION ( 'NONE',  ( -2.025474946048326158E-22, 1.000000000000000000, -1.876735158486678933E-22 ) ) ;
#6440=CARTESIAN_POINT ( 'NONE',  ( 91.12451015595509318, 77.41163679146359300, -31.64200013680036605 ) ) ;
#6458=DIRECTION ( 'NONE',  ( 0.01292414190464179213, 0.000000000000000000, 0.9999164797902017066 ) ) ;
#6460=LINE ( 'NONE', #15319, #2861 ) ;
#6461=PLANE ( 'NONE',  #11806 ) ;
#6465=CARTESIAN_POINT ( 'NONE',  ( -90.00978037925260367, 88.71181518729869708, 52.51177033982978770 ) ) ;
#6468=EDGE_CURVE ( 'NONE', #20544, #12076, #12039, .T. ) ;
#6469=CARTESIAN_POINT ( 'NONE',  ( -75.24529543015454180, 95.02827877570439341, 80.23810401866792574 ) ) ;
#6473=CARTESIAN_POINT ( 'NONE',  ( -88.17696233076783585, 88.99987371843837991, 51.57339716971453925 ) ) ;
#6477=EDGE_LOOP ( 'NONE', ( #21042, #18427, #4181, #13987, #3507, #12855, #15167 ) ) ;
#6480=CARTESIAN_POINT ( 'NONE',  ( 1.117803423002110774, 45.00000000000000000, 109.6947150755565161 ) ) ;
#6487=VERTEX_POINT ( 'NONE', #19320 ) ;
#6493=EDGE_CURVE ( 'NONE', #4942, #21601, #4780, .T. ) ;
#6497=CARTESIAN_POINT ( 'NONE',  ( -109.9283388797385612, 75.00188554563106891, 6.129144436280878239 ) ) ;
#6499=( BOUNDED_SURFACE ( )  B_SPLINE_SURFACE ( 3, 2, ( 
 ( #21435, #19813, #4201 ),
 ( #16194, #4082, #11116 ),
 ( #7308, #2037, #432 ),
 ( #5697, #15965, #9140 ),
 ( #7549, #7430, #12728 ),
 ( #7200, #19595, #9023 ),
 ( #19483, #9262, #19696 ),
 ( #12965, #3963, #12617 ),
 ( #314, #14348, #14577 ),
 ( #10987, #3867, #18016 ),
 ( #11229, #10880, #21641 ),
 ( #10770, #18136, #21317 ),
 ( #204, #2260, #17906 ),
 ( #550, #21531, #2387 ),
 ( #14231, #5801, #3757 ),
 ( #12835, #9379, #17800 ),
 ( #16413, #659, #5927 ),
 ( #14690, #19932, #21206 ) ),
 .UNSPECIFIED., .F., .F., .T. ) 
 B_SPLINE_SURFACE_WITH_KNOTS ( ( 4, 2, 2, 2, 2, 2, 2, 2, 4 ),
 ( 3, 3 ),
 ( 0.002597246120634467796, 0.003399884678228190776, 0.004202523235821913755, 0.005005161793415637168, 0.005807800351009360582, 0.006610438908603083995, 0.007413077466196807408, 0.008215716023790529954, 0.009018354581384254234 ),
 ( 0.000000000000000000, 1.000000000000000000 ),
 .UNSPECIFIED. ) 
 GEOMETRIC_REPRESENTATION_ITEM ( )  RATIONAL_B_SPLINE_SURFACE ( (
 ( 1.000000000000000000, 0.5963808372950819559, 1.000000000000000000),
 ( 1.000000000000000000, 0.5963839598476180504, 1.000000000000000000),
 ( 1.000000000000000000, 0.5970886094880794026, 1.000000000000000000),
 ( 1.000000000000000000, 0.5998681984913176723, 1.000000000000000000),
 ( 1.000000000000000000, 0.6019790828716353737, 1.000000000000000000),
 ( 1.000000000000000000, 0.6074656362385493225, 1.000000000000000000),
 ( 1.000000000000000000, 0.6108290540004431834, 1.000000000000000000),
 ( 1.000000000000000000, 0.6188252630046991998, 1.000000000000000000),
 ( 1.000000000000000000, 0.6234423941985007822, 1.000000000000000000),
 ( 1.000000000000000000, 0.6335838931037276467, 1.000000000000000000),
 ( 1.000000000000000000, 0.6391861101551582491, 1.000000000000000000),
 ( 1.000000000000000000, 0.6512661799281685981, 1.000000000000000000),
 ( 1.000000000000000000, 0.6576333021886564545, 1.000000000000000000),
 ( 1.000000000000000000, 0.6710088154586895115, 1.000000000000000000),
 ( 1.000000000000000000, 0.6780884601156411673, 1.000000000000000000),
 ( 1.000000000000000000, 0.6924279500034853374, 1.000000000000000000),
 ( 1.000000000000000000, 0.6997125326201852902, 1.000000000000000000),
 ( 1.000000000000000000, 0.7071067811865473507, 1.000000000000000000) ) ) 
 REPRESENTATION_ITEM ( '' )  SURFACE ( )  );
#6504=CARTESIAN_POINT ( 'NONE',  ( 90.73345939407627725, 80.10652859373304580, -31.90946778207672097 ) ) ;
#6508=DIRECTION ( 'NONE',  ( 0.01292414190464174703, 0.000000000000000000, 0.9999164797902015955 ) ) ;
#6510=VERTEX_POINT ( 'NONE', #1755 ) ;
#6511=DIRECTION ( 'NONE',  ( -0.01292414190464131335, 0.000000000000000000, -0.9999164797902017066 ) ) ;
#6516=DIRECTION ( 'NONE',  ( 2.025474946048326158E-22, -1.000000000000000000, 1.876735158486679638E-22 ) ) ;
#6520=B_SPLINE_CURVE_WITH_KNOTS ( 'NONE', 3,
 ( #11255, #5835, #5722, #14834, #7911, #2636, #12755, #9521, #16552, #5959, #18162, #806, #3894, #21891, #9402, #21785, #14607, #2169, #9168, #6076, #14947, #16439, #19626, #7575, #20072, #10910, #462, #689 ),
 .UNSPECIFIED., .F., .F.,
 ( 4, 2, 2, 2, 2, 2, 2, 2, 2, 2, 2, 2, 2, 4 ),
 ( 0.006298532399469917130, 0.01550158377817707420, 0.02010310946753066097, 0.02240387231220746303, 0.02470463515688426162, 0.03390768653559145251, 0.03850921222494505664, 0.04080997506962185523, 0.04311073791429865382, 0.05231378929300583430, 0.06151684067171302867, 0.06611836636106661891, 0.07071989205042020221, 0.07992294342912738270 ),
 .UNSPECIFIED. ) ;
#6522=CARTESIAN_POINT ( 'NONE',  ( 110.0212991616529052, 74.99906874937914836, 0.8747890471060546513 ) ) ;
#6531=DIRECTION ( 'NONE',  ( -0.01292414190464022741, 0.000000000000000000, -0.9999164797902017066 ) ) ;
#6542=DIRECTION ( 'NONE',  ( -0.01292414190464022741, 0.000000000000000000, -0.9999164797902017066 ) ) ;
#6551=CARTESIAN_POINT ( 'NONE',  ( 105.8297815006158515, 70.09865364193531434, 30.00121230636247560 ) ) ;
#6555=DIRECTION ( 'NONE',  ( -0.01292414190464131335, -1.902755938799530239E-22, -0.9999164797902015955 ) ) ;
#6556=DIRECTION ( 'NONE',  ( 0.9999164797902017066, 2.001050586450178931E-22, -0.01292414190464131508 ) ) ;
#6566=CARTESIAN_POINT ( 'NONE',  ( -90.12508629359015799, 87.39786947457938027, 51.15624717128011412 ) ) ;
#6569=DIRECTION ( 'NONE',  ( -2.025474946048326393E-22, 1.000000000000000000, -1.876735158486679873E-22 ) ) ;
#6574=CARTESIAN_POINT ( 'NONE',  ( -89.24856274066354445, 79.52628152566919084, 30.13108863562646533 ) ) ;
#6577=TOROIDAL_SURFACE ( 'NONE', #16152, 4.000000000000000000, 2.000000000000000000 ) ;
#6578=FACE_OUTER_BOUND ( 'NONE', #4728, .T. ) ;
#6581=DIRECTION ( 'NONE',  ( -2.025474946048326158E-22, 1.000000000000000000, -1.876735158486678933E-22 ) ) ;
#6587=ORIENTED_EDGE ( 'NONE', *, *, #4476, .T. ) ;
#6594=ORIENTED_EDGE ( 'NONE', *, *, #12021, .T. ) ;
#6597=CARTESIAN_POINT ( 'NONE',  ( -90.04153719330230388, 72.97786998644573941, 61.59291218184642247 ) ) ;
#6603=DIRECTION ( 'NONE',  ( 0.9999164797902017066, -5.258378535504111633E-16, -0.01292414190464131508 ) ) ;
#6607=EDGE_CURVE ( 'NONE', #18705, #4456, #1871, .T. ) ;
#6608=EDGE_LOOP ( 'NONE', ( #11250, #13311, #13790 ) ) ;
#6611=CIRCLE ( 'NONE', #10645, 1.999999999999997780 ) ;
#6627=VECTOR ( 'NONE', #14447, 1000.000000000000114 ) ;
#6632=VERTEX_POINT ( 'NONE', #18693 ) ;
#6649=CARTESIAN_POINT ( 'NONE',  ( -38.82295403925314758, 92.04141378167194887, 85.46747784716957597 ) ) ;
#6652=DIRECTION ( 'NONE',  ( -0.01292414190463827932, 0.000000000000000000, -0.9999164797902018176 ) ) ;
#6656=LINE ( 'NONE', #5144, #3147 ) ;
#6661=ORIENTED_EDGE ( 'NONE', *, *, #13297, .F. ) ;
#6668=AXIS2_PLACEMENT_3D ( 'NONE', #8832, #8605, #14383 ) ;
#6676=CARTESIAN_POINT ( 'NONE',  ( -90.11849266230689182, 87.42215604950109764, 51.14142411453754278 ) ) ;
#6681=ADVANCED_FACE ( 'NONE', ( #12903 ), #11171, .T. ) ;
#6683=CARTESIAN_POINT ( 'NONE',  ( -33.37547251039675444, 92.26055912610783594, -80.91241141183517982 ) ) ;
#6686=CARTESIAN_POINT ( 'NONE',  ( -88.16245334966984615, 88.15582427846244684, 52.99867833143289886 ) ) ;
#6691=ORIENTED_EDGE ( 'NONE', *, *, #8691, .T. ) ;
#6695=CARTESIAN_POINT ( 'NONE',  ( -73.00030478232707765, 95.66452290628956234, 82.28581592040848136 ) ) ;
#6696=CARTESIAN_POINT ( 'NONE',  ( 92.46788464407293873, 79.04398536104962147, -28.62013883513330015 ) ) ;
#6704=EDGE_CURVE ( 'NONE', #9279, #20198, #1146, .T. ) ;
#6713=CARTESIAN_POINT ( 'NONE',  ( 79.25753170385351609, 75.13519840835958519, -6.091774775480104154 ) ) ;
#6714=DIRECTION ( 'NONE',  ( 0.9999164797902015955, 2.001050586450178695E-22, -0.01292414190464131335 ) ) ;
#6715=CARTESIAN_POINT ( 'NONE',  ( 105.4775731789987105, 77.90269639574793814, -31.21677525025643263 ) ) ;
#6716=CARTESIAN_POINT ( 'NONE',  ( -92.79593043952057485, 70.16589065052623653, -59.06731773122654516 ) ) ;
#6719=ORIENTED_EDGE ( 'NONE', *, *, #19606, .F. ) ;
#6723=CARTESIAN_POINT ( 'NONE',  ( -64.14035809025482138, 91.69347899441576999, 66.92892513032199986 ) ) ;
#6725=CARTESIAN_POINT ( 'NONE',  ( 90.42410873942372973, 78.25489917908669213, -32.91867509261376057 ) ) ;
#6727=FACE_OUTER_BOUND ( 'NONE', #20726, .T. ) ;
#6728=FACE_OUTER_BOUND ( 'NONE', #12729, .T. ) ;
#6730=FACE_OUTER_BOUND ( 'NONE', #2509, .T. ) ;
#6733=AXIS2_PLACEMENT_3D ( 'NONE', #3840, #1888, #12240 ) ;
#6735=CARTESIAN_POINT ( 'NONE',  ( 39.36913080622081651, 72.00000000000000000, -87.51612159803863733 ) ) ;
#6742=VECTOR ( 'NONE', #15870, 1000.000000000000000 ) ;
#6745=ORIENTED_EDGE ( 'NONE', *, *, #5425, .T. ) ;
#6746=CYLINDRICAL_SURFACE ( 'NONE', #2251, 2.000000000000001332 ) ;
#6753=ORIENTED_EDGE ( 'NONE', *, *, #20902, .F. ) ;
#6764=EDGE_CURVE ( 'NONE', #9560, #18446, #17108, .T. ) ;
#6765=LINE ( 'NONE', #13787, #1150 ) ;
#6766=CARTESIAN_POINT ( 'NONE',  ( 1.247179693797900502, 44.99899999999999523, 96.49194029975444664 ) ) ;
#6770=ORIENTED_EDGE ( 'NONE', *, *, #11799, .F. ) ;
#6771=CARTESIAN_POINT ( 'NONE',  ( -90.07495684815179970, 87.56539372961334777, 51.05391499655451781 ) ) ;
#6773=DIRECTION ( 'NONE',  ( 0.9999164797902015955, 0.000000000000000000, -0.01292414190464174703 ) ) ;
#6775=CARTESIAN_POINT ( 'NONE',  ( -35.95309506732429128, 93.50464841319750064, -82.03286182426641915 ) ) ;
#6782=EDGE_LOOP ( 'NONE', ( #10003, #13943, #12443, #3107 ) ) ;
#6784=CARTESIAN_POINT ( 'NONE',  ( -90.02674258212728375, 88.67875473957917620, 52.55243696673224463 ) ) ;
#6798=ORIENTED_EDGE ( 'NONE', *, *, #18266, .F. ) ;
#6804=CYLINDRICAL_SURFACE ( 'NONE', #12135, 2.000000000000004441 ) ;
#6821=ADVANCED_FACE ( 'NONE', ( #17560 ), #6746, .F. ) ;
#6822=CYLINDRICAL_SURFACE ( 'NONE', #14459, 2.000000000000004885 ) ;
#6832=EDGE_CURVE ( 'NONE', #13967, #15481, #22436, .T. ) ;
#6834=LINE ( 'NONE', #13640, #12882 ) ;
#6836=CARTESIAN_POINT ( 'NONE',  ( -91.32251664931386870, 80.22595383786651269, -29.89762933574914783 ) ) ;
#6837=ORIENTED_EDGE ( 'NONE', *, *, #18087, .F. ) ;
#6840=CARTESIAN_POINT ( 'NONE',  ( 1.163172771417732010, 44.99899999999999523, 89.99248318111813205 ) ) ;
#6842=CARTESIAN_POINT ( 'NONE',  ( -104.8611102782643485, 69.99999999999998579, 33.22898942131119071 ) ) ;
#6850=CARTESIAN_POINT ( 'NONE',  ( 109.9781218937930589, 75.08416348859606160, 3.222660468417843482 ) ) ;
#6852=VERTEX_POINT ( 'NONE', #8795 ) ;
#6854=CARTESIAN_POINT ( 'NONE',  ( -91.73057767193260759, 77.20311952920093290, 31.31041951043025406 ) ) ;
#6863=DIRECTION ( 'NONE',  ( 0.9999164797902017066, 2.001050586450180576E-22, -0.01292414190464044946 ) ) ;
#6867=CARTESIAN_POINT ( 'NONE',  ( -37.28121903586303887, 92.86731729159741633, 84.62157808538474058 ) ) ;
#6879=DIRECTION ( 'NONE',  ( -0.01292414190464131335, -1.902755938799530239E-22, -0.9999164797902015955 ) ) ;
#6881=CYLINDRICAL_SURFACE ( 'NONE', #2993, 2.000000000000004885 ) ;
#6882=AXIS2_PLACEMENT_3D ( 'NONE', #7228, #14256, #12529 ) ;
#6883=VERTEX_POINT ( 'NONE', #22561 ) ;
#6886=ORIENTED_EDGE ( 'NONE', *, *, #15184, .T. ) ;
#6888=EDGE_CURVE ( 'NONE', #5416, #13498, #20864, .T. ) ;
#6893=CARTESIAN_POINT ( 'NONE',  ( -88.16993261600009646, 88.76241539977888806, 52.31541104021305699 ) ) ;
#6894=LINE ( 'NONE', #13916, #3080 ) ;
#6900=B_SPLINE_CURVE_WITH_KNOTS ( 'NONE', 3,
 ( #9350, #16388, #11200, #6129, #6020, #5898, #12934, #21839, #2459, #13056, #13270, #11542 ),
 .UNSPECIFIED., .F., .F.,
 ( 4, 2, 2, 2, 2, 4 ),
 ( 0.04309441970742561301, 0.05230155063785107278, 0.06150868156827653255, 0.06611224703348925202, 0.07071581249870198538, 0.07992294342912742433 ),
 .UNSPECIFIED. ) ;
#6902=CARTESIAN_POINT ( 'NONE',  ( -30.68998116395940912, 91.18377996386419682, -79.89680297002404075 ) ) ;
#6904=CARTESIAN_POINT ( 'NONE',  ( 82.49079974960680772, 75.10299918630330751, -5.493043209074147448 ) ) ;
#6906=ORIENTED_EDGE ( 'NONE', *, *, #18154, .F. ) ;
#6914=CARTESIAN_POINT ( 'NONE',  ( -92.46042328379806463, 77.12912189496637438, 29.19741020490883088 ) ) ;
#6915=VECTOR ( 'NONE', #18966, 1000.000000000000000 ) ;
#6916=LINE ( 'NONE', #13937, #15976 ) ;
#6930=CARTESIAN_POINT ( 'NONE',  ( 1.364375150383346228E-14, 45.00000000000000000, -9.836439021161248541E-15 ) ) ;
#6931=CARTESIAN_POINT ( 'NONE',  ( -89.94862617306016261, 81.58347563513834189, 79.55911641354585129 ) ) ;
#6942=ORIENTED_EDGE ( 'NONE', *, *, #19791, .F. ) ;
#6946=EDGE_CURVE ( 'NONE', #2340, #10951, #14474, .T. ) ;
#6947=CARTESIAN_POINT ( 'NONE',  ( -72.65963751957909267, 87.42236182341126494, 69.77244766351077487 ) ) ;
#6951=FACE_OUTER_BOUND ( 'NONE', #5315, .T. ) ;
#6958=ORIENTED_EDGE ( 'NONE', *, *, #17625, .F. ) ;
#6959=VERTEX_POINT ( 'NONE', #18019 ) ;
#6965=CARTESIAN_POINT ( 'NONE',  ( 106.1636641531657972, 79.04398536104962147, -28.79715981783310497 ) ) ;
#6966=AXIS2_PLACEMENT_3D ( 'NONE', #6287, #11573, #9623 ) ;
#6970=ORIENTED_EDGE ( 'NONE', *, *, #22112, .F. ) ;
#6971=CARTESIAN_POINT ( 'NONE',  ( -91.12451015595505055, 77.41163679146356458, 31.64200013680033052 ) ) ;
#6985=LINE ( 'NONE', #4921, #1602 ) ;
#7015=CARTESIAN_POINT ( 'NONE',  ( -90.02889123584817810, 87.66185544671367325, 50.99467065406356880 ) ) ;
#7019=ORIENTED_EDGE ( 'NONE', *, *, #5108, .T. ) ;
#7022=CARTESIAN_POINT ( 'NONE',  ( -36.55288090549052527, 94.02752048664899576, 83.45186405039063970 ) ) ;
#7025=CARTESIAN_POINT ( 'NONE',  ( 82.19586818426773789, 75.11053174630316676, -5.645930764600690210 ) ) ;
#7032=CARTESIAN_POINT ( 'NONE',  ( -78.73812145396803430, 75.12795917139310120, -3.912027923891130410 ) ) ;
#7034=VECTOR ( 'NONE', #15172, 1000.000000000000000 ) ;
#7038=CARTESIAN_POINT ( 'NONE',  ( -36.36981320942769003, 93.68077895625195595, -82.19051798928661867 ) ) ;
#7052=LINE ( 'NONE', #15581, #4531 ) ;
#7054=DIRECTION ( 'NONE',  ( 0.01292414190464131508, 0.000000000000000000, 0.9999164797902017066 ) ) ;
#7055=CIRCLE ( 'NONE', #12951, 5.099999999999994316 ) ;
#7059=CARTESIAN_POINT ( 'NONE',  ( 92.35175351209242933, 79.88298967448075416, 28.93780754488613738 ) ) ;
#7064=DIRECTION ( 'NONE',  ( -2.459148776293844314E-24, 1.000000000000000000, -1.902597020224326827E-22 ) ) ;
#7067=CARTESIAN_POINT ( 'NONE',  ( -93.17671387018313567, 79.04398536104955042, -26.22064129356662576 ) ) ;
#7078=DIRECTION ( 'NONE',  ( 0.01292414190464131335, 0.000000000000000000, 0.9999164797902017066 ) ) ;
#7083=EDGE_CURVE ( 'NONE', #16665, #13967, #14813, .T. ) ;
#7084=CARTESIAN_POINT ( 'NONE',  ( 71.26616241777607286, 92.22173151023523019, 83.79227730723269474 ) ) ;
#7094=VECTOR ( 'NONE', #10827, 1000.000000000000000 ) ;
#7095=CIRCLE ( 'NONE', #20666, 83.00000000000002842 ) ;
#7106=FACE_OUTER_BOUND ( 'NONE', #13010, .T. ) ;
#7112=EDGE_CURVE ( 'NONE', #10097, #14863, #20192, .T. ) ;
#7114=LINE ( 'NONE', #1613, #6742 ) ;
#7116=EDGE_CURVE ( 'NONE', #16665, #9075, #22413, .T. ) ;
#7118=ORIENTED_EDGE ( 'NONE', *, *, #21603, .T. ) ;
#7124=CARTESIAN_POINT ( 'NONE',  ( 84.85051924643074983, 104.5953608974804467, -70.00327014827948346 ) ) ;
#7130=VERTEX_POINT ( 'NONE', #9220 ) ;
#7134=CARTESIAN_POINT ( 'NONE',  ( -89.62788137478739259, 89.06476581229102862, 51.83667496493544746 ) ) ;
#7135=ADVANCED_FACE ( 'NONE', ( #11191 ), #9341, .T. ) ;
#7141=CARTESIAN_POINT ( 'NONE',  ( 81.73018904534613682, 75.12006735377336497, -5.831974844687870529 ) ) ;
#7149=CARTESIAN_POINT ( 'NONE',  ( 92.43457499998882554, 72.00000000000000000, -31.19724316448930423 ) ) ;
#7150=CARTESIAN_POINT ( 'NONE',  ( -78.41642969337061686, 75.12296263580977040, -3.819052735123477316 ) ) ;
#7162=EDGE_LOOP ( 'NONE', ( #2994, #586, #21540, #2709 ) ) ;
#7172=CARTESIAN_POINT ( 'NONE',  ( 38.46706438352715196, 72.00000000000000000, -85.27439087629288395 ) ) ;
#7177=CARTESIAN_POINT ( 'NONE',  ( 92.30767208729216122, 77.25770192717985196, 29.02102379856335901 ) ) ;
#7178=CARTESIAN_POINT ( 'NONE',  ( 92.90824731599337838, 79.04398536104963569, 26.22411128322410789 ) ) ;
#7179=ORIENTED_EDGE ( 'NONE', *, *, #8950, .T. ) ;
#7183=DIRECTION ( 'NONE',  ( -2.025474946048326393E-22, 1.000000000000000000, -1.876735158486679873E-22 ) ) ;
#7185=EDGE_CURVE ( 'NONE', #5449, #567, #7271, .T. ) ;
#7191=DIRECTION ( 'NONE',  ( -2.025474946048326158E-22, 1.000000000000000000, -1.876735158486678933E-22 ) ) ;
#7197=DIRECTION ( 'NONE',  ( 0.01292414190464174703, 0.000000000000000000, 0.9999164797902015955 ) ) ;
#7200=CARTESIAN_POINT ( 'NONE',  ( -91.52572433156647946, 77.25800443875652945, 31.39760542763772477 ) ) ;
#7202=VERTEX_POINT ( 'NONE', #21606 ) ;
#7212=EDGE_CURVE ( 'NONE', #16639, #10904, #16931, .T. ) ;
#7213=DIRECTION ( 'NONE',  ( 0.4768814951561130555, 0.000000000000000000, 0.8789675987075236119 ) ) ;
#7215=CARTESIAN_POINT ( 'NONE',  ( 36.73936676148917968, 94.93197183469658285, 81.60001862646660697 ) ) ;
#7220=ORIENTED_EDGE ( 'NONE', *, *, #19213, .T. ) ;
#7221=CARTESIAN_POINT ( 'NONE',  ( 89.71146001588847696, 97.21218566216820989, -63.65427843874460478 ) ) ;
#7224=ORIENTED_EDGE ( 'NONE', *, *, #21978, .T. ) ;
#7225=DIRECTION ( 'NONE',  ( -2.025474946048326158E-22, 1.000000000000000000, -1.876735158486679638E-22 ) ) ;
#7228=CARTESIAN_POINT ( 'NONE',  ( -88.82263333796718996, 169.9999999999999716, 1.148052203164670715 ) ) ;
#7232=CARTESIAN_POINT ( 'NONE',  ( 38.21725127624093687, 94.02752048664899576, 82.48544353620104630 ) ) ;
#7235=ADVANCED_FACE ( 'NONE', ( #7952 ), #12810, .T. ) ;
#7236=CARTESIAN_POINT ( 'NONE',  ( 90.02055463237803679, 72.00000000000000000, -63.21629334023821656 ) ) ;
#7237=CARTESIAN_POINT ( 'NONE',  ( -89.91512339040338020, 88.85449468744033652, 52.31052459259786502 ) ) ;
#7241=CARTESIAN_POINT ( 'NONE',  ( -92.43457499998879712, 79.86121811340019860, 31.19724316448926160 ) ) ;
#7243=CARTESIAN_POINT ( 'NONE',  ( 81.57020707306168106, 75.12296263580984146, -5.886915439866140076 ) ) ;
#7249=VERTEX_POINT ( 'NONE', #21936 ) ;
#7255=ORIENTED_EDGE ( 'NONE', *, *, #6263, .T. ) ;
#7269=VERTEX_POINT ( 'NONE', #15222 ) ;
#7271=LINE ( 'NONE', #507, #19496 ) ;
#7279=CARTESIAN_POINT ( 'NONE',  ( 83.75728585524183245, 104.6157580258879136, 71.30770656078364311 ) ) ;
#7280=CARTESIAN_POINT ( 'NONE',  ( -83.75728585524177561, 104.6157580258879278, -71.30770656078371417 ) ) ;
#7292=CARTESIAN_POINT ( 'NONE',  ( -39.40254987707573520, 92.58578643762697880, 84.93055112583743949 ) ) ;
#7301=CIRCLE ( 'NONE', #13199, 109.9999999999999858 ) ;
#7303=CARTESIAN_POINT ( 'NONE',  ( 66.45999312048357410, 69.99999999999998579, -87.65380681892989401 ) ) ;
#7308=CARTESIAN_POINT ( 'NONE',  ( -92.16545979397227484, 77.13735158510579026, 31.20743466190297610 ) ) ;
#7316=VERTEX_POINT ( 'NONE', #13817 ) ;
#7318=COLOUR_RGB ( '', 0.31764706, 0.68627451, 0.89019608) ;
#7328=CARTESIAN_POINT ( 'NONE',  ( -65.63430937367742501, 90.62871777570580889, 67.04661370716345914 ) ) ;
#7331=DIRECTION ( 'NONE',  ( -2.025474946048326158E-22, 1.000000000000000000, -1.876735158486679638E-22 ) ) ;
#7337=AXIS2_PLACEMENT_3D ( 'NONE', #12243, #21070, #17525 ) ;
#7340=CARTESIAN_POINT ( 'NONE',  ( 36.81267581808855738, 93.81198433751869459, 82.30576130133127322 ) ) ;
#7345=CARTESIAN_POINT ( 'NONE',  ( -89.67433851549336055, 89.04342406756380512, 51.90552969022834873 ) ) ;
#7346=AXIS2_PLACEMENT_3D ( 'NONE', #22407, #9081, #14062 ) ;
#7352=( BOUNDED_CURVE ( )  B_SPLINE_CURVE ( 3, ( #10840, #8738, #17866, #19211 ),
 .UNSPECIFIED., .F., .T. ) 
 B_SPLINE_CURVE_WITH_KNOTS ( ( 4, 4 ),
 ( 5.799006443144740786, 5.860216683781459324 ),
 .UNSPECIFIED. ) 
 CURVE ( )  GEOMETRIC_REPRESENTATION_ITEM ( )  RATIONAL_B_SPLINE_CURVE ( ( 1.000000000000000000, 0.9996877999070342691, 0.9996877999070342691, 1.000000000000000000 ) ) 
 REPRESENTATION_ITEM ( '' )  );
#7353=DIRECTION ( 'NONE',  ( 0.01220060921879500236, -0.3298969072164960603, 0.9439381207174974975 ) ) ;
#7356=EDGE_CURVE ( 'NONE', #12, #7696, #20481, .T. ) ;
#7364=CARTESIAN_POINT ( 'NONE',  ( -78.28836335706589011, 75.12327740397419973, 5.852126302717420181 ) ) ;
#7368=VERTEX_POINT ( 'NONE', #22392 ) ;
#7376=AXIS2_PLACEMENT_3D ( 'NONE', #22067, #4390, #20248 ) ;
#7387=B_SPLINE_CURVE_WITH_KNOTS ( 'NONE', 3,
 ( #15963, #2035, #10985, #7084, #7547, #21093, #21202, #86, #10878, #3523 ),
 .UNSPECIFIED., .F., .F.,
 ( 4, 2, 2, 2, 4 ),
 ( 5.721958498152796815E-17, 0.0004376694309007161097, 0.0008753388618013749735, 0.001313008292702033892, 0.001750677723602692701 ),
 .UNSPECIFIED. ) ;
#7388=CARTESIAN_POINT ( 'NONE',  ( -91.14933227754934819, 79.20679280668173305, -26.78161688013030428 ) ) ;
#7396=CARTESIAN_POINT ( 'NONE',  ( 89.70716773419727019, 79.66972452536271021, 28.26220109401201341 ) ) ;
#7398=B_SPLINE_CURVE_WITH_KNOTS ( 'NONE', 3,
 ( #5962, #7683, #1964, #7340, #19521, #3792, #7232, #8953 ),
 .UNSPECIFIED., .F., .F.,
 ( 4, 2, 2, 4 ),
 ( 0.000000000000000000, 0.0007138554872576933965, 0.001427710974515386793, 0.002855421949030781392 ),
 .UNSPECIFIED. ) ;
#7399=ADVANCED_FACE ( 'NONE', ( #18858 ), #3466, .F. ) ;
#7400=CARTESIAN_POINT ( 'NONE',  ( 89.22440607450265304, 80.22990097357060790, 29.93634654116225846 ) ) ;
#7404=EDGE_CURVE ( 'NONE', #7269, #4506, #20800, .T. ) ;
#7405=DIRECTION ( 'NONE',  ( -0.9999164797902017066, -2.001050586450178931E-22, 0.01292414190464131508 ) ) ;
#7408=B_SPLINE_CURVE_WITH_KNOTS ( 'NONE', 3,
 ( #21146, #10583, #142, #17261, #19311, #7243, #7141, #7025, #6904, #13924, #20916, #1530, #5174, #8622, #8725, #1857, #8513, #21037, #10484, #5392, #19081, #12215, #15665, #22608, #19199, #3470, #12431, #18965, #19, #1747, #19419, #15554, #3681, #15778, #14053, #10702, #8968, #17731, #1977, #22503 ),
 .UNSPECIFIED., .F., .F.,
 ( 4, 2, 2, 2, 2, 2, 2, 2, 2, 2, 2, 2, 2, 2, 2, 2, 2, 2, 2, 4 ),
 ( 0.000000000000000000, 0.0009967370484891076212, 0.001495105572733641157, 0.001993474096978174476, 0.002990211145467242416, 0.003986948193956310789, 0.004983685242445377861, 0.005980422290934445800, 0.006977159339423513740, 0.007973896387912581679, 0.008970633436401647884, 0.009967370484890715823, 0.01046573900913524979, 0.01096410753337978376, 0.01196084458186887599, 0.01295758163035796821, 0.01345595015460251606, 0.01395431867884706217, 0.01495105572733619256, 0.01594779277582532295 ),
 .UNSPECIFIED. ) ;
#7409=AXIS2_PLACEMENT_3D ( 'NONE', #13289, #16509, #886 ) ;
#7417=CARTESIAN_POINT ( 'NONE',  ( -64.14341903774379716, 91.03664218477042880, 66.69210539709879981 ) ) ;
#7428=CARTESIAN_POINT ( 'NONE',  ( 68.01573619543682980, 70.58429683895612072, -86.45204278734176739 ) ) ;
#7430=CARTESIAN_POINT ( 'NONE',  ( -92.02635692360499320, 79.83422912033660168, 31.21470397902808358 ) ) ;
#7436=AXIS2_PLACEMENT_3D ( 'NONE', #9037, #12639, #7565 ) ;
#7441=VERTEX_POINT ( 'NONE', #10140 ) ;
#7449=LINE ( 'NONE', #21451, #21721 ) ;
#7462=LINE ( 'NONE', #19842, #8860 ) ;
#7470=CARTESIAN_POINT ( 'NONE',  ( -88.17056478026623267, 88.79561276468949416, 52.25202260040794755 ) ) ;
#7474=ORIENTED_EDGE ( 'NONE', *, *, #240, .F. ) ;
#7477=ORIENTED_EDGE ( 'NONE', *, *, #772, .T. ) ;
#7480=ORIENTED_EDGE ( 'NONE', *, *, #510, .F. ) ;
#7483=CARTESIAN_POINT ( 'NONE',  ( -91.10494378670937010, 97.90071567704920596, -61.64404307423189522 ) ) ;
#7497=FACE_OUTER_BOUND ( 'NONE', #3986, .T. ) ;
#7499=AXIS2_PLACEMENT_3D ( 'NONE', #21112, #19383, #3649 ) ;
#7501=B_SPLINE_CURVE_WITH_KNOTS ( 'NONE', 3,
 ( #14745, #943, #7590, #9191, #482, #14625, #7483, #14516, #21477, #21578, #21698, #3412 ),
 .UNSPECIFIED., .F., .F.,
 ( 4, 2, 2, 2, 2, 4 ),
 ( 0.000000000000000000, 0.0007983727002588498134, 0.001596745400517699627, 0.003193490801035416167, 0.004790236201553133358, 0.006386981602070849681 ),
 .UNSPECIFIED. ) ;
#7502=CARTESIAN_POINT ( 'NONE',  ( 66.06691928577360784, 94.02752048664899576, 82.12548041065294058 ) ) ;
#7506=CARTESIAN_POINT ( 'NONE',  ( -105.0923722050658426, 70.19488773545516835, 32.49013605942701588 ) ) ;
#7508=( BOUNDED_CURVE ( )  B_SPLINE_CURVE ( 3, ( #19796, #4071, #885, #4188 ),
 .UNSPECIFIED., .F., .T. ) 
 B_SPLINE_CURVE_WITH_KNOTS ( ( 4, 4 ),
 ( 0.4472747960204460083, 0.4841788640348455020 ),
 .UNSPECIFIED. ) 
 CURVE ( )  GEOMETRIC_REPRESENTATION_ITEM ( )  RATIONAL_B_SPLINE_CURVE ( ( 1.000000000000000000, 0.9998865107004337727, 0.9998865107004337727, 1.000000000000000000 ) ) 
 REPRESENTATION_ITEM ( '' )  );
#7511=DIRECTION ( 'NONE',  ( -0.01292414190464131335, -1.902755938799530239E-22, -0.9999164797902015955 ) ) ;
#7519=CARTESIAN_POINT ( 'NONE',  ( 91.69446324238793977, 77.56197482480291683, 29.51646066538733493 ) ) ;
#7523=CARTESIAN_POINT ( 'NONE',  ( 91.51031840793916672, 96.48503848149371720, 61.03988419336475602 ) ) ;
#7525=EDGE_CURVE ( 'NONE', #15481, #12773, #15138, .T. ) ;
#7529=DIRECTION ( 'NONE',  ( 0.9999164797902015955, 2.001050586450180341E-22, -0.01292414190464038874 ) ) ;
#7533=CARTESIAN_POINT ( 'NONE',  ( -37.51181209962059881, 93.56461422141713058, 83.92720337889271320 ) ) ;
#7539=DIRECTION ( 'NONE',  ( -0.9999164797902017066, -2.001050586450178931E-22, 0.01292414190464131508 ) ) ;
#7547=CARTESIAN_POINT ( 'NONE',  ( 71.18985671402978710, 92.11167198312701032, 83.85708946072357151 ) ) ;
#7549=CARTESIAN_POINT ( 'NONE',  ( -91.77247882320317274, 77.19421037201389879, 31.29629296514997705 ) ) ;
#7550=DIRECTION ( 'NONE',  ( -0.009138748381789078140, 0.7071067811865487940, -0.7070477234798315802 ) ) ;
#7556=ORIENTED_EDGE ( 'NONE', *, *, #5824, .T. ) ;
#7565=DIRECTION ( 'NONE',  ( -6.938893903907222067E-15, -1.000000000000000000, 0.000000000000000000 ) ) ;
#7571=CARTESIAN_POINT ( 'NONE',  ( -64.14035809025482138, 91.69347899441576999, 66.92892513032199986 ) ) ;
#7575=CARTESIAN_POINT ( 'NONE',  ( 25.08966747280857845, 89.38128957862194568, 78.14996769037233548 ) ) ;
#7581=CARTESIAN_POINT ( 'NONE',  ( -89.08844981478657132, 89.10459688240003118, 51.16498045765563063 ) ) ;
#7589=CARTESIAN_POINT ( 'NONE',  ( -106.0703656581358416, 70.66226986180335246, -29.13909619158257769 ) ) ;
#7590=CARTESIAN_POINT ( 'NONE',  ( -91.59502366432084841, 95.97275144416944670, -60.91270374391781672 ) ) ;
#7591=ORIENTED_EDGE ( 'NONE', *, *, #1086, .T. ) ;
#7592=CARTESIAN_POINT ( 'NONE',  ( 93.21002351426729149, 77.12912189496647386, 28.79774562292276840 ) ) ;
#7595=CARTESIAN_POINT ( 'NONE',  ( -91.39645842968019451, 77.87428392844081770, -30.00278187767193927 ) ) ;
#7600=ADVANCED_FACE ( 'NONE', ( #3805 ), #14272, .T. ) ;
#7601=DIRECTION ( 'NONE',  ( 0.01292414190464177652, 1.902755938799532355E-22, 0.9999164797902015955 ) ) ;
#7605=VERTEX_POINT ( 'NONE', #10927 ) ;
#7606=DIRECTION ( 'NONE',  ( -0.9999164797902017066, -4.653667080246436871E-16, 0.01292414190464177999 ) ) ;
#7609=CARTESIAN_POINT ( 'NONE',  ( -90.11843179045052921, 88.40872791604708425, 52.82837235832041500 ) ) ;
#7610=ORIENTED_EDGE ( 'NONE', *, *, #14610, .F. ) ;
#7615=CARTESIAN_POINT ( 'NONE',  ( -90.15711184568681347, 79.46353706204938305, -27.61532001585845109 ) ) ;
#7616=CARTESIAN_POINT ( 'NONE',  ( 70.44022362938051174, 70.80424004364375890, 84.48783506240397401 ) ) ;
#7620=CARTESIAN_POINT ( 'NONE',  ( 92.63973831233896306, 79.05196971970121922, 26.25410855708543423 ) ) ;
#7621=CARTESIAN_POINT ( 'NONE',  ( -92.82229925712802299, 69.99999999999998579, 1.199748770783236385 ) ) ;
#7624=FACE_OUTER_BOUND ( 'NONE', #2379, .T. ) ;
#7630=CARTESIAN_POINT ( 'NONE',  ( 75.07439005099489293, 75.00866199770877074, 0.3533726697390237592 ) ) ;
#7631=CARTESIAN_POINT ( 'NONE',  ( -90.49431781703050603, 70.72571308208034679, 61.29990699711781588 ) ) ;
#7632=EDGE_LOOP ( 'NONE', ( #5022, #11471, #19064, #14426 ) ) ;
#7637=ORIENTED_EDGE ( 'NONE', *, *, #4152, .T. ) ;
#7644=DIRECTION ( 'NONE',  ( -2.025474946048326158E-22, 1.000000000000000000, -1.876735158486679638E-22 ) ) ;
#7645=DIRECTION ( 'NONE',  ( -2.459148776293844314E-24, 1.000000000000000000, -1.902597020224326827E-22 ) ) ;
#7657=B_SPLINE_CURVE_WITH_KNOTS ( 'NONE', 3,
 ( #11770, #15241, #20595, #10045, #6378, #18650, #15460, #13834, #2914, #4732, #22196, #22414, #20474, #3369, #10386, #1091 ),
 .UNSPECIFIED., .F., .F.,
 ( 4, 2, 2, 2, 2, 2, 2, 4 ),
 ( 0.000000000000000000, 0.0004288218673305856272, 0.0008576437346611712545, 0.001286465601991756882, 0.001715287469322342509, 0.002144109336652928136, 0.002572931203983513763, 0.003430574938644721447 ),
 .UNSPECIFIED. ) ;
#7661=EDGE_CURVE ( 'NONE', #18024, #6487, #13665, .T. ) ;
#7663=ORIENTED_EDGE ( 'NONE', *, *, #6175, .T. ) ;
#7669=B_SPLINE_CURVE_WITH_KNOTS ( 'NONE', 3,
 ( #15527, #15642, #8481, #22363, #6771, #4806, #17474, #3100, #1724, #1615, #17585, #4789, #22586, #3199, #13564, #8374 ),
 .UNSPECIFIED., .F., .F.,
 ( 4, 2, 2, 2, 2, 2, 2, 4 ),
 ( 6.691626947686431882E-17, 0.0003925140011974886174, 0.0007850280023949103396, 0.001177542003592332333, 0.001570056004789753892, 0.001962570005987175452, 0.002355084007184597445, 0.003140112009579444901 ),
 .UNSPECIFIED. ) ;
#7683=CARTESIAN_POINT ( 'NONE',  ( 36.15575925104655397, 93.60246426260026453, 82.12095663381342092 ) ) ;
#7687=AXIS2_PLACEMENT_3D ( 'NONE', #19033, #3767, #8461 ) ;
#7690=CARTESIAN_POINT ( 'NONE',  ( -93.23587179807654479, 72.00000000000000000, -30.79757858250321689 ) ) ;
#7691=CARTESIAN_POINT ( 'NONE',  ( -88.41179892586471567, 88.71926944898528689, 50.32451584197536221 ) ) ;
#7696=VERTEX_POINT ( 'NONE', #6331 ) ;
#7704=DIRECTION ( 'NONE',  ( -0.01292414190465215537, 0.000000000000000000, -0.9999164797902015955 ) ) ;
#7708=CARTESIAN_POINT ( 'NONE',  ( -72.65623182917823897, 87.80665977804258659, 70.23323934248251987 ) ) ;
#7719=DIRECTION ( 'NONE',  ( -0.01292414190464131508, 0.000000000000000000, -0.9999164797902017066 ) ) ;
#7720=VERTEX_POINT ( 'NONE', #2867 ) ;
#7725=CARTESIAN_POINT ( 'NONE',  ( -82.31274079517788778, 75.11017898543126137, -3.511195801982965214 ) ) ;
#7727=CARTESIAN_POINT ( 'NONE',  ( -90.13867034150928248, 88.25703757669403160, 52.94586342302623194 ) ) ;
#7735=DIRECTION ( 'NONE',  ( -0.01292414190464132896, 0.000000000000000000, -0.9999164797902015955 ) ) ;
#7737=CARTESIAN_POINT ( 'NONE',  ( -35.92446336679493157, 93.51775827232350480, -82.02042234242476582 ) ) ;
#7742=B_SPLINE_CURVE_WITH_KNOTS ( 'NONE', 3,
 ( #18669, #13419, #4541, #15262, #11569, #9618, #22212, #2828, #2934, #9953, #20494, #21756, #3694, #4875 ),
 .UNSPECIFIED., .F., .F.,
 ( 4, 2, 2, 2, 2, 2, 4 ),
 ( 0.000000000000000000, 0.001119727475084554861, 0.001679591212626828714, 0.002239454950169102784, 0.003359182425253666102, 0.003919046162795954483, 0.004478909900338241996 ),
 .UNSPECIFIED. ) ;
#7753=DIRECTION ( 'NONE',  ( -0.006350819331212799977, 0.8709385446395345731, -0.4913509118287983091 ) ) ;
#7756=EDGE_CURVE ( 'NONE', #13377, #3120, #4108, .T. ) ;
#7759=CARTESIAN_POINT ( 'NONE',  ( 77.38145957316694989, 75.10270664613308611, -5.417547979167955496 ) ) ;
#7766=CARTESIAN_POINT ( 'NONE',  ( -69.24448582912822303, 92.41827837429551096, 85.47053766693683485 ) ) ;
#7768=CARTESIAN_POINT ( 'NONE',  ( 89.11130500643436392, 98.76544454674674967, -64.49243618084513230 ) ) ;
#7770=CARTESIAN_POINT ( 'NONE',  ( 91.40469917791151033, 79.08369667522882196, -28.73783386972092302 ) ) ;
#7780=CIRCLE ( 'NONE', #2635, 110.0000000000000000 ) ;
#7781=VERTEX_POINT ( 'NONE', #14741 ) ;
#7782=CARTESIAN_POINT ( 'NONE',  ( -71.88056509240439595, 96.34227735399929315, 78.69877631277590524 ) ) ;
#7784=FACE_OUTER_BOUND ( 'NONE', #16108, .T. ) ;
#7785=CIRCLE ( 'NONE', #1563, 110.0000000000000000 ) ;
#7786=EDGE_CURVE ( 'NONE', #7720, #12921, #20427, .T. ) ;
#7790=LINE ( 'NONE', #11243, #5599 ) ;
#7791=DIRECTION ( 'NONE',  ( 0.01292414190464131508, 0.000000000000000000, 0.9999164797902017066 ) ) ;
#7792=ORIENTED_EDGE ( 'NONE', *, *, #11262, .T. ) ;
#7795=ORIENTED_EDGE ( 'NONE', *, *, #5316, .F. ) ;
#7813=CARTESIAN_POINT ( 'NONE',  ( -89.57008079183799509, 88.24871054370684931, 50.63090528479802543 ) ) ;
#7824=EDGE_CURVE ( 'NONE', #12220, #19868, #16790, .T. ) ;
#7832=FACE_OUTER_BOUND ( 'NONE', #18394, .T. ) ;
#7835=EDGE_CURVE ( 'NONE', #19083, #13764, #7055, .T. ) ;
#7841=EDGE_LOOP ( 'NONE', ( #5258, #733, #4558, #602 ) ) ;
#7842=DIRECTION ( 'NONE',  ( -0.9999164797902015955, -2.001050586450178695E-22, 0.01292414190464131335 ) ) ;
#7849=CARTESIAN_POINT ( 'NONE',  ( -105.2816027134186641, 70.66149885336977832, 31.87151722101068430 ) ) ;
#7853=CARTESIAN_POINT ( 'NONE',  ( -71.57228119427200852, 96.47114962407205496, 78.56582497698298084 ) ) ;
#7863=LINE ( 'NONE', #7621, #21991 ) ;
#7869=FACE_OUTER_BOUND ( 'NONE', #2872, .T. ) ;
#7870=ORIENTED_EDGE ( 'NONE', *, *, #21564, .F. ) ;
#7872=CIRCLE ( 'NONE', #7376, 110.0000000000000000 ) ;
#7873=CIRCLE ( 'NONE', #10091, 2.000000000000004885 ) ;
#7885=CARTESIAN_POINT ( 'NONE',  ( 91.23603883849617091, 78.43035437438882695, 30.82342686631245243 ) ) ;
#7887=PLANE ( 'NONE',  #21352 ) ;
#7891=FACE_OUTER_BOUND ( 'NONE', #16841, .T. ) ;
#7907=DIRECTION ( 'NONE',  ( -2.025474946048326158E-22, 1.000000000000000000, -1.876735158486679638E-22 ) ) ;
#7910=VECTOR ( 'NONE', #16791, 1000.000000000000114 ) ;
#7911=CARTESIAN_POINT ( 'NONE',  ( -23.03918042842984804, 89.37478006253336105, 78.76536267817510861 ) ) ;
#7925=CARTESIAN_POINT ( 'NONE',  ( 90.50186546057696546, 78.02565673216736286, -32.58161589089097276 ) ) ;
#7929=EDGE_LOOP ( 'NONE', ( #8164, #1883, #17926, #20619 ) ) ;
#7931=CARTESIAN_POINT ( 'NONE',  ( 68.81222610332000045, 91.74143318381845802, -85.81887827424428394 ) ) ;
#7932=ORIENTED_EDGE ( 'NONE', *, *, #20290, .F. ) ;
#7935=CARTESIAN_POINT ( 'NONE',  ( 41.56623493000984126, 91.17157287525387233, 82.46967996629570052 ) ) ;
#7936=CYLINDRICAL_SURFACE ( 'NONE', #15576, 2.000000000000004441 ) ;
#7943=EDGE_LOOP ( 'NONE', ( #21826, #8028, #1777, #8438 ) ) ;
#7946=ORIENTED_EDGE ( 'NONE', *, *, #10260, .F. ) ;
#7948=CARTESIAN_POINT ( 'NONE',  ( -90.14671295017259922, 88.16084041142528349, 53.01462269988137876 ) ) ;
#7950=EDGE_CURVE ( 'NONE', #19868, #7605, #847, .T. ) ;
#7952=FACE_OUTER_BOUND ( 'NONE', #878, .T. ) ;
#7962=CARTESIAN_POINT ( 'NONE',  ( -40.65822637310711940, 72.00000000000000000, -84.25167897319539634 ) ) ;
#7967=ORIENTED_EDGE ( 'NONE', *, *, #9347, .T. ) ;
#7970=ORIENTED_EDGE ( 'NONE', *, *, #5411, .T. ) ;
#7974=CARTESIAN_POINT ( 'NONE',  ( 75.89440375158403640, 75.05036917497849913, -4.086763113510438750 ) ) ;
#7976=CARTESIAN_POINT ( 'NONE',  ( -106.7514472241618932, 78.38843585434905492, 26.63023763040591163 ) ) ;
#7978=EDGE_CURVE ( 'NONE', #21811, #9274, #10339, .T. ) ;
#7985=CARTESIAN_POINT ( 'NONE',  ( 91.18542874977053714, 79.95750479416805945, -31.50072335808802038 ) ) ;
#8001=ORIENTED_EDGE ( 'NONE', *, *, #15989, .F. ) ;
#8006=ORIENTED_EDGE ( 'NONE', *, *, #11604, .T. ) ;
#8013=CARTESIAN_POINT ( 'NONE',  ( -106.2491592972476155, 77.90302844854605269, -28.48020057081445344 ) ) ;
#8019=ORIENTED_EDGE ( 'NONE', *, *, #8083, .T. ) ;
#8020=DIRECTION ( 'NONE',  ( 0.01292414190464131335, 0.000000000000000000, 0.9999164797902017066 ) ) ;
#8023=DIRECTION ( 'NONE',  ( -0.01292414190464137060, 0.000000000000000000, -0.9999164797902015955 ) ) ;
#8028=ORIENTED_EDGE ( 'NONE', *, *, #13450, .F. ) ;
#8030=ADVANCED_FACE ( 'NONE', ( #2053 ), #453, .F. ) ;
#8031=DIRECTION ( 'NONE',  ( 0.9999164797902015955, 4.653667080246434899E-16, -0.01292414190464084844 ) ) ;
#8035=CARTESIAN_POINT ( 'NONE',  ( -41.56623493000981284, 69.99999999999998579, -82.46967996629571473 ) ) ;
#8040=ORIENTED_EDGE ( 'NONE', *, *, #10175, .T. ) ;
#8043=CARTESIAN_POINT ( 'NONE',  ( 69.43142427201327394, 92.58578643762697880, -85.31868097644085935 ) ) ;
#8055=CARTESIAN_POINT ( 'NONE',  ( -90.17005756999139976, 87.12416931164095502, 51.32274856367679661 ) ) ;
#8058=EDGE_CURVE ( 'NONE', #959, #9371, #17350, .T. ) ;
#8064=EDGE_LOOP ( 'NONE', ( #334, #9113, #11892, #21360, #469, #9337, #2020, #3806, #12631, #4590, #1756, #6081, #6198, #1668, #22255 ) ) ;
#8067=CARTESIAN_POINT ( 'NONE',  ( -88.18706637290659955, 88.71869973106718987, 50.32066939225188662 ) ) ;
#8071=ORIENTED_EDGE ( 'NONE', *, *, #6946, .F. ) ;
#8080=VECTOR ( 'NONE', #13632, 1000.000000000000000 ) ;
#8083=EDGE_CURVE ( 'NONE', #6883, #11658, #19506, .T. ) ;
#8084=DIRECTION ( 'NONE',  ( 0.01292414190463827932, 0.000000000000000000, 0.9999164797902018176 ) ) ;
#8092=CARTESIAN_POINT ( 'NONE',  ( 68.71681667565954399, 69.99999999999998579, -85.89527988174788220 ) ) ;
#8100=CARTESIAN_POINT ( 'NONE',  ( 105.6376945813395025, 78.65441476617404248, -30.67074184297056405 ) ) ;
#8104=VECTOR ( 'NONE', #10282, 1000.000000000000114 ) ;
#8107=FACE_OUTER_BOUND ( 'NONE', #17152, .T. ) ;
#8112=B_SPLINE_CURVE_WITH_KNOTS ( 'NONE', 3,
 ( #18559, #16844, #20721, #20485, #15469, #13621 ),
 .UNSPECIFIED., .F., .F.,
 ( 4, 2, 4 ),
 ( 2.403703357979454770E-17, 0.0009937831915592871320, 0.001987566383118549978 ),
 .UNSPECIFIED. ) ;
#8113=CARTESIAN_POINT ( 'NONE',  ( 92.11140453220075131, 79.82915613195545745, -31.20677464679435076 ) ) ;
#8114=CIRCLE ( 'NONE', #9951, 1.999999999999997780 ) ;
#8126=( GEOMETRIC_REPRESENTATION_CONTEXT ( 3 ) GLOBAL_UNCERTAINTY_ASSIGNED_CONTEXT ( ( #8743 ) ) GLOBAL_UNIT_ASSIGNED_CONTEXT ( ( #3324, #5034, #10228 ) ) REPRESENTATION_CONTEXT ( 'NONE', 'WORKASPACE' ) );
#8128=CARTESIAN_POINT ( 'NONE',  ( -66.73173682738223533, 70.03297899285537653, 87.44705638319801722 ) ) ;
#8144=DIRECTION ( 'NONE',  ( -0.9999164797902015955, -2.001050586450181282E-22, 0.01292414190463992731 ) ) ;
#8145=DIRECTION ( 'NONE',  ( 0.01292414190464131335, 1.902755938799530239E-22, 0.9999164797902015955 ) ) ;
#8150=VECTOR ( 'NONE', #6714, 1000.000000000000114 ) ;
#8151=CYLINDRICAL_SURFACE ( 'NONE', #8402, 95.00000000000004263 ) ;
#8160=CARTESIAN_POINT ( 'NONE',  ( -1.421655609510531049, 105.0000000000000000, -109.9908127769221977 ) ) ;
#8164=ORIENTED_EDGE ( 'NONE', *, *, #15708, .T. ) ;
#8165=CARTESIAN_POINT ( 'NONE',  ( 37.28121903589197217, 92.86731729164014837, -84.62157808539689086 ) ) ;
#8167=ORIENTED_EDGE ( 'NONE', *, *, #13386, .F. ) ;
#8170=CARTESIAN_POINT ( 'NONE',  ( 106.2052848363078539, 71.73256685213068806, 28.64329287727201034 ) ) ;
#8173=AXIS2_PLACEMENT_3D ( 'NONE', #4028, #11281, #16472 ) ;
#8174=ORIENTED_EDGE ( 'NONE', *, *, #6023, .T. ) ;
#8176=DIRECTION ( 'NONE',  ( -0.01292414190464132896, 0.000000000000000000, -0.9999164797902015955 ) ) ;
#8177=DIRECTION ( 'NONE',  ( 0.9999164797902017066, 2.001050586450178931E-22, -0.01292414190464131508 ) ) ;
#8184=ORIENTED_EDGE ( 'NONE', *, *, #14504, .T. ) ;
#8186=CARTESIAN_POINT ( 'NONE',  ( -89.97337599888878401, 88.77373198860428261, 52.43004476888089727 ) ) ;
#8188=FACE_OUTER_BOUND ( 'NONE', #7632, .T. ) ;
#8193=CARTESIAN_POINT ( 'NONE',  ( -79.92740525950245001, 55.00000000000000000, 6.133505399301367511 ) ) ;
#8194=CARTESIAN_POINT ( 'NONE',  ( -35.95309506732429128, 93.50464841319750064, -82.03286182426641915 ) ) ;
#8199=EDGE_LOOP ( 'NONE', ( #17123, #7967, #22303 ) ) ;
#8200=DIRECTION ( 'NONE',  ( -0.009985269297343229641, -0.6348858185549676181, -0.7725414498878673264 ) ) ;
#8217=CARTESIAN_POINT ( 'NONE',  ( -88.73519446327063065, 70.71303863658374667, 62.85397390640905257 ) ) ;
#8219=ORIENTED_EDGE ( 'NONE', *, *, #880, .T. ) ;
#8229=ADVANCED_FACE ( 'NONE', ( #18355 ), #9214, .F. ) ;
#8230=DIRECTION ( 'NONE',  ( 0.01292414190464131335, 1.902755938799531179E-22, 0.9999164797902017066 ) ) ;
#8231=DIRECTION ( 'NONE',  ( -0.006350819331212801712, 0.8709385446395347952, -0.4913509118287984201 ) ) ;
#8238=EDGE_CURVE ( 'NONE', #10247, #14770, #16173, .T. ) ;
#8239=VERTEX_POINT ( 'NONE', #21998 ) ;
#8253=CARTESIAN_POINT ( 'NONE',  ( -66.06691928577359363, 94.02752048664900997, -82.12548041065298321 ) ) ;
#8255=DIRECTION ( 'NONE',  ( 0.9999164797902017066, 2.001050586450178931E-22, -0.01292414190464131508 ) ) ;
#8258=CARTESIAN_POINT ( 'NONE',  ( 65.88241411543798165, 104.3814432989690602, 67.85066342192635602 ) ) ;
#8262=EDGE_CURVE ( 'NONE', #15798, #9516, #2404, .T. ) ;
#8263=CARTESIAN_POINT ( 'NONE',  ( 1.417778366939166146, 45.00000000000000000, 109.6908378329851246 ) ) ;
#8266=ORIENTED_EDGE ( 'NONE', *, *, #12387, .F. ) ;
#8280=DIRECTION ( 'NONE',  ( -0.01292414190463830014, 0.000000000000000000, -0.9999164797902017066 ) ) ;
#8289=CIRCLE ( 'NONE', #16743, 3.999999999999995559 ) ;
#8291=CARTESIAN_POINT ( 'NONE',  ( -88.16466383535862406, 88.38054089998362883, 52.81015645075888898 ) ) ;
#8293=CARTESIAN_POINT ( 'NONE',  ( -1.079165849037536207, 44.99899999999999523, -83.49302606248184588 ) ) ;
#8301=EDGE_CURVE ( 'NONE', #19631, #9627, #6611, .T. ) ;
#8303=LINE ( 'NONE', #15336, #22135 ) ;
#8313=CARTESIAN_POINT ( 'NONE',  ( -1.079165849037536207, 69.99999999999998579, -83.49302606248184588 ) ) ;
#8325=CARTESIAN_POINT ( 'NONE',  ( -2.067862704742604141, 69.99999999999998579, -159.9866367664322979 ) ) ;
#8328=ORIENTED_EDGE ( 'NONE', *, *, #10385, .F. ) ;
#8330=ORIENTED_EDGE ( 'NONE', *, *, #20378, .T. ) ;
#8333=EDGE_CURVE ( 'NONE', #12220, #2857, #3727, .T. ) ;
#8374=CARTESIAN_POINT ( 'NONE',  ( -88.18706637290659955, 88.71869973106718987, 50.32066939225188662 ) ) ;
#8375=ORIENTED_EDGE ( 'NONE', *, *, #20997, .T. ) ;
#8379=CARTESIAN_POINT ( 'NONE',  ( 90.40889375659912730, 78.43035437438885538, -33.17122784026042837 ) ) ;
#8382=VECTOR ( 'NONE', #7644, 1000.000000000000000 ) ;
#8386=VECTOR ( 'NONE', #3116, 1000.000000000000114 ) ;
#8389=CARTESIAN_POINT ( 'NONE',  ( -89.95410508456485843, 88.80250242289463358, 52.38924411555903760 ) ) ;
#8392=DIRECTION ( 'NONE',  ( -0.8588562297929583922, -0.3902276408394327323, 0.3317956673477156504 ) ) ;
#8396=CARTESIAN_POINT ( 'NONE',  ( -88.16340328200274712, 88.26057420812728083, 52.92017833001973770 ) ) ;
#8397=CARTESIAN_POINT ( 'NONE',  ( -88.55404276674165942, 79.97526064827543735, 31.48874835467963607 ) ) ;
#8400=EDGE_CURVE ( 'NONE', #7605, #12053, #5012, .T. ) ;
#8402=AXIS2_PLACEMENT_3D ( 'NONE', #15294, #20416, #8023 ) ;
#8403=ORIENTED_EDGE ( 'NONE', *, *, #1489, .T. ) ;
#8405=DIRECTION ( 'NONE',  ( -0.01292414190464044946, -4.254338997373069277E-37, -0.9999164797902017066 ) ) ;
#8406=CARTESIAN_POINT ( 'NONE',  ( 88.42085790543281121, 80.22997387171264450, -32.23265953185130428 ) ) ;
#8410=FACE_OUTER_BOUND ( 'NONE', #14511, .T. ) ;
#8412=ORIENTED_EDGE ( 'NONE', *, *, #2177, .F. ) ;
#8417=EDGE_CURVE ( 'NONE', #4942, #3481, #8931, .T. ) ;
#8423=CARTESIAN_POINT ( 'NONE',  ( -89.90382325080345538, 72.53934035976358530, 61.83857552320039730 ) ) ;
#8425=CARTESIAN_POINT ( 'NONE',  ( -91.74710091628168129, 71.28171241778764511, -60.68341510339269007 ) ) ;
#8431=CIRCLE ( 'NONE', #5856, 2.000000000000004885 ) ;
#8438=ORIENTED_EDGE ( 'NONE', *, *, #22223, .F. ) ;
#8442=AXIS2_PLACEMENT_3D ( 'NONE', #2554, #6105, #7719 ) ;
#8461=DIRECTION ( 'NONE',  ( 0.01292414190464131335, 0.000000000000000000, 0.9999164797902017066 ) ) ;
#8481=CARTESIAN_POINT ( 'NONE',  ( -90.16222517276825954, 87.23703400121539175, 51.25429106922742051 ) ) ;
#8485=CARTESIAN_POINT ( 'NONE',  ( 106.0939156777172485, 70.76422767839095229, 29.05317630099624893 ) ) ;
#8491=AXIS2_PLACEMENT_3D ( 'NONE', #13212, #8255, #20181 ) ;
#8500=CARTESIAN_POINT ( 'NONE',  ( -90.08563665347566030, 88.51714521506588085, 52.72240440167576025 ) ) ;
#8501=EDGE_CURVE ( 'NONE', #4637, #9075, #16316, .T. ) ;
#8502=AXIS2_PLACEMENT_3D ( 'NONE', #16239, #8851, #12546 ) ;
#8513=CARTESIAN_POINT ( 'NONE',  ( 84.91238002074454982, 75.00865516402794242, -2.421554962614585360 ) ) ;
#8517=ORIENTED_EDGE ( 'NONE', *, *, #13583, .T. ) ;
#8524=ADVANCED_FACE ( 'NONE', ( #17912 ), #21537, .F. ) ;
#8525=ORIENTED_EDGE ( 'NONE', *, *, #247, .T. ) ;
#8527=DIRECTION ( 'NONE',  ( 0.01292414190464217898, 1.902755938799531885E-22, 0.9999164797902015955 ) ) ;
#8528=CARTESIAN_POINT ( 'NONE',  ( 90.75111155332047019, 98.75957274858882329, 62.16377225325069844 ) ) ;
#8529=DIRECTION ( 'NONE',  ( 2.025474946048326158E-22, -1.000000000000000000, 1.876735158486679638E-22 ) ) ;
#8534=CIRCLE ( 'NONE', #15163, 5.099999999999992539 ) ;
#8535=LINE ( 'NONE', #3034, #15236 ) ;
#8548=CARTESIAN_POINT ( 'NONE',  ( -91.23603883849614249, 79.86121811340019860, -30.82342686631250217 ) ) ;
#8552=CARTESIAN_POINT ( 'NONE',  ( -90.17340641399441381, 87.01242838177741135, 51.39043932755232902 ) ) ;
#8557=DIRECTION ( 'NONE',  ( 2.025474946048326158E-22, -1.000000000000000000, 1.876735158486679638E-22 ) ) ;
#8558=EDGE_LOOP ( 'NONE', ( #7932, #21056 ) ) ;
#8565=CARTESIAN_POINT ( 'NONE',  ( -104.8202145123291018, 69.99999999999998579, 33.35749735200943178 ) ) ;
#8573=DIRECTION ( 'NONE',  ( -0.01292414190464131335, 0.000000000000000000, -0.9999164797902017066 ) ) ;
#8574=ADVANCED_FACE ( 'NONE', ( #6167 ), #22350, .F. ) ;
#8581=CARTESIAN_POINT ( 'NONE',  ( -92.14659905926313854, 77.13858430795839638, 31.20924108170686040 ) ) ;
#8587=CARTESIAN_POINT ( 'NONE',  ( -41.56623493000981284, 72.00000000000000000, -82.46967996629571473 ) ) ;
#8592=AXIS2_PLACEMENT_3D ( 'NONE', #6383, #9359, #18118 ) ;
#8595=DIRECTION ( 'NONE',  ( -0.9999164797902017066, -5.258382537605284335E-16, 0.01292414190464131508 ) ) ;
#8603=DIRECTION ( 'NONE',  ( 0.9999164797902017066, 2.001050586450178695E-22, -0.01292414190464131508 ) ) ;
#8605=DIRECTION ( 'NONE',  ( -2.025474946048326158E-22, 1.000000000000000000, -1.876735158486679638E-22 ) ) ;
#8606=ORIENTED_EDGE ( 'NONE', *, *, #11291, .T. ) ;
#8611=ORIENTED_EDGE ( 'NONE', *, *, #13936, .F. ) ;
#8612=DIRECTION ( 'NONE',  ( -0.9999164797902017066, -2.001050586450178931E-22, 0.01292414190464131508 ) ) ;
#8613=ADVANCED_FACE ( 'NONE', ( #7891 ), #4310, .T. ) ;
#8614=CARTESIAN_POINT ( 'NONE',  ( -89.89702621265139726, 88.86943147588976899, 52.27963238237415311 ) ) ;
#8619=FACE_OUTER_BOUND ( 'NONE', #21912, .T. ) ;
#8620=CARTESIAN_POINT ( 'NONE',  ( 91.21019055468687498, 72.00000000000000000, 28.82359390673205723 ) ) ;
#8621=CARTESIAN_POINT ( 'NONE',  ( 41.59208321381912299, 91.17157287525387233, 84.46951292587608862 ) ) ;
#8622=CARTESIAN_POINT ( 'NONE',  ( 84.38591728079271093, 75.03398072390710638, -3.646888635650151311 ) ) ;
#8624=VERTEX_POINT ( 'NONE', #4428 ) ;
#8629=CARTESIAN_POINT ( 'NONE',  ( 85.63433794141033673, 105.0000000000000000, 69.04172771111926465 ) ) ;
#8632=CARTESIAN_POINT ( 'NONE',  ( -105.7099399341925192, 78.83711888896343112, 30.42080736548454212 ) ) ;
#8641=EDGE_CURVE ( 'NONE', #369, #16780, #12970, .T. ) ;
#8657=DIRECTION ( 'NONE',  ( -2.025474946048326158E-22, 1.000000000000000000, -1.876735158486679638E-22 ) ) ;
#8678=CARTESIAN_POINT ( 'NONE',  ( 70.91392079944854743, 69.99999999999998579, 84.09052168258639881 ) ) ;
#8680=CARTESIAN_POINT ( 'NONE',  ( 85.01653497985981289, 104.3814432989690602, -69.80106575130697877 ) ) ;
#8681=LINE ( 'NONE', #12283, #8767 ) ;
#8685=CARTESIAN_POINT ( 'NONE',  ( 41.61793149762840471, 69.99999999999998579, 86.46934588545650513 ) ) ;
#8691=EDGE_CURVE ( 'NONE', #5449, #11742, #781, .T. ) ;
#8700=ORIENTED_EDGE ( 'NONE', *, *, #13529, .T. ) ;
#8706=AXIS2_PLACEMENT_3D ( 'NONE', #15081, #12072, #8280 ) ;
#8714=CYLINDRICAL_SURFACE ( 'NONE', #3238, 5.099999999999992539 ) ;
#8716=CARTESIAN_POINT ( 'NONE',  ( -88.16708379909647419, 88.58102416753696673, 52.59057003169024824 ) ) ;
#8725=CARTESIAN_POINT ( 'NONE',  ( 84.54811758989713155, 75.02636992936612614, -3.352151862290983608 ) ) ;
#8731=CARTESIAN_POINT ( 'NONE',  ( -75.62605524907648658, 75.03814149158517921, 3.672988387105930119 ) ) ;
#8733=CARTESIAN_POINT ( 'NONE',  ( -105.4775731789987674, 77.90269639574782445, 31.21677525025618039 ) ) ;
#8734=CARTESIAN_POINT ( 'NONE',  ( -35.95309506732429128, 93.50464841319750064, -82.03286182426641915 ) ) ;
#8735=CARTESIAN_POINT ( 'NONE',  ( 70.91392079944854743, 72.00000000000000000, 84.09052168258639881 ) ) ;
#8738=CARTESIAN_POINT ( 'NONE',  ( -39.11273342774205730, 91.99797716581187501, -83.46418088055293083 ) ) ;
#8742=EDGE_LOOP ( 'NONE', ( #903, #15900, #3968, #9123 ) ) ;
#8743=UNCERTAINTY_MEASURE_WITH_UNIT (LENGTH_MEASURE( 1.000000000000000082E-05 ), #3324, 'distance_accuracy_value', 'NONE');
#8750=EDGE_CURVE ( 'NONE', #11360, #7130, #4423, .T. ) ;
#8752=CARTESIAN_POINT ( 'NONE',  ( 106.0833544754547972, 79.13355406794953240, -29.09322962842207971 ) ) ;
#8758=CARTESIAN_POINT ( 'NONE',  ( 91.32251664931575874, 80.22595383786462264, 29.89762933574812465 ) ) ;
#8760=CARTESIAN_POINT ( 'NONE',  ( 89.59766859896282654, 79.73843791202818920, 28.47398564242246977 ) ) ;
#8761=ORIENTED_EDGE ( 'NONE', *, *, #20324, .T. ) ;
#8766=CARTESIAN_POINT ( 'NONE',  ( 1.721625266288852263, 105.0000000000000000, 109.9865264768483968 ) ) ;
#8767=VECTOR ( 'NONE', #15730, 1000.000000000000114 ) ;
#8769=CARTESIAN_POINT ( 'NONE',  ( -92.35175351209242933, 79.88298967447890675, -28.93780754488527052 ) ) ;
#8771=ADVANCED_FACE ( 'NONE', ( #18796 ), #4987, .T. ) ;
#8772=LINE ( 'NONE', #1912, #15093 ) ;
#8781=CYLINDRICAL_SURFACE ( 'NONE', #9077, 2.000000000000004441 ) ;
#8789=VERTEX_POINT ( 'NONE', #18899 ) ;
#8791=VECTOR ( 'NONE', #16431, 1000.000000000000114 ) ;
#8795=CARTESIAN_POINT ( 'NONE',  ( 89.22767861003025303, 80.31838830481380853, 30.18953644180655971 ) ) ;
#8798=CARTESIAN_POINT ( 'NONE',  ( 64.99457118636311748, 105.0000000000000000, -0.8400692238016954638 ) ) ;
#8806=CARTESIAN_POINT ( 'NONE',  ( 36.94244151028511425, 91.99797716581187501, -84.44721085690419216 ) ) ;
#8809=CARTESIAN_POINT ( 'NONE',  ( 394.9504264446939032, 92.58578643762699301, -89.52608615654116875 ) ) ;
#8810=ADVANCED_FACE ( 'NONE', ( #6727, #13751 ), #20736, .T. ) ;
#8811=AXIS2_PLACEMENT_3D ( 'NONE', #5671, #7064, #12709 ) ;
#8815=DIRECTION ( 'NONE',  ( 0.9999164797902017066, 2.001050586450178931E-22, -0.01292414190464131508 ) ) ;
#8817=CARTESIAN_POINT ( 'NONE',  ( -110.3452273899772962, 79.04398536104962147, -25.99873445483951073 ) ) ;
#8819=EDGE_LOOP ( 'NONE', ( #12542, #17468, #17143, #8001 ) ) ;
#8828=( BOUNDED_SURFACE ( )  B_SPLINE_SURFACE ( 3, 2, ( 
 ( #22353, #6649, #18932 ),
 ( #13784, #6867, #14487 ),
 ( #17922, #12175, #21113 ),
 ( #5363, #14705, #14593 ) ),
 .UNSPECIFIED., .F., .F., .T. ) 
 B_SPLINE_SURFACE_WITH_KNOTS ( ( 4, 4 ),
 ( 3, 3 ),
 ( 5.799006443144740786, 5.860583945225279479 ),
 ( 0.000000000000000000, 1.000000000000000000 ),
 .UNSPECIFIED. ) 
 GEOMETRIC_REPRESENTATION_ITEM ( )  RATIONAL_B_SPLINE_SURFACE ( (
 ( 1.000000000000000000, 0.9016180287879261845, 1.000000000000000000),
 ( 1.000000000000000000, 0.9034913259101577943, 1.000000000000000000),
 ( 1.000000000000000000, 0.9052491015987668144, 1.000000000000000000),
 ( 1.000000000000000000, 0.9068900557993655465, 1.000000000000000000) ) ) 
 REPRESENTATION_ITEM ( '' )  SURFACE ( )  );
#8832=CARTESIAN_POINT ( 'NONE',  ( 1.364374947835851710E-14, 55.00000000000000000, -9.836440897896405351E-15 ) ) ;
#8841=CARTESIAN_POINT ( 'NONE',  ( 90.05385374424744782, 71.62832261676159362, -63.16885269282647641 ) ) ;
#8843=CARTESIAN_POINT ( 'NONE',  ( -90.06799945166942223, 87.57178311039056950, 51.04991898090875679 ) ) ;
#8847=VERTEX_POINT ( 'NONE', #8552 ) ;
#8850=AXIS2_PLACEMENT_3D ( 'NONE', #623, #5659, #12695 ) ;
#8851=DIRECTION ( 'NONE',  ( 0.8077751305149092342, -0.4220031449644174315, 0.4115977212786322004 ) ) ;
#8860=VECTOR ( 'NONE', #2414, 1000.000000000000114 ) ;
#8866=ADVANCED_FACE ( 'NONE', ( #21076 ), #10966, .F. ) ;
#8875=DIRECTION ( 'NONE',  ( 0.9999164797902017066, 2.001050586450178931E-22, -0.01292414190464131508 ) ) ;
#8877=ORIENTED_EDGE ( 'NONE', *, *, #7756, .F. ) ;
#8886=CARTESIAN_POINT ( 'NONE',  ( -64.28883878761487836, 83.29019440189557599, 55.44125366118053932 ) ) ;
#8889=CARTESIAN_POINT ( 'NONE',  ( 91.61331032192579471, 77.62808270880876194, 29.62115891282539692 ) ) ;
#8898=CARTESIAN_POINT ( 'NONE',  ( -1.163172771417704698, 44.99899999999999523, -89.99248318111816047 ) ) ;
#8900=CARTESIAN_POINT ( 'NONE',  ( -70.53865358177314704, 70.91952051830753589, -84.40563445996846781 ) ) ;
#8901=EDGE_CURVE ( 'NONE', #12496, #5690, #9932, .T. ) ;
#8904=CIRCLE ( 'NONE', #14821, 1.989999999999999103 ) ;
#8905=PLANE ( 'NONE',  #18820 ) ;
#8911=LINE ( 'NONE', #19365, #19582 ) ;
#8931=B_SPLINE_CURVE_WITH_KNOTS ( 'NONE', 3,
 ( #17332, #19144, #8581, #15620, #6854, #16187, #6971, #13998, #5238, #12282, #19264, #10542, #17561, #1812, #18022, #16080 ),
 .UNSPECIFIED., .F., .F.,
 ( 4, 2, 2, 2, 2, 2, 2, 4 ),
 ( 0.000000000000000000, 0.0004291333152394312378, 0.0008582666304788624757, 0.001716533260957770054, 0.002145666576197221946, 0.002574799891436673621, 0.003003933206676125730, 0.003433066521915577405 ),
 .UNSPECIFIED. ) ;
#8932=CARTESIAN_POINT ( 'NONE',  ( -39.42082737383935154, 91.17157287525387233, 83.51645567887779009 ) ) ;
#8934=CARTESIAN_POINT ( 'NONE',  ( 35.92446336679496000, 93.51775827232349059, 82.02042234242476582 ) ) ;
#8936=DIRECTION ( 'NONE',  ( 0.01292414190464178173, 1.902755938799531414E-22, 0.9999164797902017066 ) ) ;
#8937=EDGE_CURVE ( 'NONE', #14770, #7130, #5777, .T. ) ;
#8950=EDGE_CURVE ( 'NONE', #8624, #16665, #19784, .T. ) ;
#8953=CARTESIAN_POINT ( 'NONE',  ( 38.69757710431291287, 94.02752048664899576, 82.47923521851859618 ) ) ;
#8960=CARTESIAN_POINT ( 'NONE',  ( -90.09360468281239775, 87.50216161139763926, 51.09253514669736518 ) ) ;
#8962=ADVANCED_FACE ( 'NONE', ( #5331 ), #15818, .T. ) ;
#8964=DIRECTION ( 'NONE',  ( -2.025474946048326393E-22, 1.000000000000000000, -1.876735158486679873E-22 ) ) ;
#8965=( BOUNDED_CURVE ( )  B_SPLINE_CURVE ( 3, ( #19642, #11161, #16580, #16697 ),
 .UNSPECIFIED., .F., .T. ) 
 B_SPLINE_CURVE_WITH_KNOTS ( ( 4, 4 ),
 ( 0.4229686233981270749, 0.4841788640348455575 ),
 .UNSPECIFIED. ) 
 CURVE ( )  GEOMETRIC_REPRESENTATION_ITEM ( )  RATIONAL_B_SPLINE_CURVE ( ( 1.000000000000000000, 0.9996877999070342691, 0.9996877999070342691, 1.000000000000000000 ) ) 
 REPRESENTATION_ITEM ( '' )  );
#8967=CIRCLE ( 'NONE', #5670, 1.999999999999999112 ) ;
#8968=CARTESIAN_POINT ( 'NONE',  ( 81.38158604529294848, 75.12830914639056346, 3.884784555313749888 ) ) ;
#8969=CARTESIAN_POINT ( 'NONE',  ( -64.98109895693632154, 170.8565945647193587, 1.882390201297356347 ) ) ;
#8970=ORIENTED_EDGE ( 'NONE', *, *, #17846, .T. ) ;
#8971=CARTESIAN_POINT ( 'NONE',  ( 91.27111462898963623, 78.10400798472784345, 30.35002675991152898 ) ) ;
#8973=FACE_OUTER_BOUND ( 'NONE', #4269, .T. ) ;
#8980=ORIENTED_EDGE ( 'NONE', *, *, #11755, .T. ) ;
#8981=CARTESIAN_POINT ( 'NONE',  ( -91.23603883849614249, 72.00000000000000000, -30.82342686631250217 ) ) ;
#8985=CARTESIAN_POINT ( 'NONE',  ( 41.56623493000984126, 91.17157287525387233, 82.46967996629570052 ) ) ;
#8987=AXIS2_PLACEMENT_3D ( 'NONE', #843, #6556, #8176 ) ;
#9003=CARTESIAN_POINT ( 'NONE',  ( 91.45164190239772495, 80.14421549785700449, 29.66212192225453848 ) ) ;
#9009=CARTESIAN_POINT ( 'NONE',  ( -91.87497954589036908, 77.44324451750601668, -29.32612497091890802 ) ) ;
#9015=PLANE ( 'NONE',  #1403 ) ;
#9020=CARTESIAN_POINT ( 'NONE',  ( 80.05923150692980528, 75.13699351169597662, 4.065642694558706083 ) ) ;
#9021=DIRECTION ( 'NONE',  ( -0.9999164797902017066, -2.001050586450178931E-22, 0.01292414190464131508 ) ) ;
#9023=CARTESIAN_POINT ( 'NONE',  ( -90.65029634199436259, 79.17021053268413766, 29.01211804384233517 ) ) ;
#9030=CARTESIAN_POINT ( 'NONE',  ( 41.56623493000984126, 72.00000000000000000, 82.46967996629570052 ) ) ;
#9033=EDGE_CURVE ( 'NONE', #15210, #18024, #5889, .T. ) ;
#9037=CARTESIAN_POINT ( 'NONE',  ( 39.42082737383939417, 91.17157287525388654, -83.51645567887783272 ) ) ;
#9040=CARTESIAN_POINT ( 'NONE',  ( 88.24077620913463704, 100.2813628572214384, -65.67913105001751717 ) ) ;
#9044=VERTEX_POINT ( 'NONE', #11425 ) ;
#9057=B_SPLINE_CURVE_WITH_KNOTS ( 'NONE', 3,
 ( #6121, #16610, #20113, #2344, #9345, #17878, #7388, #14432, #16382, #7615, #14654, #19897, #4167, #11194, #18422, #13711, #16937, #1315 ),
 .UNSPECIFIED., .F., .F.,
 ( 4, 2, 2, 2, 2, 2, 2, 2, 4 ),
 ( 0.000000000000000000, 0.0008023074076923488894, 0.001604614815384697779, 0.002406922223077046560, 0.003209229630769395557, 0.004011537038461744122, 0.004813844446154093119, 0.005616151853846442117, 0.006418459261538791115 ),
 .UNSPECIFIED. ) ;
#9059=CARTESIAN_POINT ( 'NONE',  ( -88.16590590355198742, 88.48929759811795748, 52.69915227853057615 ) ) ;
#9061=EDGE_CURVE ( 'NONE', #14836, #3481, #5519, .T. ) ;
#9066=DIRECTION ( 'NONE',  ( -0.004263634442766563518, -0.9440169652124856814, -0.3298693541575922761 ) ) ;
#9073=B_SPLINE_CURVE_WITH_KNOTS ( 'NONE', 3,
 ( #17191, #16993, #11463, #4887, #15709, #8900, #14102, #3619, #20743, #71, #17785, #10630, #17541, #17433 ),
 .UNSPECIFIED., .F., .F.,
 ( 4, 2, 2, 2, 2, 2, 4 ),
 ( 0.000000000000000000, 0.0005169893790259204921, 0.001033978758051840984, 0.001550968137077761476, 0.002067957516103681968, 0.003101936274155522952, 0.004135915032207363937 ),
 .UNSPECIFIED. ) ;
#9074=CARTESIAN_POINT ( 'NONE',  ( 92.91906646248270363, 77.13883058002313931, 28.81763569833105976 ) ) ;
#9075=VERTEX_POINT ( 'NONE', #13062 ) ;
#9077=AXIS2_PLACEMENT_3D ( 'NONE', #17896, #12720, #15832 ) ;
#9081=DIRECTION ( 'NONE',  ( -2.025474946048326158E-22, 1.000000000000000000, -1.876735158486679638E-22 ) ) ;
#9084=CARTESIAN_POINT ( 'NONE',  ( 105.1274178938603825, 70.25451017443431567, -32.37651503794369034 ) ) ;
#9087=ADVANCED_FACE ( 'NONE', ( #7624 ), #19084, .F. ) ;
#9092=CARTESIAN_POINT ( 'NONE',  ( -83.78835501158950194, 75.05963785504690122, 4.457120374836909704 ) ) ;
#9095=( BOUNDED_SURFACE ( )  B_SPLINE_SURFACE ( 3, 2, ( 
 ( #20739, #4990, #12018 ),
 ( #19006, #3268, #1570 ),
 ( #22543, #6836, #19121 ),
 ( #3398, #5217, #19354 ),
 ( #12711, #17657, #3733 ),
 ( #17780, #20959, #21299 ),
 ( #10752, #19678, #16291 ),
 ( #1788, #15822, #12479 ),
 ( #19465, #21079, #10969 ),
 ( #9009, #19243, #3508 ),
 ( #5335, #8769, #3947 ),
 ( #2021, #21412, #13968 ),
 ( #14098, #12597, #12373 ),
 ( #10524, #17997, #17538 ),
 ( #188, #10626, #1906 ),
 ( #3614, #5565, #412 ),
 ( #2236, #15946, #67 ),
 ( #12254, #14451, #7067 ) ),
 .UNSPECIFIED., .F., .F., .T. ) 
 B_SPLINE_SURFACE_WITH_KNOTS ( ( 4, 2, 2, 2, 2, 2, 2, 2, 4 ),
 ( 3, 3 ),
 ( 0.003005090483489989556, 0.003807341501471057498, 0.004609592519452125441, 0.005411843537433192949, 0.006214094555414261326, 0.007016345573395328834, 0.007818596591376396343, 0.008620847609357464719, 0.009423098627338533095 ),
 ( 0.000000000000000000, 1.000000000000000000 ),
 .UNSPECIFIED. ) 
 GEOMETRIC_REPRESENTATION_ITEM ( )  RATIONAL_B_SPLINE_SURFACE ( (
 ( 1.000000000000000000, 0.7071067811865485719, 1.000000000000000000),
 ( 1.000000000000000000, 0.6996407321460798023, 1.000000000000000000),
 ( 1.000000000000000000, 0.6923367522676026065, 1.000000000000000000),
 ( 1.000000000000000000, 0.6780525511373404202, 1.000000000000000000),
 ( 1.000000000000000000, 0.6710180578259783424, 1.000000000000000000),
 ( 1.000000000000000000, 0.6575437683257994159, 1.000000000000000000),
 ( 1.000000000000000000, 0.6511910073847769764, 1.000000000000000000),
 ( 1.000000000000000000, 0.6392329869082821192, 1.000000000000000000),
 ( 1.000000000000000000, 0.6335699185532992495, 1.000000000000000000),
 ( 1.000000000000000000, 0.6233860397584745083, 1.000000000000000000),
 ( 1.000000000000000000, 0.6188536248677669604, 1.000000000000000000),
 ( 1.000000000000000000, 0.6108845495338486309, 1.000000000000000000),
 ( 1.000000000000000000, 0.6074396204518894837, 1.000000000000000000),
 ( 1.000000000000000000, 0.6019717515916982453, 1.000000000000000000),
 ( 1.000000000000000000, 0.5998961748958268059, 1.000000000000000000),
 ( 1.000000000000000000, 0.5970819659646876554, 1.000000000000000000),
 ( 1.000000000000000000, 0.5963755918899067421, 1.000000000000000000),
 ( 1.000000000000000000, 0.5963808372950819559, 1.000000000000000000) ) ) 
 REPRESENTATION_ITEM ( '' )  SURFACE ( )  );
#9097=EDGE_LOOP ( 'NONE', ( #19053, #8700, #20878, #18030, #947 ) ) ;
#9102=VECTOR ( 'NONE', #7529, 1000.000000000000114 ) ;
#9110=B_SPLINE_CURVE_WITH_KNOTS ( 'NONE', 3,
 ( #8734, #5648, #7038, #17088, #21049, #15789, #17507, #3585 ),
 .UNSPECIFIED., .F., .F.,
 ( 4, 2, 2, 4 ),
 ( 4.486197489951441732E-16, 0.0007139082715502006972, 0.001427816543099952751, 0.002855633086199477026 ),
 .UNSPECIFIED. ) ;
#9111=CARTESIAN_POINT ( 'NONE',  ( 89.22443767324084263, 80.23075532867255788, 29.93879111800735870 ) ) ;
#9112=CARTESIAN_POINT ( 'NONE',  ( 89.22767861003025303, 80.31838830481380853, 30.18953644180655971 ) ) ;
#9113=ORIENTED_EDGE ( 'NONE', *, *, #17226, .T. ) ;
#9123=ORIENTED_EDGE ( 'NONE', *, *, #12387, .T. ) ;
#9129=CARTESIAN_POINT ( 'NONE',  ( 85.09289243014617909, 54.99999999999999289, -1.099844476084985700 ) ) ;
#9130=DIRECTION ( 'NONE',  ( 0.01292414190464131335, 1.902755938799530239E-22, 0.9999164797902015955 ) ) ;
#9140=CARTESIAN_POINT ( 'NONE',  ( -91.40469917791146770, 79.08369667522879354, 28.73783386972080223 ) ) ;
#9151=ORIENTED_EDGE ( 'NONE', *, *, #13317, .T. ) ;
#9152=AXIS2_PLACEMENT_3D ( 'NONE', #230, #12523, #10677 ) ;
#9168=CARTESIAN_POINT ( 'NONE',  ( 7.165475679525708408, 86.29954751296186544, 75.08469730518739027 ) ) ;
#9173=ADVANCED_FACE ( 'NONE', ( #9712 ), #13275, .F. ) ;
#9174=LINE ( 'NONE', #12759, #10270 ) ;
#9179=CARTESIAN_POINT ( 'NONE',  ( -88.96403593049780056, 88.58898090146213633, 50.41366170828801074 ) ) ;
#9185=ORIENTED_EDGE ( 'NONE', *, *, #10277, .T. ) ;
#9190=CARTESIAN_POINT ( 'NONE',  ( -106.2089377515398922, 71.86507807689916660, -28.62973177816246917 ) ) ;
#9191=CARTESIAN_POINT ( 'NONE',  ( -91.51031840793912409, 96.48503848149375983, -61.03988419336481996 ) ) ;
#9194=CARTESIAN_POINT ( 'NONE',  ( -63.99205529224568068, 99.43075776215394512, 78.40283286226222970 ) ) ;
#9199=CARTESIAN_POINT ( 'NONE',  ( -75.89761971758728976, 75.05050884166004721, 4.091003432312519728 ) ) ;
#9201=CARTESIAN_POINT ( 'NONE',  ( -88.07410310386867991, 72.00000000000001421, 59.83417019015373484 ) ) ;
#9212=AXIS2_PLACEMENT_3D ( 'NONE', #22290, #6581, #3133 ) ;
#9214=TOROIDAL_SURFACE ( 'NONE', #2938, 83.00000000000001421, 2.000000000000000000 ) ;
#9217=ORIENTED_EDGE ( 'NONE', *, *, #5108, .F. ) ;
#9218=ORIENTED_EDGE ( 'NONE', *, *, #21109, .F. ) ;
#9220=CARTESIAN_POINT ( 'NONE',  ( 92.40872671617952960, 69.99999999999998579, -33.19707612406970298 ) ) ;
#9225=CARTESIAN_POINT ( 'NONE',  ( 68.97076059960825489, 70.03291683438813209, 85.69217454375154830 ) ) ;
#9229=CARTESIAN_POINT ( 'NONE',  ( -92.40872671617950118, 72.00000000000000000, 33.19707612406966035 ) ) ;
#9232=CARTESIAN_POINT ( 'NONE',  ( 89.33542534687491354, 79.97945796766221349, 29.20190675877598352 ) ) ;
#9233=DIRECTION ( 'NONE',  ( -0.01292414190464131335, 0.000000000000000000, -0.9999164797902017066 ) ) ;
#9240=CYLINDRICAL_SURFACE ( 'NONE', #20469, 6.499999999999998224 ) ;
#9247=CARTESIAN_POINT ( 'NONE',  ( 74.91776319474617196, 75.00176710950381676, -1.633185153038630100 ) ) ;
#9251=CARTESIAN_POINT ( 'NONE',  ( 1.364373935098378649E-14, 105.0000000000000000, -9.836450281572198869E-15 ) ) ;
#9257=CIRCLE ( 'NONE', #5581, 110.0000000000000000 ) ;
#9258=CARTESIAN_POINT ( 'NONE',  ( 93.18417523045800976, 77.12912189496647386, 26.79791266334236610 ) ) ;
#9262=CARTESIAN_POINT ( 'NONE',  ( -91.76144944056422048, 79.85812038788782274, 31.26012496009715846 ) ) ;
#9267=ADVANCED_FACE ( 'NONE', ( #14470 ), #10539, .F. ) ;
#9274=VERTEX_POINT ( 'NONE', #3868 ) ;
#9277=CARTESIAN_POINT ( 'NONE',  ( 75.90743353164279483, 96.21294322789843534, 79.81268430165899019 ) ) ;
#9279=VERTEX_POINT ( 'NONE', #21096 ) ;
#9280=LINE ( 'NONE', #10895, #4853 ) ;
#9297=VERTEX_POINT ( 'NONE', #16076 ) ;
#9301=VECTOR ( 'NONE', #11962, 1000.000000000000114 ) ;
#9302=FACE_OUTER_BOUND ( 'NONE', #14214, .T. ) ;
#9303=CARTESIAN_POINT ( 'NONE',  ( -88.18570483488321088, 88.83504250765321331, 50.51296395271546658 ) ) ;
#9306=VERTEX_POINT ( 'NONE', #2141 ) ;
#9313=ORIENTED_EDGE ( 'NONE', *, *, #4824, .F. ) ;
#9318=CARTESIAN_POINT ( 'NONE',  ( 93.06424251235320355, 77.12912189496643123, 28.79962987465162172 ) ) ;
#9321=CARTESIAN_POINT ( 'NONE',  ( -91.23296681615020987, 78.26422321607698507, -30.58575029229929143 ) ) ;
#9331=EDGE_LOOP ( 'NONE', ( #20581, #3078, #4498, #3558 ) ) ;
#9336=CARTESIAN_POINT ( 'NONE',  ( -105.3709006619169628, 71.09718787230099224, 31.57492962159251348 ) ) ;
#9337=ORIENTED_EDGE ( 'NONE', *, *, #13936, .T. ) ;
#9341=CYLINDRICAL_SURFACE ( 'NONE', #8850, 2.000000000000004885 ) ;
#9345=CARTESIAN_POINT ( 'NONE',  ( -91.86780221137910019, 79.10677575599461875, -26.44518439498801854 ) ) ;
#9347=EDGE_CURVE ( 'NONE', #7130, #9297, #15483, .T. ) ;
#9350=CARTESIAN_POINT ( 'NONE',  ( -0.9693106428480923187, 86.14745084375785211, -74.99373598426512899 ) ) ;
#9357=ORIENTED_EDGE ( 'NONE', *, *, #8238, .F. ) ;
#9359=DIRECTION ( 'NONE',  ( 0.01125613334114312913, 0.4913919529878050807, 0.8708658036695648974 ) ) ;
#9364=CARTESIAN_POINT ( 'NONE',  ( 77.49749086929654140, 75.10304909037273546, 3.426285700830333791 ) ) ;
#9371=VERTEX_POINT ( 'NONE', #19261 ) ;
#9376=EDGE_CURVE ( 'NONE', #13307, #10113, #8114, .T. ) ;
#9377=CARTESIAN_POINT ( 'NONE',  ( 90.90077733783162728, 77.56213813822601821, -31.87679858714243153 ) ) ;
#9379=CARTESIAN_POINT ( 'NONE',  ( -90.51848467603900872, 80.22648697776344306, 32.24949179442770486 ) ) ;
#9380=CARTESIAN_POINT ( 'NONE',  ( 41.56623493000986258, 91.17157287525387233, 82.46967996629570052 ) ) ;
#9393=CARTESIAN_POINT ( 'NONE',  ( 1.117803423002105445, 55.00000000000000000, 109.6947150755565161 ) ) ;
#9398=CARTESIAN_POINT ( 'NONE',  ( -106.3651776870870833, 78.54983655346497073, -28.04389441634544866 ) ) ;
#9402=CARTESIAN_POINT ( 'NONE',  ( -2.116856996920899014, 86.19447564219862556, 75.08617727949184939 ) ) ;
#9410=CARTESIAN_POINT ( 'NONE',  ( -89.37770891450712440, 88.38797322560618852, 50.54303061661246943 ) ) ;
#9419=CARTESIAN_POINT ( 'NONE',  ( -105.7217631510340681, 70.01235472379876512, -30.37969943364871028 ) ) ;
#9423=CARTESIAN_POINT ( 'NONE',  ( 0.4135725409485815351, 72.00000000000000000, 31.99732735328655053 ) ) ;
#9426=CYLINDRICAL_SURFACE ( 'NONE', #19577, 2.000000000000001332 ) ;
#9430=DIRECTION ( 'NONE',  ( 0.9999164797902017066, 0.000000000000000000, -0.01292414190463832269 ) ) ;
#9437=VERTEX_POINT ( 'NONE', #3136 ) ;
#9439=CARTESIAN_POINT ( 'NONE',  ( -83.05224505503836951, 75.08638595516889325, 5.128520313100306538 ) ) ;
#9440=CARTESIAN_POINT ( 'NONE',  ( -90.16487608766178141, 87.18261312935477747, 51.28728107363841104 ) ) ;
#9441=B_SPLINE_CURVE_WITH_KNOTS ( 'NONE', 3,
 ( #11874, #15444, #10033, #13487, #22397, #15105, #20804, #11754, #1531, #11984 ),
 .UNSPECIFIED., .F., .F.,
 ( 4, 2, 2, 2, 4 ),
 ( 6.509259464525837440E-17, 0.0004376694309007175192, 0.0008753388618013698778, 0.001313008292702022399, 0.001750677723602674703 ),
 .UNSPECIFIED. ) ;
#9443=ORIENTED_EDGE ( 'NONE', *, *, #7525, .T. ) ;
#9446=LINE ( 'NONE', #16816, #15478 ) ;
#9449=CARTESIAN_POINT ( 'NONE',  ( -90.06393689865117835, 72.00000000000000000, 59.85988923254397065 ) ) ;
#9456=CARTESIAN_POINT ( 'NONE',  ( 93.21002351426731991, 79.82103140525720164, 28.79774562292276840 ) ) ;
#9462=CARTESIAN_POINT ( 'NONE',  ( 90.82246629754762068, 169.9999999999999716, -1.173900486973974200 ) ) ;
#9464=CARTESIAN_POINT ( 'NONE',  ( 105.4076409534521446, 69.99999999999998579, -33.36508996883003419 ) ) ;
#9470=DIRECTION ( 'NONE',  ( 0.01292414190464131682, 0.000000000000000000, 0.9999164797902017066 ) ) ;
#9471=CARTESIAN_POINT ( 'NONE',  ( 76.10617011087394701, 75.05943625219154569, -4.352187486329626154 ) ) ;
#9486=CARTESIAN_POINT ( 'NONE',  ( 91.92966151681221731, 79.05204536692269812, -28.63995821788549279 ) ) ;
#9488=CARTESIAN_POINT ( 'NONE',  ( 1.163172771417732010, 45.00000000000000000, 89.99248318111813205 ) ) ;
#9493=EDGE_LOOP ( 'NONE', ( #19762, #21579, #19698, #11999, #7179, #20560 ) ) ;
#9498=ADVANCED_FACE ( 'NONE', ( #8410 ), #16414, .T. ) ;
#9512=CARTESIAN_POINT ( 'NONE',  ( 82.94572876491719171, 105.0000000000000000, -72.24960954674284608 ) ) ;
#9516=VERTEX_POINT ( 'NONE', #10595 ) ;
#9521=CARTESIAN_POINT ( 'NONE',  ( -18.68000515982659948, 88.26848370977704406, 77.55425219113827495 ) ) ;
#9531=CARTESIAN_POINT ( 'NONE',  ( -89.46067271499279627, 89.11592295107170969, 51.60461869884851183 ) ) ;
#9537=LINE ( 'NONE', #20086, #19854 ) ;
#9549=ORIENTED_EDGE ( 'NONE', *, *, #6112, .T. ) ;
#9551=CARTESIAN_POINT ( 'NONE',  ( -93.06424251235314671, 77.12912189496638860, -28.79962987465164304 ) ) ;
#9557=DIRECTION ( 'NONE',  ( -0.009985269297354625040, -0.6348858185549794975, -0.7725414498878574454 ) ) ;
#9560=VERTEX_POINT ( 'NONE', #8735 ) ;
#9561=LINE ( 'NONE', #16596, #15727 ) ;
#9562=EDGE_CURVE ( 'NONE', #367, #16244, #8967, .T. ) ;
#9563=ORIENTED_EDGE ( 'NONE', *, *, #5379, .T. ) ;
#9565=AXIS2_PLACEMENT_3D ( 'NONE', #8325, #1240, #22640 ) ;
#9566=CARTESIAN_POINT ( 'NONE',  ( -83.31183079427971450, 75.07749829403635999, 4.920832620970953641 ) ) ;
#9568=CARTESIAN_POINT ( 'NONE',  ( -88.16163815486164879, 88.05173128619230738, 53.06165861546533336 ) ) ;
#9572=ORIENTED_EDGE ( 'NONE', *, *, #17774, .F. ) ;
#9577=CARTESIAN_POINT ( 'NONE',  ( -41.58451242677340076, 92.58578643762699301, -83.88377541325534992 ) ) ;
#9581=EDGE_CURVE ( 'NONE', #6852, #5956, #15258, .T. ) ;
#9586=AXIS2_PLACEMENT_3D ( 'NONE', #18114, #20255, #4518 ) ;
#9588=ORIENTED_EDGE ( 'NONE', *, *, #18628, .F. ) ;
#9595=CARTESIAN_POINT ( 'NONE',  ( -90.17340641399441381, 87.01242838177741135, 51.39043932755232902 ) ) ;
#9600=VECTOR ( 'NONE', #8529, 1000.000000000000000 ) ;
#9607=EDGE_CURVE ( 'NONE', #17671, #10325, #6916, .T. ) ;
#9610=VERTEX_POINT ( 'NONE', #12227 ) ;
#9614=DIRECTION ( 'NONE',  ( 2.025474946048326158E-22, -1.000000000000000000, 1.876735158486679638E-22 ) ) ;
#9616=CARTESIAN_POINT ( 'NONE',  ( 68.71681667565954399, 72.00000000000000000, -85.89527988174788220 ) ) ;
#9618=CARTESIAN_POINT ( 'NONE',  ( 92.60113547278147905, 70.26667278203287026, 59.37223626620095729 ) ) ;
#9619=ORIENTED_EDGE ( 'NONE', *, *, #3728, .F. ) ;
#9623=DIRECTION ( 'NONE',  ( 0.01292414190464131682, 1.902755938799531179E-22, 0.9999164797902017066 ) ) ;
#9627=VERTEX_POINT ( 'NONE', #15566 ) ;
#9629=CARTESIAN_POINT ( 'NONE',  ( -64.03197570747913403, 99.62212517233105302, 75.31426563926737572 ) ) ;
#9639=ADVANCED_FACE ( 'NONE', ( #2201 ), #157, .F. ) ;
#9652=DIRECTION ( 'NONE',  ( -2.025474946048326158E-22, 1.000000000000000000, -1.876735158486679638E-22 ) ) ;
#9656=CARTESIAN_POINT ( 'NONE',  ( -89.84471876097053666, 87.96141862524974897, 50.80991467805918660 ) ) ;
#9661=EDGE_LOOP ( 'NONE', ( #9185, #11093 ) ) ;
#9667=AXIS2_PLACEMENT_3D ( 'NONE', #6413, #9848, #18912 ) ;
#9680=CARTESIAN_POINT ( 'NONE',  ( 88.82263333796723259, 169.9999999999999716, -1.148052203164690033 ) ) ;
#9685=ORIENTED_EDGE ( 'NONE', *, *, #106, .T. ) ;
#9686=AXIS2_PLACEMENT_3D ( 'NONE', #20114, #13050, #21942 ) ;
#9690=CARTESIAN_POINT ( 'NONE',  ( -90.17158066196779487, 87.09867769988316866, 51.33820610053523126 ) ) ;
#9698=CARTESIAN_POINT ( 'NONE',  ( -89.78684647853550871, 79.34753190266584966, 29.57356476272790502 ) ) ;
#9699=LINE ( 'NONE', #13263, #6915 ) ;
#9712=FACE_OUTER_BOUND ( 'NONE', #10651, .T. ) ;
#9717=ORIENTED_EDGE ( 'NONE', *, *, #10409, .F. ) ;
#9719=DIRECTION ( 'NONE',  ( -2.025474946048326158E-22, 1.000000000000000000, -1.876735158486679638E-22 ) ) ;
#9726=CARTESIAN_POINT ( 'NONE',  ( 79.39526044036306018, 75.13524200571961842, 4.041958712526196429 ) ) ;
#9727=FACE_OUTER_BOUND ( 'NONE', #236, .T. ) ;
#9731=ORIENTED_EDGE ( 'NONE', *, *, #14599, .T. ) ;
#9732=CARTESIAN_POINT ( 'NONE',  ( -68.99891043397279589, 92.11203426037263853, 85.66888312730651478 ) ) ;
#9735=CARTESIAN_POINT ( 'NONE',  ( -67.12230846849016075, 89.94961994313915454, 67.62393891741413654 ) ) ;
#9767=DIRECTION ( 'NONE',  ( 2.025474946048326158E-22, -1.000000000000000000, 1.876735158486679638E-22 ) ) ;
#9777=CARTESIAN_POINT ( 'NONE',  ( 65.90110554552377664, 105.0000000000000000, 69.29678410920483600 ) ) ;
#9783=ORIENTED_EDGE ( 'NONE', *, *, #11663, .T. ) ;
#9785=CARTESIAN_POINT ( 'NONE',  ( -80.22026031257210832, 86.08487693883552083, 75.35739733108806604 ) ) ;
#9796=CARTESIAN_POINT ( 'NONE',  ( -88.16332400514416179, 88.24736152454507021, 52.92523720185091207 ) ) ;
#9800=EDGE_LOOP ( 'NONE', ( #18155, #21025, #3160, #9313 ) ) ;
#9801=ORIENTED_EDGE ( 'NONE', *, *, #14709, .T. ) ;
#9805=CARTESIAN_POINT ( 'NONE',  ( -88.44888535621197434, 80.14369956782289250, 31.98268552584471180 ) ) ;
#9814=ADVANCED_FACE ( 'NONE', ( #6219 ), #18845, .T. ) ;
#9827=CARTESIAN_POINT ( 'NONE',  ( 105.5454984634617972, 78.31265485325668863, -30.98643060412782546 ) ) ;
#9831=DIRECTION ( 'NONE',  ( -0.01292414190464217898, -1.902755938799531885E-22, -0.9999164797902015955 ) ) ;
#9834=CARTESIAN_POINT ( 'NONE',  ( 68.71681667565957241, 71.82428002877155393, -85.89527988174788220 ) ) ;
#9836=EDGE_CURVE ( 'NONE', #3588, #5713, #3498, .T. ) ;
#9837=CYLINDRICAL_SURFACE ( 'NONE', #11111, 1.990000000000003988 ) ;
#9840=DIRECTION ( 'NONE',  ( -0.01292414190463830014, 0.000000000000000000, -0.9999164797902017066 ) ) ;
#9844=ORIENTED_EDGE ( 'NONE', *, *, #10659, .F. ) ;
#9848=DIRECTION ( 'NONE',  ( 2.025474946048326158E-22, -1.000000000000000000, 1.876735158486679638E-22 ) ) ;
#9857=CYLINDRICAL_SURFACE ( 'NONE', #17325, 5.099999999999992539 ) ;
#9861=VERTEX_POINT ( 'NONE', #20343 ) ;
#9864=CARTESIAN_POINT ( 'NONE',  ( -2.067862704742604141, 69.99999999999998579, -159.9866367664322979 ) ) ;
#9869=DIRECTION ( 'NONE',  ( -0.01292414190464131508, -1.902755938799530474E-22, -0.9999164797902017066 ) ) ;
#9875=LINE ( 'NONE', #11713, #19874 ) ;
#9879=CYLINDRICAL_SURFACE ( 'NONE', #13438, 2.000000000000004885 ) ;
#9887=CARTESIAN_POINT ( 'NONE',  ( -83.92517094583074311, 79.85565591775390715, 71.13418697079595177 ) ) ;
#9888=CARTESIAN_POINT ( 'NONE',  ( 105.7941983518663136, 70.06152065884126046, 30.12648231254615894 ) ) ;
#9894=CARTESIAN_POINT ( 'NONE',  ( 90.43474204040840903, 34.61572286322119396, -31.17139488068002251 ) ) ;
#9902=CARTESIAN_POINT ( 'NONE',  ( -90.11148781677563591, 87.44634235373453635, 51.12665407066659640 ) ) ;
#9908=CARTESIAN_POINT ( 'NONE',  ( -74.46989193151192410, 95.80563795305937447, 80.95834026808688577 ) ) ;
#9918=CARTESIAN_POINT ( 'NONE',  ( 92.19968689859011590, 79.04398536104956463, -28.61667231988791826 ) ) ;
#9922=DIRECTION ( 'NONE',  ( -0.01292414190463827932, 0.000000000000000000, -0.9999164797902018176 ) ) ;
#9930=EDGE_CURVE ( 'NONE', #12065, #17671, #12317, .T. ) ;
#9932=CIRCLE ( 'NONE', #12872, 2.000000000000004885 ) ;
#9934=VERTEX_POINT ( 'NONE', #20677 ) ;
#9939=CARTESIAN_POINT ( 'NONE',  ( -0.9693106428480922077, 72.00000000000000000, -74.99373598426512899 ) ) ;
#9946=DIRECTION ( 'NONE',  ( 0.9999164797902017066, 2.001050586450177050E-22, -0.01292414190464218071 ) ) ;
#9951=AXIS2_PLACEMENT_3D ( 'NONE', #14349, #19596, #10881 ) ;
#9953=CARTESIAN_POINT ( 'NONE',  ( 91.81287659828484493, 71.13119029400844795, 60.58394261007850901 ) ) ;
#9955=VERTEX_POINT ( 'NONE', #18950 ) ;
#9961=ORIENTED_EDGE ( 'NONE', *, *, #5120, .T. ) ;
#9965=DIRECTION ( 'NONE',  ( 0.01292414190463953873, 0.000000000000000000, 0.9999164797902017066 ) ) ;
#9971=AXIS2_PLACEMENT_3D ( 'NONE', #17004, #20406, #11480 ) ;
#9976=CARTESIAN_POINT ( 'NONE',  ( -90.43474204040838060, 72.00000000000000000, 31.17139488067998343 ) ) ;
#9978=CARTESIAN_POINT ( 'NONE',  ( -1.247179693797872524, 44.99899999999999523, -96.49194029975447506 ) ) ;
#9981=CARTESIAN_POINT ( 'NONE',  ( -88.74294073166163344, 70.70905333810220839, 62.85632276041776123 ) ) ;
#9997=DIRECTION ( 'NONE',  ( -0.9999164797902017066, -2.001050586450178931E-22, 0.01292414190464131508 ) ) ;
#9999=CARTESIAN_POINT ( 'NONE',  ( 64.08803682720244410, 103.0000000000000000, -70.97692255680823337 ) ) ;
#10003=ORIENTED_EDGE ( 'NONE', *, *, #10761, .F. ) ;
#10004=CARTESIAN_POINT ( 'NONE',  ( -73.00030478232707765, 95.66452290628956234, 82.28581592040848136 ) ) ;
#10008=CARTESIAN_POINT ( 'NONE',  ( 105.9308899693960626, 70.24357031783570449, 29.64301131075924545 ) ) ;
#10022=CARTESIAN_POINT ( 'NONE',  ( -90.08534597741504513, 88.53258948335707146, 52.71256580331551334 ) ) ;
#10025=ORIENTED_EDGE ( 'NONE', *, *, #12368, .T. ) ;
#10027=B_SPLINE_CURVE_WITH_KNOTS ( 'NONE', 3,
 ( #13741, #20608, #13410, #11787, #6716, #20488, #15253, #11903, #10279, #13844, #8425, #22206, #1555, #5086 ),
 .UNSPECIFIED., .F., .F.,
 ( 4, 2, 2, 2, 2, 2, 4 ),
 ( 0.000000000000000000, 0.001119727475084575678, 0.001679591212626860156, 0.002239454950169144417, 0.003359182425253676510, 0.003919046162795964891, 0.004478909900338253272 ),
 .UNSPECIFIED. ) ;
#10028=CARTESIAN_POINT ( 'NONE',  ( -72.51438462527775641, 87.23323244114081376, 69.92599951943640235 ) ) ;
#10029=CARTESIAN_POINT ( 'NONE',  ( -75.38289248423089361, 96.35610324583468866, 81.62497328870777835 ) ) ;
#10031=DIRECTION ( 'NONE',  ( -2.025474946048326158E-22, 1.000000000000000000, -1.876735158486679638E-22 ) ) ;
#10033=CARTESIAN_POINT ( 'NONE',  ( -71.43040806848136981, 92.41825753590678971, -83.65230687350626226 ) ) ;
#10040=EDGE_CURVE ( 'NONE', #20154, #13967, #7398, .T. ) ;
#10045=CARTESIAN_POINT ( 'NONE',  ( -64.02612899542262426, 99.97194305692366356, 75.76661472217124071 ) ) ;
#10063=AXIS2_PLACEMENT_3D ( 'NONE', #57, #13848, #3387 ) ;
#10070=DIRECTION ( 'NONE',  ( 5.257939330034138471E-16, 1.000000000000000000, -6.796193297819532347E-18 ) ) ;
#10084=DIRECTION ( 'NONE',  ( 0.9999164797902017066, 2.001050586450178931E-22, -0.01292414190464131508 ) ) ;
#10091=AXIS2_PLACEMENT_3D ( 'NONE', #2104, #12693, #1766 ) ;
#10095=LINE ( 'NONE', #9976, #17425 ) ;
#10097=VERTEX_POINT ( 'NONE', #9981 ) ;
#10099=EDGE_CURVE ( 'NONE', #21379, #4157, #19267, .T. ) ;
#10113=VERTEX_POINT ( 'NONE', #13335 ) ;
#10120=EDGE_LOOP ( 'NONE', ( #988, #709, #12775, #10725 ) ) ;
#10126=DIRECTION ( 'NONE',  ( -2.025474946048326158E-22, 1.000000000000000000, -1.876735158486679638E-22 ) ) ;
#10130=CARTESIAN_POINT ( 'NONE',  ( -39.42082737383930890, 91.17157287525388654, 83.51645567887777588 ) ) ;
#10132=VERTEX_POINT ( 'NONE', #4667 ) ;
#10135=CARTESIAN_POINT ( 'NONE',  ( -89.95810659785270502, 88.78972713510226811, 52.40189527015975557 ) ) ;
#10136=ORIENTED_EDGE ( 'NONE', *, *, #18770, .T. ) ;
#10140=CARTESIAN_POINT ( 'NONE',  ( -64.35900422130245602, 88.71869973106718987, 50.01268641288888972 ) ) ;
#10143=B_SPLINE_CURVE_WITH_KNOTS ( 'NONE', 3,
 ( #19744, #9190, #16240, #21247, #12771, #13019, #5515, #11269, #7589, #4015, #11042, #2314, #19540, #9419, #17851, #16459 ),
 .UNSPECIFIED., .F., .F.,
 ( 4, 2, 2, 2, 2, 2, 2, 4 ),
 ( 0.000000000000000000, 0.0003989315947993856814, 0.0007978631895987713628, 0.001196794784398157044, 0.001595726379197542726, 0.002393589568796313221, 0.002792521163595688711, 0.003191452758395064201 ),
 .UNSPECIFIED. ) ;
#10151=CARTESIAN_POINT ( 'NONE',  ( 89.78684647853556555, 79.34753190266587808, -29.57356476272795121 ) ) ;
#10157=VERTEX_POINT ( 'NONE', #11597 ) ;
#10162=CARTESIAN_POINT ( 'NONE',  ( -89.95770071757259245, 72.76905099204731187, 61.70965611469623013 ) ) ;
#10171=CARTESIAN_POINT ( 'NONE',  ( 88.41758806590425479, 80.31838830481380853, -32.48564084813598640 ) ) ;
#10175=EDGE_CURVE ( 'NONE', #6510, #15210, #15290, .T. ) ;
#10179=EDGE_LOOP ( 'NONE', ( #14583, #11961, #18276, #15629, #11997, #19181, #5404, #8877, #18888 ) ) ;
#10180=LINE ( 'NONE', #15489, #19371 ) ;
#10181=VERTEX_POINT ( 'NONE', #8258 ) ;
#10183=CARTESIAN_POINT ( 'NONE',  ( 1.364374644014609697E-14, 69.99999999999998579, -9.836443712999143722E-15 ) ) ;
#10184=ADVANCED_FACE ( 'NONE', ( #16884, #2853, #1148 ), #11701, .F. ) ;
#10187=CARTESIAN_POINT ( 'NONE',  ( -90.00466877033377955, 70.05991977044968166, 63.23890890537643372 ) ) ;
#10193=CIRCLE ( 'NONE', #5400, 110.0000000000000000 ) ;
#10210=FACE_OUTER_BOUND ( 'NONE', #18589, .T. ) ;
#10213=EDGE_CURVE ( 'NONE', #13377, #8239, #20074, .T. ) ;
#10224=DIRECTION ( 'NONE',  ( -2.025474946048326158E-22, 1.000000000000000000, -1.876735158486679638E-22 ) ) ;
#10228=( NAMED_UNIT ( * ) SI_UNIT ( $, .STERADIAN. ) SOLID_ANGLE_UNIT ( ) );
#10229=CARTESIAN_POINT ( 'NONE',  ( 106.2343493168401665, 77.75544475269074951, 28.53532068555786694 ) ) ;
#10230=CARTESIAN_POINT ( 'NONE',  ( 105.6473595942261738, 69.99999999999998579, 30.63715735456338862 ) ) ;
#10237=CARTESIAN_POINT ( 'NONE',  ( -90.02055463237803679, 34.61572286322119396, 63.21629334023816682 ) ) ;
#10240=CARTESIAN_POINT ( 'NONE',  ( 91.23431456517670313, 70.15875158948053070, -61.45272182677553729 ) ) ;
#10241=CARTESIAN_POINT ( 'NONE',  ( -88.16520156323190349, 88.42903772351857583, 52.76279105450071683 ) ) ;
#10246=DIRECTION ( 'NONE',  ( 5.257939330034138471E-16, 1.000000000000000000, -6.796193297819532347E-18 ) ) ;
#10247=VERTEX_POINT ( 'NONE', #5058 ) ;
#10253=ORIENTED_EDGE ( 'NONE', *, *, #7356, .T. ) ;
#10257=FACE_OUTER_BOUND ( 'NONE', #6272, .T. ) ;
#10258=DIRECTION ( 'NONE',  ( 0.9999164797902017066, 2.001050586450178931E-22, -0.01292414190464131508 ) ) ;
#10260=EDGE_CURVE ( 'NONE', #5580, #20892, #14171, .T. ) ;
#10270=VECTOR ( 'NONE', #9652, 1000.000000000000000 ) ;
#10276=CARTESIAN_POINT ( 'NONE',  ( -88.26117087638380099, 71.62891547111030377, 62.33105731329421673 ) ) ;
#10277=EDGE_CURVE ( 'NONE', #899, #20716, #7408, .T. ) ;
#10279=CARTESIAN_POINT ( 'NONE',  ( -92.03665420188171709, 70.73625599351603910, -60.24390366714261802 ) ) ;
#10282=DIRECTION ( 'NONE',  ( -0.9999164797902015955, -2.001050586450181282E-22, 0.01292414190463992731 ) ) ;
#10283=CARTESIAN_POINT ( 'NONE',  ( -0.9693106428480923187, 86.14745084375785211, -74.99373598426512899 ) ) ;
#10288=CARTESIAN_POINT ( 'NONE',  ( 88.44788333809653125, 80.14655074237849419, -31.99095626761635458 ) ) ;
#10301=VECTOR ( 'NONE', #331, 1000.000000000000000 ) ;
#10309=CYLINDRICAL_SURFACE ( 'NONE', #1280, 85.00000000000002842 ) ;
#10311=CARTESIAN_POINT ( 'NONE',  ( 108.2112308668079521, 76.78797451630624948, -19.89137302265093510 ) ) ;
#10315=CIRCLE ( 'NONE', #15849, 97.00000000000005684 ) ;
#10318=DIRECTION ( 'NONE',  ( -0.01292414190464131335, -1.902755938799530239E-22, -0.9999164797902015955 ) ) ;
#10325=VERTEX_POINT ( 'NONE', #21577 ) ;
#10327=CARTESIAN_POINT ( 'NONE',  ( -66.18268079339598842, 69.99999999999998579, 87.86269266872857031 ) ) ;
#10332=VERTEX_POINT ( 'NONE', #829 ) ;
#10339=LINE ( 'NONE', #6766, #14436 ) ;
#10342=CARTESIAN_POINT ( 'NONE',  ( -88.18357261921191537, 87.01242838177741135, 51.36472028516209321 ) ) ;
#10352=CARTESIAN_POINT ( 'NONE',  ( 84.66199002107499894, 104.7463091522047733, -70.23140500867290825 ) ) ;
#10356=ORIENTED_EDGE ( 'NONE', *, *, #15664, .F. ) ;
#10361=CARTESIAN_POINT ( 'NONE',  ( -79.99331838321612054, 55.00000000000000000, 1.033931352371344481 ) ) ;
#10362=CARTESIAN_POINT ( 'NONE',  ( -90.13526681931318763, 87.35670873163414285, 51.18135378728248952 ) ) ;
#10367=EDGE_CURVE ( 'NONE', #8624, #5449, #17843, .T. ) ;
#10370=DIRECTION ( 'NONE',  ( -0.01292414190463830014, 0.000000000000000000, -0.9999164797902017066 ) ) ;
#10373=TOROIDAL_SURFACE ( 'NONE', #14054, 4.000000000000000000, 2.000000000000000000 ) ;
#10374=CARTESIAN_POINT ( 'NONE',  ( 90.43474204040840903, 72.00000000000000000, -31.17139488068002251 ) ) ;
#10375=ORIENTED_EDGE ( 'NONE', *, *, #7786, .T. ) ;
#10379=CARTESIAN_POINT ( 'NONE',  ( 88.83250513209151222, 79.73807450349755754, -30.77911165157509643 ) ) ;
#10380=DIRECTION ( 'NONE',  ( -0.01292414190463827932, 0.000000000000000000, -0.9999164797902018176 ) ) ;
#10384=CARTESIAN_POINT ( 'NONE',  ( 105.1935855565140088, 70.39579207655377502, -32.16088115703477968 ) ) ;
#10385=EDGE_CURVE ( 'NONE', #21648, #16549, #10143, .T. ) ;
#10386=CARTESIAN_POINT ( 'NONE',  ( -63.99469827093767549, 99.63525711781676364, 78.19835058642853198 ) ) ;
#10387=VERTEX_POINT ( 'NONE', #4132 ) ;
#10391=DIRECTION ( 'NONE',  ( -0.01292414190463832269, 0.000000000000000000, -0.9999164797902017066 ) ) ;
#10396=DIRECTION ( 'NONE',  ( -2.025474946048326158E-22, 1.000000000000000000, -1.876735158486679638E-22 ) ) ;
#10404=CARTESIAN_POINT ( 'NONE',  ( 90.51365344713448735, 78.00107869518899406, -32.54507930669857529 ) ) ;
#10409=EDGE_CURVE ( 'NONE', #8789, #3455, #10826, .T. ) ;
#10413=DIRECTION ( 'NONE',  ( 0.01292414190464131335, 0.000000000000000000, 0.9999164797902017066 ) ) ;
#10423=ORIENTED_EDGE ( 'NONE', *, *, #21843, .F. ) ;
#10436=DIRECTION ( 'NONE',  ( -0.8909995034498461308, -2.656742962652179567E-22, -0.4540042784513463880 ) ) ;
#10441=DIRECTION ( 'NONE',  ( -0.004263634442766563518, 0.9440169652124856814, -0.3298693541575922761 ) ) ;
#10444=FACE_OUTER_BOUND ( 'NONE', #12490, .T. ) ;
#10450=VERTEX_POINT ( 'NONE', #13233 ) ;
#10457=CARTESIAN_POINT ( 'NONE',  ( 106.3114127004272689, 78.31407127224935039, 28.24702759725663270 ) ) ;
#10459=CARTESIAN_POINT ( 'NONE',  ( 105.4334892372614405, 72.00000000000000000, -31.36525700924962834 ) ) ;
#10460=DIRECTION ( 'NONE',  ( 0.4654428868037304712, -0.8850574712643681785, -0.006015952371159197752 ) ) ;
#10463=CARTESIAN_POINT ( 'NONE',  ( 84.25113090574824071, 104.9515410254813759, -70.72375658096314055 ) ) ;
#10468=EDGE_CURVE ( 'NONE', #495, #591, #8289, .T. ) ;
#10470=B_SPLINE_CURVE_WITH_KNOTS ( 'NONE', 3,
 ( #3041, #15470, #17078, #18561, #6715, #2819, #9827, #16845, #8100, #18660, #15136, #22085, #13408, #20379, #8752, #14201 ),
 .UNSPECIFIED., .F., .F.,
 ( 4, 2, 2, 2, 2, 2, 2, 4 ),
 ( 0.000000000000000000, 0.0004728798714925855047, 0.0009457597429851710095, 0.001418639614477756623, 0.001891519485970342019, 0.002364399357462927415, 0.002837279228955513245, 0.003783038971940663221 ),
 .UNSPECIFIED. ) ;
#10471=B_SPLINE_CURVE_WITH_KNOTS ( 'NONE', 3,
 ( #18148, #16533, #786, #7782, #18343, #2617, #9629 ),
 .UNSPECIFIED., .F., .F.,
 ( 4, 3, 4 ),
 ( 3.399349888776295571E-17, 0.004000000000097216589, 0.01315492597274157613 ),
 .UNSPECIFIED. ) ;
#10473=CARTESIAN_POINT ( 'NONE',  ( -88.16724451997782808, 88.59287701227550826, 52.57531193446310880 ) ) ;
#10474=DIRECTION ( 'NONE',  ( -0.9999164797902015955, -2.001050586450178695E-22, 0.01292414190464131335 ) ) ;
#10481=DIRECTION ( 'NONE',  ( 0.9999164797902017066, 2.001050586450181517E-22, -0.01292414190463992731 ) ) ;
#10484=CARTESIAN_POINT ( 'NONE',  ( 85.08844994865407330, 75.00000638978997358, -1.434341340840276091 ) ) ;
#10490=CARTESIAN_POINT ( 'NONE',  ( -76.93671954797112278, 75.08645580250139062, -3.062200394342287080 ) ) ;
#10492=CARTESIAN_POINT ( 'NONE',  ( -106.1636641531658398, 79.04398536104955042, 28.79715981783285628 ) ) ;
#10496=CARTESIAN_POINT ( 'NONE',  ( 104.8202145123290876, 69.99999999999998579, -33.35749735200946731 ) ) ;
#10505=ADVANCED_FACE ( 'NONE', ( #2868 ), #9879, .F. ) ;
#10508=PLANE ( 'NONE',  #12426 ) ;
#10511=CARTESIAN_POINT ( 'NONE',  ( 64.10672825728823909, 104.3814432989690602, -69.53080186952975339 ) ) ;
#10516=CARTESIAN_POINT ( 'NONE',  ( 90.14522075562641135, 79.46791348803257904, 27.62924625256333044 ) ) ;
#10517=CARTESIAN_POINT ( 'NONE',  ( -110.8973471360828285, 103.0000000000000000, -68.71519772349600430 ) ) ;
#10519=CARTESIAN_POINT ( 'NONE',  ( 91.62437796271727564, 95.44063823554748183, 60.86849236629024773 ) ) ;
#10524=CARTESIAN_POINT ( 'NONE',  ( -92.55117574443677597, 77.19412514573775752, -28.91372802644275453 ) ) ;
#10525=ORIENTED_EDGE ( 'NONE', *, *, #21536, .F. ) ;
#10528=CARTESIAN_POINT ( 'NONE',  ( 1.364374644014609697E-14, 69.99999999999998579, -9.836443712999143722E-15 ) ) ;
#10533=ORIENTED_EDGE ( 'NONE', *, *, #219, .T. ) ;
#10539=PLANE ( 'NONE',  #18397 ) ;
#10540=ORIENTED_EDGE ( 'NONE', *, *, #58, .T. ) ;
#10542=CARTESIAN_POINT ( 'NONE',  ( -90.50186546057693704, 78.02565673216736286, 32.58161589089091592 ) ) ;
#10559=CARTESIAN_POINT ( 'NONE',  ( 92.40872671617952960, 72.00000000000000000, -33.19707612406970298 ) ) ;
#10561=ORIENTED_EDGE ( 'NONE', *, *, #3162, .T. ) ;
#10564=ORIENTED_EDGE ( 'NONE', *, *, #7116, .F. ) ;
#10570=DIRECTION ( 'NONE',  ( 0.01292414190464131508, 1.902755938799530474E-22, 0.9999164797902017066 ) ) ;
#10571=CIRCLE ( 'NONE', #6882, 95.00000000000004263 ) ;
#10574=AXIS2_PLACEMENT_3D ( 'NONE', #12911, #7606, #2332 ) ;
#10576=CARTESIAN_POINT ( 'NONE',  ( -88.16661084868957232, 88.54544711483490005, 52.63461214281247891 ) ) ;
#10583=CARTESIAN_POINT ( 'NONE',  ( 80.26441115539796556, 75.13699351169600504, -6.137861275126254235 ) ) ;
#10589=CARTESIAN_POINT ( 'NONE',  ( -76.67152933958324468, 75.07738311394996344, -2.850188674051770121 ) ) ;
#10591=AXIS2_PLACEMENT_3D ( 'NONE', #14652, #739, #861 ) ;
#10595=CARTESIAN_POINT ( 'NONE',  ( 1.121675378414705104, 55.00000000000000000, 109.9942809619911799 ) ) ;
#10596=CIRCLE ( 'NONE', #699, 2.000000000000000000 ) ;
#10598=ORIENTED_EDGE ( 'NONE', *, *, #21123, .T. ) ;
#10604=EDGE_CURVE ( 'NONE', #8847, #10113, #11974, .T. ) ;
#10606=ORIENTED_EDGE ( 'NONE', *, *, #19735, .T. ) ;
#10607=ORIENTED_EDGE ( 'NONE', *, *, #18084, .F. ) ;
#10613=DIRECTION ( 'NONE',  ( 0.01292414190464131335, 0.000000000000000000, 0.9999164797902017066 ) ) ;
#10619=DIRECTION ( 'NONE',  ( -0.01292414190463827932, 0.000000000000000000, -0.9999164797902018176 ) ) ;
#10622=CARTESIAN_POINT ( 'NONE',  ( 90.82246629754764911, 169.9999999999999716, -1.173900486973972868 ) ) ;
#10626=CARTESIAN_POINT ( 'NONE',  ( -92.88576702167225108, 79.82922271357917055, -28.81576165492124986 ) ) ;
#10630=CARTESIAN_POINT ( 'NONE',  ( -68.97076059960821226, 70.03291683438813209, -85.69217454375159093 ) ) ;
#10636=VECTOR ( 'NONE', #13267, 1000.000000000000114 ) ;
#10639=VERTEX_POINT ( 'NONE', #12183 ) ;
#10645=AXIS2_PLACEMENT_3D ( 'NONE', #18817, #17109, #3420 ) ;
#10651=EDGE_LOOP ( 'NONE', ( #13928, #14563, #21119, #2784 ) ) ;
#10655=VECTOR ( 'NONE', #3942, 1000.000000000000000 ) ;
#10657=VECTOR ( 'NONE', #723, 1000.000000000000114 ) ;
#10659=EDGE_CURVE ( 'NONE', #18024, #9297, #6656, .T. ) ;
#10660=VECTOR ( 'NONE', #5481, 1000.000000000000114 ) ;
#10677=DIRECTION ( 'NONE',  ( -0.9999164797902017066, 1.387778780781447253E-14, 0.01292414190463832269 ) ) ;
#10682=ORIENTED_EDGE ( 'NONE', *, *, #17625, .T. ) ;
#10693=CARTESIAN_POINT ( 'NONE',  ( -88.16755730635141219, 88.61500917853037151, 52.54598585929731058 ) ) ;
#10702=CARTESIAN_POINT ( 'NONE',  ( 81.69827340936640780, 75.12327740397421394, 3.784263597974759641 ) ) ;
#10709=CARTESIAN_POINT ( 'NONE',  ( 1.364374644014609697E-14, 69.99999999999998579, -9.836443712999143722E-15 ) ) ;
#10710=CYLINDRICAL_SURFACE ( 'NONE', #14971, 2.000000000000001332 ) ;
#10715=CARTESIAN_POINT ( 'NONE',  ( -105.5195728421876282, 78.18109283220577765, 31.07451122637823815 ) ) ;
#10719=CARTESIAN_POINT ( 'NONE',  ( 395.1215762121263992, 103.0000000000000000, -76.28455149755049547 ) ) ;
#10722=CARTESIAN_POINT ( 'NONE',  ( -72.51438462527775641, 87.23323244114081376, 69.92599951943640235 ) ) ;
#10724=ORIENTED_EDGE ( 'NONE', *, *, #7950, .F. ) ;
#10725=ORIENTED_EDGE ( 'NONE', *, *, #8937, .F. ) ;
#10729=ORIENTED_EDGE ( 'NONE', *, *, #1938, .F. ) ;
#10731=AXIS2_PLACEMENT_3D ( 'NONE', #10977, #18745, #16403 ) ;
#10742=CARTESIAN_POINT ( 'NONE',  ( 92.88576702167598853, 79.82922271357915633, 28.81576165492026931 ) ) ;
#10744=B_SPLINE_CURVE_WITH_KNOTS ( 'NONE', 3,
 ( #6370, #17394, #13391, #22405 ),
 .UNSPECIFIED., .F., .F.,
 ( 4, 4 ),
 ( 0.03593651043649991050, 0.03600679027956682487 ),
 .UNSPECIFIED. ) ;
#10752=CARTESIAN_POINT ( 'NONE',  ( -91.47552206421207188, 77.76803451549854174, -29.83954006679693549 ) ) ;
#10758=AXIS2_PLACEMENT_3D ( 'NONE', #5920, #4076, #14679 ) ;
#10761=EDGE_CURVE ( 'NONE', #2857, #15210, #18350, .T. ) ;
#10770=CARTESIAN_POINT ( 'NONE',  ( -90.67285013207035149, 77.76891457534604513, 32.19520807900870807 ) ) ;
#10784=EDGE_CURVE ( 'NONE', #9371, #4637, #11465, .T. ) ;
#10787=DIRECTION ( 'NONE',  ( -0.9999164797902015955, -2.001050586450178695E-22, 0.01292414190464131335 ) ) ;
#10788=FACE_OUTER_BOUND ( 'NONE', #1293, .T. ) ;
#10795=ORIENTED_EDGE ( 'NONE', *, *, #1383, .F. ) ;
#10797=CIRCLE ( 'NONE', #19940, 6.499999999999998224 ) ;
#10799=CARTESIAN_POINT ( 'NONE',  ( 37.51181209962140883, 93.56461422141670425, -83.92720337889311111 ) ) ;
#10803=EDGE_CURVE ( 'NONE', #15344, #3120, #15944, .T. ) ;
#10807=DIRECTION ( 'NONE',  ( -2.459148776293844314E-24, 1.000000000000000000, -1.902597020224326827E-22 ) ) ;
#10810=DIRECTION ( 'NONE',  ( 0.9999164797902017066, 2.001050586450177285E-22, -0.01292414190464218071 ) ) ;
#10822=CARTESIAN_POINT ( 'NONE',  ( -88.16961949373364860, 88.74519938941557484, 52.34624730313399255 ) ) ;
#10826=LINE ( 'NONE', #11503, #7910 ) ;
#10827=DIRECTION ( 'NONE',  ( 0.008205354412248750534, -0.7726059781012502015, 0.6348327927582032570 ) ) ;
#10829=EDGE_CURVE ( 'NONE', #10951, #6274, #13718, .T. ) ;
#10830=CARTESIAN_POINT ( 'NONE',  ( 91.39645842968023715, 77.87428392844077507, 30.00278187767188243 ) ) ;
#10835=CARTESIAN_POINT ( 'NONE',  ( -75.98071139535758789, 75.05062594699535339, -2.131736981522680541 ) ) ;
#10837=CARTESIAN_POINT ( 'NONE',  ( -105.6376945813395594, 78.65441476617392880, 30.67074184297031536 ) ) ;
#10839=LINE ( 'NONE', #3482, #5214 ) ;
#10840=CARTESIAN_POINT ( 'NONE',  ( -40.65822637310711940, 91.17157287525390075, -84.25167897319539634 ) ) ;
#10850=CARTESIAN_POINT ( 'NONE',  ( -89.60390812178910380, 70.24399151081296111, 63.08126157891754104 ) ) ;
#10859=CARTESIAN_POINT ( 'NONE',  ( 91.28977804672281593, 78.08428866167092508, 30.31923231637453142 ) ) ;
#10863=LINE ( 'NONE', #8766, #18038 ) ;
#10878=CARTESIAN_POINT ( 'NONE',  ( 70.91392079944857585, 91.32005360614645895, 84.09052168258639881 ) ) ;
#10880=CARTESIAN_POINT ( 'NONE',  ( -91.18542874977060819, 79.95750479417183954, 31.50072335808886947 ) ) ;
#10881=DIRECTION ( 'NONE',  ( -0.01292414190463832269, 0.000000000000000000, -0.9999164797902017066 ) ) ;
#10895=CARTESIAN_POINT ( 'NONE',  ( -65.93268019054298179, 104.4142135623730923, -71.73965483371374319 ) ) ;
#10904=VERTEX_POINT ( 'NONE', #17085 ) ;
#10910=CARTESIAN_POINT ( 'NONE',  ( 30.69487628741233465, 91.18588819953914992, 79.89877478592977411 ) ) ;
#10916=ADVANCED_FACE ( 'NONE', ( #2930 ), #18566, .T. ) ;
#10917=VERTEX_POINT ( 'NONE', #10283 ) ;
#10920=CARTESIAN_POINT ( 'NONE',  ( -89.94033328634043301, 88.81992964173861083, 52.36201159483771761 ) ) ;
#10922=SHAPE_REPRESENTATION ( 'Upper Movable Jaw Swivel Housing', ( #6292 ), #8126 ) ;
#10926=CARTESIAN_POINT ( 'NONE',  ( 1.364373935098378649E-14, 105.0000000000000000, -9.836450281572198869E-15 ) ) ;
#10927=CARTESIAN_POINT ( 'NONE',  ( 64.08803682720245831, 105.0000000000000000, -70.97692255680823337 ) ) ;
#10930=CARTESIAN_POINT ( 'NONE',  ( 69.07678759757092735, 92.22190598759938496, -85.60612736256493349 ) ) ;
#10933=CARTESIAN_POINT ( 'NONE',  ( 91.82493316891849133, 77.47293851758952599, 29.37406230631716397 ) ) ;
#10936=CARTESIAN_POINT ( 'NONE',  ( -92.50752184771765485, 77.20349362929613335, -28.92971669647242905 ) ) ;
#10942=DIRECTION ( 'NONE',  ( 2.025474946048326158E-22, -1.000000000000000000, 1.876735158486679638E-22 ) ) ;
#10945=ORIENTED_EDGE ( 'NONE', *, *, #18426, .F. ) ;
#10946=CARTESIAN_POINT ( 'NONE',  ( -81.57403594986455175, 75.12325561942537888, 5.894141314586137881 ) ) ;
#10950=B_SPLINE_CURVE_WITH_KNOTS ( 'NONE', 3,
 ( #14571, #12958, #20041, #4194, #767, #9732, #11443, #7766, #16747, #14803 ),
 .UNSPECIFIED., .F., .F.,
 ( 4, 2, 2, 2, 4 ),
 ( 0.000000000000000000, 0.0004370559136044749457, 0.0008741118272089498913, 0.001311167740813424729, 0.001748223654417899783 ),
 .UNSPECIFIED. ) ;
#10951=VERTEX_POINT ( 'NONE', #13630 ) ;
#10962=CARTESIAN_POINT ( 'NONE',  ( 91.41775219751511372, 77.84255103198131565, 29.95431514106030590 ) ) ;
#10964=ORIENTED_EDGE ( 'NONE', *, *, #1017, .T. ) ;
#10966=PLANE ( 'NONE',  #1512 ) ;
#10969=CARTESIAN_POINT ( 'NONE',  ( -90.14522075562827297, 79.46791348803235167, -27.62924625256264122 ) ) ;
#10974=AXIS2_PLACEMENT_3D ( 'NONE', #7690, #19970, #696 ) ;
#10977=CARTESIAN_POINT ( 'NONE',  ( -92.40872671617950118, 72.00000000000000000, 33.19707612406966746 ) ) ;
#10985=CARTESIAN_POINT ( 'NONE',  ( 71.43040806848138402, 92.41825753590681813, 83.65230687350620542 ) ) ;
#10987=CARTESIAN_POINT ( 'NONE',  ( -90.90077733783158465, 77.56213813822601821, 31.87679858714241021 ) ) ;
#10998=ORIENTED_EDGE ( 'NONE', *, *, #19606, .T. ) ;
#11003=ORIENTED_EDGE ( 'NONE', *, *, #12120, .F. ) ;
#11011=VERTEX_POINT ( 'NONE', #16047 ) ;
#11020=EDGE_LOOP ( 'NONE', ( #6745, #13208, #3463, #15541 ) ) ;
#11022=B_SPLINE_CURVE_WITH_KNOTS ( 'NONE', 3,
 ( #18857, #19196, #20568, #5170, #11866, #1415, #15436, #12210, #9908, #18961, #3006, #22390, #1195, #3220, #6469, #13480 ),
 .UNSPECIFIED., .F., .F.,
 ( 4, 2, 2, 2, 2, 2, 2, 4 ),
 ( 0.000000000000000000, 0.0004395957642550035564, 0.0008791915285100071129, 0.001758383057019986470, 0.002197978821274975281, 0.002637574585529963659, 0.003077170349784952470, 0.003516766114039940848 ),
 .UNSPECIFIED. ) ;
#11042=CARTESIAN_POINT ( 'NONE',  ( -105.9308899693960484, 70.24357031783570449, -29.64301131075929518 ) ) ;
#11056=ORIENTED_EDGE ( 'NONE', *, *, #6468, .T. ) ;
#11066=CARTESIAN_POINT ( 'NONE',  ( -84.84767091729572996, 75.01394013563931651, -0.5387156272771348453 ) ) ;
#11067=CARTESIAN_POINT ( 'NONE',  ( -88.16184267143731290, 88.07739181906583781, 53.04568397887596376 ) ) ;
#11075=CARTESIAN_POINT ( 'NONE',  ( -39.45590449607104944, 92.86731729158431392, -83.62973377257371510 ) ) ;
#11080=CIRCLE ( 'NONE', #17311, 2.000000000000001332 ) ;
#11083=CARTESIAN_POINT ( 'NONE',  ( 1.364374644014609697E-14, 69.99999999999998579, -9.836443712999143722E-15 ) ) ;
#11084=EDGE_CURVE ( 'NONE', #198, #13705, #627, .T. ) ;
#11088=FACE_OUTER_BOUND ( 'NONE', #11272, .T. ) ;
#11091=LINE ( 'NONE', #9464, #9102 ) ;
#11092=ORIENTED_EDGE ( 'NONE', *, *, #19061, .T. ) ;
#11093=ORIENTED_EDGE ( 'NONE', *, *, #1948, .T. ) ;
#11097=ADVANCED_FACE ( 'NONE', ( #19669 ), #12805, .T. ) ;
#11101=CARTESIAN_POINT ( 'NONE',  ( 70.91392079944854743, 91.17157287525388654, 84.09052168258639881 ) ) ;
#11111=AXIS2_PLACEMENT_3D ( 'NONE', #21981, #8231, #6282 ) ;
#11112=CARTESIAN_POINT ( 'NONE',  ( 92.16545979397402277, 77.13735158510392864, -31.20743466190268833 ) ) ;
#11116=CARTESIAN_POINT ( 'NONE',  ( -92.19651396575542890, 79.04398536194661062, 28.61663131200403498 ) ) ;
#11118=ORIENTED_EDGE ( 'NONE', *, *, #18556, .T. ) ;
#11128=DIRECTION ( 'NONE',  ( 0.01292414190464131335, 1.902755938799530239E-22, 0.9999164797902015955 ) ) ;
#11135=FACE_OUTER_BOUND ( 'NONE', #3124, .T. ) ;
#11139=LINE ( 'NONE', #2847, #11820 ) ;
#11152=CARTESIAN_POINT ( 'NONE',  ( -89.85439142418879044, 87.94879146495189559, 50.81774004189161076 ) ) ;
#11158=DIRECTION ( 'NONE',  ( -0.9999164797902015955, -2.001050586450178695E-22, 0.01292414190464131335 ) ) ;
#11161=CARTESIAN_POINT ( 'NONE',  ( -35.39322062607227792, 92.77591188308414871, 83.66707218845635907 ) ) ;
#11162=ORIENTED_EDGE ( 'NONE', *, *, #18266, .T. ) ;
#11170=EDGE_CURVE ( 'NONE', #7316, #9279, #5626, .T. ) ;
#11171=SPHERICAL_SURFACE ( 'NONE', #13253, 2.000000000000000000 ) ;
#11180=EDGE_LOOP ( 'NONE', ( #4944, #12558, #4991, #15124 ) ) ;
#11184=CARTESIAN_POINT ( 'NONE',  ( -90.16570127241018895, 87.17484075746328642, 51.29199764768473813 ) ) ;
#11191=FACE_OUTER_BOUND ( 'NONE', #20256, .T. ) ;
#11192=FACE_OUTER_BOUND ( 'NONE', #4709, .T. ) ;
#11194=CARTESIAN_POINT ( 'NONE',  ( -89.40819020483021973, 79.89452498912720557, -28.94780723987650362 ) ) ;
#11196=VERTEX_POINT ( 'NONE', #6695 ) ;
#11197=LINE ( 'NONE', #397, #19073 ) ;
#11198=DIRECTION ( 'NONE',  ( 0.01292414190465215537, 0.000000000000000000, 0.9999164797902015955 ) ) ;
#11200=CARTESIAN_POINT ( 'NONE',  ( 5.208897394599592445, 86.29861661753390933, -75.24359988578153491 ) ) ;
#11204=( BOUNDED_CURVE ( )  B_SPLINE_CURVE ( 3, ( #11913, #21377, #13636, #3821 ),
 .UNSPECIFIED., .F., .T. ) 
 B_SPLINE_CURVE_WITH_KNOTS ( ( 4, 4 ),
 ( 0.6960171423055208084, 0.7385976378458812830 ),
 .UNSPECIFIED. ) 
 CURVE ( )  GEOMETRIC_REPRESENTATION_ITEM ( )  RATIONAL_B_SPLINE_CURVE ( ( 1.000000000000000000, 0.9998489141570392480, 0.9998489141570392480, 1.000000000000000000 ) ) 
 REPRESENTATION_ITEM ( '' )  );
#11207=CARTESIAN_POINT ( 'NONE',  ( -90.82246629754759226, 169.9999999999999716, 1.173900486973951773 ) ) ;
#11209=ORIENTED_EDGE ( 'NONE', *, *, #2179, .F. ) ;
#11217=CARTESIAN_POINT ( 'NONE',  ( 76.67480597215256921, 75.07749829403637420, 2.852969916228293101 ) ) ;
#11218=CARTESIAN_POINT ( 'NONE',  ( -89.89473308095314508, 71.83810385978752322, 62.23413549537023215 ) ) ;
#11224=CARTESIAN_POINT ( 'NONE',  ( 90.02055463237802257, 95.71211110526448351, -63.21629334023823077 ) ) ;
#11227=FACE_OUTER_BOUND ( 'NONE', #16117, .T. ) ;
#11229=CARTESIAN_POINT ( 'NONE',  ( -90.81765045018502747, 77.62753381201262926, 31.97827203367538473 ) ) ;
#11240=ORIENTED_EDGE ( 'NONE', *, *, #13853, .F. ) ;
#11243=CARTESIAN_POINT ( 'NONE',  ( 38.89810712971356566, 72.00000000000000000, -85.50986645835283184 ) ) ;
#11245=VERTEX_POINT ( 'NONE', #15449 ) ;
#11247=CARTESIAN_POINT ( 'NONE',  ( -92.40872671617950118, 34.61572286322119396, 33.19707612406966746 ) ) ;
#11250=ORIENTED_EDGE ( 'NONE', *, *, #5603, .T. ) ;
#11251=CARTESIAN_POINT ( 'NONE',  ( -106.7989984338461937, 79.11557862755601889, -26.34385626240375444 ) ) ;
#11255=CARTESIAN_POINT ( 'NONE',  ( -33.82085273160089400, 93.50464841319747222, 82.93470554904384073 ) ) ;
#11261=CARTESIAN_POINT ( 'NONE',  ( -88.17496191764027458, 88.96312264442134676, 51.79368639984505762 ) ) ;
#11262=EDGE_CURVE ( 'NONE', #4456, #10097, #11326, .T. ) ;
#11269=CARTESIAN_POINT ( 'NONE',  ( -106.0939156777172769, 70.76422767839098071, -29.05317630099631288 ) ) ;
#11270=DIRECTION ( 'NONE',  ( 0.4768814951561130555, 0.000000000000000000, 0.8789675987075236119 ) ) ;
#11272=EDGE_LOOP ( 'NONE', ( #5638, #5119, #14342, #2392 ) ) ;
#11273=CARTESIAN_POINT ( 'NONE',  ( 38.82295403925315469, 92.04141378167194887, -85.46747784716957597 ) ) ;
#11277=CARTESIAN_POINT ( 'NONE',  ( -91.82493316891843449, 77.47293851758952599, -29.37406230631722082 ) ) ;
#11278=LINE ( 'NONE', #5868, #2841 ) ;
#11281=DIRECTION ( 'NONE',  ( 0.8789675987075231678, 8.853465811791729457E-23, -0.4768814951561137772 ) ) ;
#11288=CARTESIAN_POINT ( 'NONE',  ( -82.74895026642346352, 75.09868225356439098, -3.260777892351517160 ) ) ;
#11290=CARTESIAN_POINT ( 'NONE',  ( -90.15234812386498220, 88.12764344393974625, 53.04178249888710184 ) ) ;
#11291=EDGE_CURVE ( 'NONE', #7202, #18705, #8303, .T. ) ;
#11293=AXIS2_PLACEMENT_3D ( 'NONE', #1051, #22038, #6341 ) ;
#11297=CARTESIAN_POINT ( 'NONE',  ( -40.65822637310712651, 91.17157287525390075, -84.25167897319538213 ) ) ;
#11298=B_SPLINE_CURVE_WITH_KNOTS ( 'NONE', 3,
 ( #4480, #4595, #9785, #9887, #20672, #16910, #16702, #1177 ),
 .UNSPECIFIED., .F., .F.,
 ( 4, 2, 2, 4 ),
 ( 0.002383014531731640628, 0.01915976248411578250, 0.02754813646030784824, 0.03593651043649991050 ),
 .UNSPECIFIED. ) ;
#11299=CARTESIAN_POINT ( 'NONE',  ( 69.49687660543776246, 70.17287388826144934, 85.26604680535983505 ) ) ;
#11300=VERTEX_POINT ( 'NONE', #20583 ) ;
#11301=ORIENTED_EDGE ( 'NONE', *, *, #11514, .T. ) ;
#11302=DIRECTION ( 'NONE',  ( -2.025474946048326158E-22, 1.000000000000000000, -1.876735158486679638E-22 ) ) ;
#11303=CARTESIAN_POINT ( 'NONE',  ( 41.12105953731187924, 69.99999999999998579, 86.47576806556189410 ) ) ;
#11307=ADVANCED_FACE ( 'NONE', ( #4841 ), #17035, .T. ) ;
#11309=ORIENTED_EDGE ( 'NONE', *, *, #21123, .F. ) ;
#11313=DIRECTION ( 'NONE',  ( -0.01292414190464216336, 1.716839728801787493E-15, -0.9999164797902015955 ) ) ;
#11318=DIRECTION ( 'NONE',  ( -0.9999164797902015955, -2.001050586450178695E-22, 0.01292414190464131335 ) ) ;
#11325=CARTESIAN_POINT ( 'NONE',  ( -68.43148148480358373, 69.99999999999998579, -86.12277481476654373 ) ) ;
#11326=( BOUNDED_CURVE ( )  B_SPLINE_CURVE ( 3, ( #22187, #16942, #11759, #20362 ),
 .UNSPECIFIED., .F., .T. ) 
 B_SPLINE_CURVE_WITH_KNOTS ( ( 4, 4 ),
 ( 4.712388980384688786, 5.317223215405117109 ),
 .UNSPECIFIED. ) 
 CURVE ( )  GEOMETRIC_REPRESENTATION_ITEM ( )  RATIONAL_B_SPLINE_CURVE ( ( 1.000000000000000000, 0.9697462613334437709, 0.9697462613334437709, 1.000000000000000000 ) ) 
 REPRESENTATION_ITEM ( '' )  );
#11333=CARTESIAN_POINT ( 'NONE',  ( 91.52572433156683473, 77.25800443875652945, -31.39760542763762174 ) ) ;
#11338=EDGE_CURVE ( 'NONE', #10325, #12065, #12253, .T. ) ;
#11342=ORIENTED_EDGE ( 'NONE', *, *, #10829, .T. ) ;
#11343=ORIENTED_EDGE ( 'NONE', *, *, #21564, .T. ) ;
#11344=DIRECTION ( 'NONE',  ( 2.025474946048326158E-22, -1.000000000000000000, 1.876735158486679638E-22 ) ) ;
#11350=CIRCLE ( 'NONE', #3266, 2.000000000000002665 ) ;
#11355=ORIENTED_EDGE ( 'NONE', *, *, #14869, .F. ) ;
#11359=DIRECTION ( 'NONE',  ( 0.9999164797902015955, 2.001050586450178695E-22, -0.01292414190464131335 ) ) ;
#11360=VERTEX_POINT ( 'NONE', #7149 ) ;
#11370=CARTESIAN_POINT ( 'NONE',  ( -89.19153677579346606, 89.12515160658807645, 51.27603402924245302 ) ) ;
#11382=VERTEX_POINT ( 'NONE', #15784 ) ;
#11386=CARTESIAN_POINT ( 'NONE',  ( -92.63999567227412513, 77.17622496481537553, -28.88303657775555067 ) ) ;
#11402=CARTESIAN_POINT ( 'NONE',  ( -90.17340840077037001, 87.01269140057999607, 51.39028561444528975 ) ) ;
#11404=VERTEX_POINT ( 'NONE', #1752 ) ;
#11409=CARTESIAN_POINT ( 'NONE',  ( -70.52438641214237691, 96.69972324582255396, 81.21852732034712119 ) ) ;
#11425=CARTESIAN_POINT ( 'NONE',  ( 1.721625266288826284, 55.00000000000000000, 109.9865264768483968 ) ) ;
#11437=CARTESIAN_POINT ( 'NONE',  ( 75.37956130235376406, 75.02634323965499163, -3.232840821497602768 ) ) ;
#11443=CARTESIAN_POINT ( 'NONE',  ( -69.07678759757092735, 92.22190598759939917, 85.60612736256487665 ) ) ;
#11445=CARTESIAN_POINT ( 'NONE',  ( -69.96008568250819337, 88.65447058343966091, 68.72499042888327381 ) ) ;
#11451=VECTOR ( 'NONE', #11359, 1000.000000000000114 ) ;
#11453=CARTESIAN_POINT ( 'NONE',  ( -63.92222308695259869, 94.02752048664899576, 83.80561885825630952 ) ) ;
#11457=DIRECTION ( 'NONE',  ( 0.9999164797902015955, 2.001050586450178695E-22, -0.01292414190464131335 ) ) ;
#11460=ORIENTED_EDGE ( 'NONE', *, *, #3315, .F. ) ;
#11463=CARTESIAN_POINT ( 'NONE',  ( -70.88639693877759385, 71.65513756697318115, -84.11375151051879584 ) ) ;
#11465=( BOUNDED_CURVE ( )  B_SPLINE_CURVE ( 3, ( #14372, #19510, #10799, #769 ),
 .UNSPECIFIED., .F., .T. ) 
 B_SPLINE_CURVE_WITH_KNOTS ( ( 4, 4 ),
 ( 5.799006443144739897, 5.835910511159140057 ),
 .UNSPECIFIED. ) 
 CURVE ( )  GEOMETRIC_REPRESENTATION_ITEM ( )  RATIONAL_B_SPLINE_CURVE ( ( 1.000000000000000000, 0.9998865107004337727, 0.9998865107004337727, 1.000000000000000000 ) ) 
 REPRESENTATION_ITEM ( '' )  );
#11470=CARTESIAN_POINT ( 'NONE',  ( 1.364374644014609697E-14, 69.99999999999998579, -9.836443712999143722E-15 ) ) ;
#11471=ORIENTED_EDGE ( 'NONE', *, *, #5465, .T. ) ;
#11476=AXIS2_PLACEMENT_3D ( 'NONE', #4246, #18603, #13230 ) ;
#11480=DIRECTION ( 'NONE',  ( 0.01292414190464174703, 0.000000000000000000, 0.9999164797902015955 ) ) ;
#11481=ORIENTED_EDGE ( 'NONE', *, *, #20534, .T. ) ;
#11482=EDGE_CURVE ( 'NONE', #784, #19287, #12337, .T. ) ;
#11503=CARTESIAN_POINT ( 'NONE',  ( 106.2089377515399065, 72.00000000000000000, 28.62973177816241588 ) ) ;
#11508=CARTESIAN_POINT ( 'NONE',  ( 36.55288090549195346, 94.02752048664900997, -83.45186405039071076 ) ) ;
#11510=CARTESIAN_POINT ( 'NONE',  ( -72.65825583664232568, 87.55014249100273105, 69.92630806761130202 ) ) ;
#11514=EDGE_CURVE ( 'NONE', #16244, #20892, #17910, .T. ) ;
#11518=VECTOR ( 'NONE', #14993, 1000.000000000000114 ) ;
#11526=CARTESIAN_POINT ( 'NONE',  ( -90.17237370337481650, 87.08103440711009569, 51.34890273202512390 ) ) ;
#11527=EDGE_LOOP ( 'NONE', ( #3110, #7792, #1768, #14768, #2132 ) ) ;
#11535=CARTESIAN_POINT ( 'NONE',  ( -88.17922987063910512, 89.01127821350927150, 51.31456706190138561 ) ) ;
#11536=CARTESIAN_POINT ( 'NONE',  ( -90.66698955146013361, 79.16774870435553169, 29.00429242512959149 ) ) ;
#11542=CARTESIAN_POINT ( 'NONE',  ( 33.82085273160093664, 93.50464841319750064, -82.93470554904388337 ) ) ;
#11549=VECTOR ( 'NONE', #577, 999.9999999999998863 ) ;
#11551=ORIENTED_EDGE ( 'NONE', *, *, #14978, .F. ) ;
#11553=ORIENTED_EDGE ( 'NONE', *, *, #8238, .T. ) ;
#11557=LINE ( 'NONE', #6386, #19824 ) ;
#11567=CARTESIAN_POINT ( 'NONE',  ( 92.46788464407295294, 79.04398536104956463, -28.62013883513311896 ) ) ;
#11569=CARTESIAN_POINT ( 'NONE',  ( 92.79593043952061748, 70.16589065052625074, 59.06731773122648832 ) ) ;
#11573=DIRECTION ( 'NONE',  ( -2.025474946048326158E-22, 1.000000000000000000, -1.876735158486679638E-22 ) ) ;
#11580=DIRECTION ( 'NONE',  ( -0.01292414190464137060, 0.000000000000000000, -0.9999164797902015955 ) ) ;
#11591=CARTESIAN_POINT ( 'NONE',  ( -106.2142196127746558, 77.44923501812726840, -28.61015647369513459 ) ) ;
#11596=ADVANCED_FACE ( 'NONE', ( #7832 ), #9426, .T. ) ;
#11597=CARTESIAN_POINT ( 'NONE',  ( 81.70668847916368804, 104.4142135623730780, -73.64792636435126383 ) ) ;
#11604=EDGE_CURVE ( 'NONE', #16244, #3397, #16327, .T. ) ;
#11612=CARTESIAN_POINT ( 'NONE',  ( 89.66113247980437961, 100.6041916471017856, 63.72504470331089266 ) ) ;
#11618=CARTESIAN_POINT ( 'NONE',  ( -66.71891079484507259, 98.29072687177919931, 79.57820418736568513 ) ) ;
#11620=CARTESIAN_POINT ( 'NONE',  ( -72.65963751957909267, 87.42236182341126494, 69.77244766351077487 ) ) ;
#11621=DIRECTION ( 'NONE',  ( -0.01292414190464130641, 0.000000000000000000, -0.9999164797902015955 ) ) ;
#11627=EDGE_LOOP ( 'NONE', ( #18850, #11209, #5745, #16009 ) ) ;
#11628=DIRECTION ( 'NONE',  ( -0.9999164797902020396, 2.081668151161667201E-14, 0.01292414190462050187 ) ) ;
#11633=CARTESIAN_POINT ( 'NONE',  ( -90.12935778220864336, 87.38120584935140300, 51.16641606481163507 ) ) ;
#11634=CARTESIAN_POINT ( 'NONE',  ( 40.65822637310715493, 91.17157287525387233, 84.25167897319539634 ) ) ;
#11636=EDGE_CURVE ( 'NONE', #14619, #21224, #4447, .T. ) ;
#11641=CARTESIAN_POINT ( 'NONE',  ( 2.067862704742617463, 69.99999999999998579, 159.9866367664322979 ) ) ;
#11644=ORIENTED_EDGE ( 'NONE', *, *, #17041, .F. ) ;
#11648=CARTESIAN_POINT ( 'NONE',  ( 89.99335928417747255, 79.29537036754122425, -29.40900737050180780 ) ) ;
#11651=ORIENTED_EDGE ( 'NONE', *, *, #247, .F. ) ;
#11658=VERTEX_POINT ( 'NONE', #15419 ) ;
#11663=EDGE_CURVE ( 'NONE', #7781, #12967, #11298, .T. ) ;
#11666=CARTESIAN_POINT ( 'NONE',  ( -109.7386064778677621, 75.43227853978193309, -7.937952133666764887 ) ) ;
#11671=DIRECTION ( 'NONE',  ( 0.01292414190464523903, 0.000000000000000000, 0.9999164797902017066 ) ) ;
#11678=ORIENTED_EDGE ( 'NONE', *, *, #12739, .T. ) ;
#11679=ORIENTED_EDGE ( 'NONE', *, *, #12460, .F. ) ;
#11680=EDGE_CURVE ( 'NONE', #12459, #21648, #15202, .T. ) ;
#11688=CARTESIAN_POINT ( 'NONE',  ( 90.02055463237803679, 95.44063823554751025, -63.21629334023821656 ) ) ;
#11697=CARTESIAN_POINT ( 'NONE',  ( -89.66113247980429435, 100.6041916471018709, -63.72504470331098503 ) ) ;
#11699=DIRECTION ( 'NONE',  ( -0.006350819331214699499, 0.8709385446395367936, -0.4913509118287948674 ) ) ;
#11701=PLANE ( 'NONE',  #13071 ) ;
#11703=CARTESIAN_POINT ( 'NONE',  ( -109.3552458118615363, 88.71869973106718987, 50.59427279859775695 ) ) ;
#11705=TOROIDAL_SURFACE ( 'NONE', #12458, 97.00000000000004263, 2.000000000000000000 ) ;
#11707=DIRECTION ( 'NONE',  ( -0.4540042784513456109, 0.000000000000000000, 0.8909995034498464639 ) ) ;
#11713=CARTESIAN_POINT ( 'NONE',  ( 38.89810712971355855, 91.17157287525387233, -85.50986645835283184 ) ) ;
#11724=FACE_OUTER_BOUND ( 'NONE', #19098, .T. ) ;
#11726=CARTESIAN_POINT ( 'NONE',  ( 105.9930786687657616, 70.38870405239202910, 29.41946405304832268 ) ) ;
#11729=STYLED_ITEM ( 'NONE', ( #19198 ), #17376 ) ;
#11737=ADVANCED_FACE ( 'NONE', ( #2667 ), #7936, .F. ) ;
#11738=FACE_OUTER_BOUND ( 'NONE', #17972, .T. ) ;
#11740=CARTESIAN_POINT ( 'NONE',  ( -90.14075885923632825, 87.33211882309382190, 51.19633987193193292 ) ) ;
#11742=VERTEX_POINT ( 'NONE', #6213 ) ;
#11750=ORIENTED_EDGE ( 'NONE', *, *, #2786, .T. ) ;
#11752=CARTESIAN_POINT ( 'NONE',  ( -88.16874431701178594, 88.69758567471752997, 52.43331850404257466 ) ) ;
#11754=CARTESIAN_POINT ( 'NONE',  ( -70.93357090261923759, 91.46354453597339784, -84.07396062241134871 ) ) ;
#11755=EDGE_CURVE ( 'NONE', #9279, #7202, #21411, .T. ) ;
#11757=ORIENTED_EDGE ( 'NONE', *, *, #7786, .F. ) ;
#11758=CARTESIAN_POINT ( 'NONE',  ( -92.40872671617950118, 72.00000000000000000, 33.19707612406966746 ) ) ;
#11759=CARTESIAN_POINT ( 'NONE',  ( -88.28334709335607045, 71.38106462369736960, 62.47119547224009040 ) ) ;
#11760=CARTESIAN_POINT ( 'NONE',  ( 89.41602473586598876, 79.46258270018843461, -29.93333348547120210 ) ) ;
#11763=ORIENTED_EDGE ( 'NONE', *, *, #3162, .F. ) ;
#11768=EDGE_CURVE ( 'NONE', #10450, #17005, #20880, .T. ) ;
#11770=CARTESIAN_POINT ( 'NONE',  ( -64.03197570747913403, 99.62212517233105302, 75.31426563926737572 ) ) ;
#11774=ORIENTED_EDGE ( 'NONE', *, *, #12999, .F. ) ;
#11775=ADVANCED_FACE ( 'NONE', ( #21230 ), #1618, .F. ) ;
#11777=VECTOR ( 'NONE', #11457, 1000.000000000000114 ) ;
#11781=DIRECTION ( 'NONE',  ( 0.01292414190464131508, 0.000000000000000000, 0.9999164797902017066 ) ) ;
#11784=CARTESIAN_POINT ( 'NONE',  ( -88.16157026904451754, 88.04290212818517602, 53.06700061362226961 ) ) ;
#11787=CARTESIAN_POINT ( 'NONE',  ( -92.89382307712746467, 70.12557134413805215, -58.91325363510486568 ) ) ;
#11794=CARTESIAN_POINT ( 'NONE',  ( 90.65403358069686135, 80.14440291447091624, -32.01641220276457034 ) ) ;
#11797=DIRECTION ( 'NONE',  ( 0.9999164797902015955, 2.001050586450176109E-22, -0.01292414190464270113 ) ) ;
#11799=EDGE_CURVE ( 'NONE', #18358, #17537, #15707, .T. ) ;
#11803=ORIENTED_EDGE ( 'NONE', *, *, #9562, .T. ) ;
#11805=EDGE_LOOP ( 'NONE', ( #2615, #9844, #18063, #3189 ) ) ;
#11806=AXIS2_PLACEMENT_3D ( 'NONE', #10237, #4937, #13699 ) ;
#11810=CARTESIAN_POINT ( 'NONE',  ( -68.68766895589030241, 71.65104882840749667, 85.91861595181278233 ) ) ;
#11813=DIRECTION ( 'NONE',  ( 0.006350819331212799977, -0.8709385446395345731, 0.4913509118287983091 ) ) ;
#11815=FACE_OUTER_BOUND ( 'NONE', #16954, .T. ) ;
#11820=VECTOR ( 'NONE', #7907, 1000.000000000000000 ) ;
#11823=CARTESIAN_POINT ( 'NONE',  ( 106.8724933792760226, 79.04398536104964990, 26.04362031086705542 ) ) ;
#11837=CARTESIAN_POINT ( 'NONE',  ( 1.717753310876226625, 55.00000000000000000, 109.6869605904137330 ) ) ;
#11843=CARTESIAN_POINT ( 'NONE',  ( -84.78539177974977292, 105.0000000000000000, -70.08164767436865361 ) ) ;
#11847=CARTESIAN_POINT ( 'NONE',  ( 1.121675378414679125, 105.0000000000000000, 109.9942809619911799 ) ) ;
#11851=CARTESIAN_POINT ( 'NONE',  ( 85.63433794141033673, 105.0000000000000000, 69.04172771111926465 ) ) ;
#11862=ORIENTED_EDGE ( 'NONE', *, *, #6023, .F. ) ;
#11863=CARTESIAN_POINT ( 'NONE',  ( -90.13703512730879197, 87.34900181192021762, 51.18604840036999093 ) ) ;
#11866=CARTESIAN_POINT ( 'NONE',  ( -73.50537112628094860, 95.94772729216980167, 81.83508847720149504 ) ) ;
#11867=CARTESIAN_POINT ( 'NONE',  ( -90.40889375659909888, 72.00000000000000000, 33.17122784026039284 ) ) ;
#11869=ORIENTED_EDGE ( 'NONE', *, *, #396, .T. ) ;
#11870=SURFACE_SIDE_STYLE ('',( #19080 ) ) ;
#11872=CARTESIAN_POINT ( 'NONE',  ( -88.17224338757175417, 88.87565977966644937, 52.08196082309276420 ) ) ;
#11874=CARTESIAN_POINT ( 'NONE',  ( -71.61338682171090397, 92.58578643762702143, -83.49564556265197268 ) ) ;
#11876=VERTEX_POINT ( 'NONE', #14498 ) ;
#11877=DIRECTION ( 'NONE',  ( 0.01292414190464131335, 0.000000000000000000, 0.9999164797902017066 ) ) ;
#11888=LINE ( 'NONE', #18874, #9600 ) ;
#11892=ORIENTED_EDGE ( 'NONE', *, *, #16352, .T. ) ;
#11893=CARTESIAN_POINT ( 'NONE',  ( -90.04195528733428944, 70.03010874511689110, 63.23285121931508712 ) ) ;
#11899=EDGE_CURVE ( 'NONE', #12967, #10097, #16101, .T. ) ;
#11903=CARTESIAN_POINT ( 'NONE',  ( -92.21925947168412563, 70.54513337289785113, -59.96440893983639597 ) ) ;
#11911=CARTESIAN_POINT ( 'NONE',  ( 88.42079784105918350, 80.23159800265106867, -32.23730667790416504 ) ) ;
#11913=CARTESIAN_POINT ( 'NONE',  ( -69.43142427201328815, 92.58578643762699301, 85.31868097644080251 ) ) ;
#11922=CARTESIAN_POINT ( 'NONE',  ( -109.1029698478473051, 104.3814432989690602, 70.11238825523858509 ) ) ;
#11931=PLANE ( 'NONE',  #15897 ) ;
#11933=ORIENTED_EDGE ( 'NONE', *, *, #4857, .T. ) ;
#11961=ORIENTED_EDGE ( 'NONE', *, *, #11663, .F. ) ;
#11962=DIRECTION ( 'NONE',  ( -0.9999164797902015955, -2.001050586450177050E-22, 0.01292414190464223796 ) ) ;
#11974=CIRCLE ( 'NONE', #2055, 1.989999999999997105 ) ;
#11976=CARTESIAN_POINT ( 'NONE',  ( -88.16578817886077957, 88.47953432603556223, 52.70984377781922348 ) ) ;
#11984=CARTESIAN_POINT ( 'NONE',  ( -70.91392079944854743, 91.17157287525390075, -84.09052168258642723 ) ) ;
#11994=CARTESIAN_POINT ( 'NONE',  ( 89.90836385050337753, 100.2819950034553926, 63.37719018575645435 ) ) ;
#11997=ORIENTED_EDGE ( 'NONE', *, *, #16815, .T. ) ;
#11998=ORIENTED_EDGE ( 'NONE', *, *, #15005, .T. ) ;
#11999=ORIENTED_EDGE ( 'NONE', *, *, #21407, .T. ) ;
#12000=CARTESIAN_POINT ( 'NONE',  ( 92.43457499998882554, 77.12912189496645965, -31.19724316448930423 ) ) ;
#12018=CARTESIAN_POINT ( 'NONE',  ( -89.22767861003021039, 80.31838830481380853, -30.18953644180660945 ) ) ;
#12021=EDGE_CURVE ( 'NONE', #9861, #9560, #6422, .T. ) ;
#12024=CARTESIAN_POINT ( 'NONE',  ( -90.40889375659909888, 69.99999999999998579, 33.17122784026039284 ) ) ;
#12029=CIRCLE ( 'NONE', #21186, 2.000000000000004441 ) ;
#12030=EDGE_CURVE ( 'NONE', #11876, #7316, #10095, .T. ) ;
#12034=CARTESIAN_POINT ( 'NONE',  ( 108.6051929143323065, 76.36431273661730756, -17.61389195241292782 ) ) ;
#12039=B_SPLINE_CURVE_WITH_KNOTS ( 'NONE', 3,
 ( #17616, #12559, #14286, #19431, #8733, #10715, #19208, #3692, #10837, #8632, #28, #13934, #16133, #17860, #3479, #10492 ),
 .UNSPECIFIED., .F., .F.,
 ( 4, 2, 2, 2, 2, 2, 2, 4 ),
 ( 0.000000000000000000, 0.0004728798714926100619, 0.0009457597429852201238, 0.001418639614477830132, 0.001891519485970440248, 0.002364399357463050581, 0.002837279228955660263, 0.003783038971940870521 ),
 .UNSPECIFIED. ) ;
#12052=AXIS2_PLACEMENT_3D ( 'NONE', #12944, #6140, #983 ) ;
#12053=VERTEX_POINT ( 'NONE', #21890 ) ;
#12057=CARTESIAN_POINT ( 'NONE',  ( -68.71681667565952978, 69.99999999999998579, 85.89527988174785378 ) ) ;
#12061=ORIENTED_EDGE ( 'NONE', *, *, #2259, .F. ) ;
#12065=VERTEX_POINT ( 'NONE', #6186 ) ;
#12069=DIRECTION ( 'NONE',  ( 0.000000000000000000, 0.000000000000000000, 1.000000000000000000 ) ) ;
#12071=CARTESIAN_POINT ( 'NONE',  ( 106.2089377515398780, 77.28919246392754872, 28.62973177816271431 ) ) ;
#12072=DIRECTION ( 'NONE',  ( 2.025474946048326158E-22, -1.000000000000000000, 1.876735158486679638E-22 ) ) ;
#12076=VERTEX_POINT ( 'NONE', #18484 ) ;
#12079=ORIENTED_EDGE ( 'NONE', *, *, #16606, .F. ) ;
#12080=CARTESIAN_POINT ( 'NONE',  ( 90.37009694938035409, 70.86971351442876710, -62.71573865539092907 ) ) ;
#12081=CARTESIAN_POINT ( 'NONE',  ( -90.05797812368525967, 88.60843922159206443, 52.63312143047516400 ) ) ;
#12088=CARTESIAN_POINT ( 'NONE',  ( -4.843581286828654520, 86.22336876296598973, -75.02848097551373030 ) ) ;
#12092=DIRECTION ( 'NONE',  ( 0.9999164797902015955, 2.001050586450177050E-22, -0.01292414190464223796 ) ) ;
#12096=ORIENTED_EDGE ( 'NONE', *, *, #3895, .F. ) ;
#12113=CYLINDRICAL_SURFACE ( 'NONE', #6037, 1.999999999999997780 ) ;
#12114=AXIS2_PLACEMENT_3D ( 'NONE', #9030, #11344, #325 ) ;
#12115=ORIENTED_EDGE ( 'NONE', *, *, #11768, .T. ) ;
#12120=EDGE_CURVE ( 'NONE', #18358, #367, #4911, .T. ) ;
#12130=AXIS2_PLACEMENT_3D ( 'NONE', #6250, #16496, #16833 ) ;
#12134=ORIENTED_EDGE ( 'NONE', *, *, #7185, .F. ) ;
#12135=AXIS2_PLACEMENT_3D ( 'NONE', #3134, #18758, #9922 ) ;
#12137=CIRCLE ( 'NONE', #6269, 6.499999999999998224 ) ;
#12138=FACE_OUTER_BOUND ( 'NONE', #12383, .T. ) ;
#12167=CARTESIAN_POINT ( 'NONE',  ( -39.36913080622078809, 69.99999999999998579, 87.51612159803859470 ) ) ;
#12174=ORIENTED_EDGE ( 'NONE', *, *, #13562, .F. ) ;
#12175=CARTESIAN_POINT ( 'NONE',  ( -35.70966223998150468, 93.64690829566262664, 83.82160924485184239 ) ) ;
#12178=LINE ( 'NONE', #16090, #10301 ) ;
#12180=VECTOR ( 'NONE', #8964, 1000.000000000000000 ) ;
#12183=CARTESIAN_POINT ( 'NONE',  ( -83.58290648752343088, 104.4142135623730780, -71.51152175067954886 ) ) ;
#12185=ORIENTED_EDGE ( 'NONE', *, *, #1383, .T. ) ;
#12190=CARTESIAN_POINT ( 'NONE',  ( 106.2880716433167976, 78.18499655656310665, 28.33463432393087089 ) ) ;
#12203=CARTESIAN_POINT ( 'NONE',  ( 64.07473967894682687, 103.0000000000000000, -72.00569783435743432 ) ) ;
#12204=CARTESIAN_POINT ( 'NONE',  ( -89.90032551572470254, 87.88518503742774612, 50.85709393580534510 ) ) ;
#12210=CARTESIAN_POINT ( 'NONE',  ( -74.36685259725942387, 95.85792126150981574, 81.05301575120802227 ) ) ;
#12215=CARTESIAN_POINT ( 'NONE',  ( 84.94669401314519064, 75.00864948959271317, 0.2251543083152826030 ) ) ;
#12216=CIRCLE ( 'NONE', #8173, 1.999999999999997335 ) ;
#12220=VERTEX_POINT ( 'NONE', #3417 ) ;
#12222=CARTESIAN_POINT ( 'NONE',  ( -79.39043653009960622, 75.13519862315604314, -4.041203518313574605 ) ) ;
#12227=CARTESIAN_POINT ( 'NONE',  ( -65.90110554552374822, 105.0000000000000000, -69.29678410920486442 ) ) ;
#12231=EDGE_LOOP ( 'NONE', ( #14640, #3777, #18792 ) ) ;
#12233=B_SPLINE_CURVE_WITH_KNOTS ( 'NONE', 3,
 ( #21697, #2660, #5859, #13020 ),
 .UNSPECIFIED., .F., .F.,
 ( 4, 4 ),
 ( 0.1567379737884350144, 0.1627913398252618660 ),
 .UNSPECIFIED. ) ;
#12238=CARTESIAN_POINT ( 'NONE',  ( 91.86813470756436573, 77.17527876199572745, -31.26628371047692667 ) ) ;
#12240=DIRECTION ( 'NONE',  ( -0.01292414190464131335, -1.902755938799530239E-22, -0.9999164797902015955 ) ) ;
#12243=CARTESIAN_POINT ( 'NONE',  ( -64.99457118636308905, 169.9999999999999716, 0.8400692238016759239 ) ) ;
#12253=CIRCLE ( 'NONE', #19218, 110.0000000000000142 ) ;
#12254=CARTESIAN_POINT ( 'NONE',  ( -93.21002351426727728, 77.12912189496638860, -28.79774562292281814 ) ) ;
#12259=AXIS2_PLACEMENT_3D ( 'NONE', #21623, #15126, #4066 ) ;
#12260=CARTESIAN_POINT ( 'NONE',  ( -64.99457118636308905, 105.0000000000000000, 0.8400692238016757019 ) ) ;
#12263=ORIENTED_EDGE ( 'NONE', *, *, #17039, .T. ) ;
#12267=VERTEX_POINT ( 'NONE', #1807 ) ;
#12273=PRODUCT_DEFINITION ( 'UNKNOWN', '', #770, #5572 ) ;
#12274=DIRECTION ( 'NONE',  ( 0.01292414190464131508, 3.469447142229204684E-15, 0.9999164797902017066 ) ) ;
#12282=CARTESIAN_POINT ( 'NONE',  ( -90.64608739977010998, 77.80075968338644543, 32.24365086765050847 ) ) ;
#12283=CARTESIAN_POINT ( 'NONE',  ( -64.99457118636308905, 177.0000000000003695, 0.8400692238016794766 ) ) ;
#12291=CARTESIAN_POINT ( 'NONE',  ( -70.91392079944854743, 69.99999999999998579, -84.09052168258642723 ) ) ;
#12299=DIRECTION ( 'NONE',  ( -2.025474946048326158E-22, 1.000000000000000000, -1.876735158486679638E-22 ) ) ;
#12306=ADVANCED_FACE ( 'NONE', ( #14469 ), #6499, .T. ) ;
#12314=CARTESIAN_POINT ( 'NONE',  ( 37.54386652542171277, 92.77591188308413450, 82.72434418715882032 ) ) ;
#12317=LINE ( 'NONE', #1731, #1676 ) ;
#12321=ORIENTED_EDGE ( 'NONE', *, *, #3315, .T. ) ;
#12324=CARTESIAN_POINT ( 'NONE',  ( -89.99979403183252202, 87.72028009250037428, 50.95876237836445455 ) ) ;
#12325=ADVANCED_FACE ( 'NONE', ( #18569 ), #7887, .T. ) ;
#12330=( LENGTH_UNIT ( ) NAMED_UNIT ( * ) SI_UNIT ( .MILLI., .METRE. ) );
#12337=LINE ( 'NONE', #17613, #1623 ) ;
#12338=CARTESIAN_POINT ( 'NONE',  ( -75.38806545726168906, 75.02669947309938436, 3.231589135580875904 ) ) ;
#12345=CYLINDRICAL_SURFACE ( 'NONE', #5509, 2.000000000000004885 ) ;
#12362=CARTESIAN_POINT ( 'NONE',  ( -89.85940970469351896, 88.83791317007154476, 86.46162627816347879 ) ) ;
#12365=CARTESIAN_POINT ( 'NONE',  ( 92.80269534486838268, 79.83421200779717708, 28.82571798309749056 ) ) ;
#12367=CYLINDRICAL_SURFACE ( 'NONE', #1496, 2.000000000000004441 ) ;
#12368=EDGE_CURVE ( 'NONE', #4404, #21811, #13321, .T. ) ;
#12372=ORIENTED_EDGE ( 'NONE', *, *, #58, .F. ) ;
#12373=CARTESIAN_POINT ( 'NONE',  ( -91.37189824458694432, 79.16991425845397146, -26.65847270750067111 ) ) ;
#12380=PLANE ( 'NONE',  #20287 ) ;
#12383=EDGE_LOOP ( 'NONE', ( #15031, #21661, #21437, #18362 ) ) ;
#12387=EDGE_CURVE ( 'NONE', #9306, #10904, #8534, .T. ) ;
#12410=CARTESIAN_POINT ( 'NONE',  ( 90.02055463237803679, 72.00000000000000000, -63.21629334023821656 ) ) ;
#12411=ORIENTED_EDGE ( 'NONE', *, *, #12030, .F. ) ;
#12412=FACE_OUTER_BOUND ( 'NONE', #11020, .T. ) ;
#12420=ORIENTED_EDGE ( 'NONE', *, *, #13529, .F. ) ;
#12424=CARTESIAN_POINT ( 'NONE',  ( -90.06162176126106544, 87.58759337840020009, 51.04022814688357812 ) ) ;
#12426=AXIS2_PLACEMENT_3D ( 'NONE', #15686, #390, #2108 ) ;
#12431=CARTESIAN_POINT ( 'NONE',  ( 84.36058151735579713, 75.03814149158517921, 1.605125682363267803 ) ) ;
#12439=CARTESIAN_POINT ( 'NONE',  ( -76.83013909114643525, 75.08639547911839429, 5.048240262065343487 ) ) ;
#12441=TOROIDAL_SURFACE ( 'NONE', #1057, 97.00000000000004263, 2.000000000000000000 ) ;
#12442=ADVANCED_FACE ( 'NONE', ( #15027 ), #9837, .T. ) ;
#12443=ORIENTED_EDGE ( 'NONE', *, *, #7661, .F. ) ;
#12450=ORIENTED_EDGE ( 'NONE', *, *, #17355, .T. ) ;
#12455=EDGE_CURVE ( 'NONE', #10325, #7269, #7742, .T. ) ;
#12458=AXIS2_PLACEMENT_3D ( 'NONE', #9680, #8177, #20222 ) ;
#12459=VERTEX_POINT ( 'NONE', #1757 ) ;
#12460=EDGE_CURVE ( 'NONE', #17368, #11196, #11204, .T. ) ;
#12468=CARTESIAN_POINT ( 'NONE',  ( 91.22751156961064112, 80.31838830481379432, 30.16368815799726733 ) ) ;
#12469=EDGE_CURVE ( 'NONE', #1373, #12267, #9110, .T. ) ;
#12471=B_SPLINE_CURVE_WITH_KNOTS ( 'NONE', 3,
 ( #4274, #4504, #6239, #6122, #4050, #13265, #7616, #14655, #18303, #4384, #11299, #9225, #16612, #12929 ),
 .UNSPECIFIED., .F., .F.,
 ( 4, 2, 2, 2, 2, 2, 4 ),
 ( 0.000000000000000000, 0.0005169893790259184321, 0.001033978758051836864, 0.001550968137077755188, 0.002067957516103673728, 0.003101936274155510376, 0.004135915032207347457 ),
 .UNSPECIFIED. ) ;
#12475=CARTESIAN_POINT ( 'NONE',  ( 92.43457499998882554, 69.99999999999998579, -31.19724316448930779 ) ) ;
#12479=CARTESIAN_POINT ( 'NONE',  ( -89.98285967923901296, 79.53265832318567163, -27.83436926225114050 ) ) ;
#12480=ORIENTED_EDGE ( 'NONE', *, *, #20997, .F. ) ;
#12490=EDGE_LOOP ( 'NONE', ( #1736, #10607, #6418, #19202 ) ) ;
#12491=DIRECTION ( 'NONE',  ( 0.01292414190464131335, 0.000000000000000000, 0.9999164797902017066 ) ) ;
#12492=DIRECTION ( 'NONE',  ( -0.7968670734554590407, -0.4220031449644014443, 0.4323380770678043605 ) ) ;
#12496=VERTEX_POINT ( 'NONE', #8981 ) ;
#12518=ORIENTED_EDGE ( 'NONE', *, *, #4969, .F. ) ;
#12523=DIRECTION ( 'NONE',  ( 1.490566292661454305E-14, 1.000000000000000000, -1.926591840573834312E-16 ) ) ;
#12526=AXIS2_PLACEMENT_3D ( 'NONE', #15644, #20671, #1294 ) ;
#12529=DIRECTION ( 'NONE',  ( -0.01292414190464049456, -1.752983723092351571E-15, -0.9999164797902015955 ) ) ;
#12536=CARTESIAN_POINT ( 'NONE',  ( -89.72047535737752355, 89.01802868918773015, 51.97649104033645528 ) ) ;
#12537=EDGE_CURVE ( 'NONE', #2301, #17537, #10839, .T. ) ;
#12542=ORIENTED_EDGE ( 'NONE', *, *, #3461, .T. ) ;
#12543=ORIENTED_EDGE ( 'NONE', *, *, #1920, .T. ) ;
#12546=DIRECTION ( 'NONE',  ( 0.4654428868037193689, 0.8850574712643738406, -0.006015952371159188211 ) ) ;
#12550=DIRECTION ( 'NONE',  ( 2.025474946048326158E-22, -1.000000000000000000, 1.876735158486679638E-22 ) ) ;
#12554=CARTESIAN_POINT ( 'NONE',  ( -110.3526887502520992, 77.12912189496645965, -26.57600582461530081 ) ) ;
#12558=ORIENTED_EDGE ( 'NONE', *, *, #17126, .T. ) ;
#12559=CARTESIAN_POINT ( 'NONE',  ( -105.4334892372614121, 77.28905753105595977, 31.36525700924959636 ) ) ;
#12564=VERTEX_POINT ( 'NONE', #22316 ) ;
#12568=ORIENTED_EDGE ( 'NONE', *, *, #12796, .F. ) ;
#12580=DIRECTION ( 'NONE',  ( 0.009138748381789079875, 0.7071067811865487940, 0.7070477234798316912 ) ) ;
#12597=CARTESIAN_POINT ( 'NONE',  ( -92.62880990220969579, 79.84869560962759749, -28.85690742247488672 ) ) ;
#12598=VERTEX_POINT ( 'NONE', #21590 ) ;
#12599=EDGE_CURVE ( 'NONE', #21368, #9437, #12216, .T. ) ;
#12600=ADVANCED_FACE ( 'NONE', ( #14636 ), #10373, .F. ) ;
#12605=CIRCLE ( 'NONE', #1252, 2.000000000000000888 ) ;
#12607=DIRECTION ( 'NONE',  ( 2.025474946048326158E-22, -1.000000000000000000, 1.876735158486678933E-22 ) ) ;
#12612=ORIENTED_EDGE ( 'NONE', *, *, #5705, .F. ) ;
#12615=CARTESIAN_POINT ( 'NONE',  ( 67.26198047107926925, 70.17996908938924605, -87.03937574298602442 ) ) ;
#12617=CARTESIAN_POINT ( 'NONE',  ( -89.97519728687143470, 79.29963411167480558, 29.42247391813824109 ) ) ;
#12631=ORIENTED_EDGE ( 'NONE', *, *, #21192, .T. ) ;
#12632=LINE ( 'NONE', #21328, #15426 ) ;
#12633=ORIENTED_EDGE ( 'NONE', *, *, #11514, .F. ) ;
#12634=CARTESIAN_POINT ( 'NONE',  ( 71.61338682171094661, 92.58578643762700722, 83.49564556265194426 ) ) ;
#12639=DIRECTION ( 'NONE',  ( 0.9999164797902017066, -6.938893703802208150E-15, -0.01292414190464825571 ) ) ;
#12653=ORIENTED_EDGE ( 'NONE', *, *, #5726, .T. ) ;
#12662=CARTESIAN_POINT ( 'NONE',  ( -89.92919990131169072, 88.83226839477106296, 52.34107143949843532 ) ) ;
#12665=ORIENTED_EDGE ( 'NONE', *, *, #22384, .T. ) ;
#12673=FACE_OUTER_BOUND ( 'NONE', #4034, .T. ) ;
#12679=CARTESIAN_POINT ( 'NONE',  ( -78.90025544361535026, 75.13007332810630601, -3.950326719918461293 ) ) ;
#12686=CYLINDRICAL_SURFACE ( 'NONE', #8442, 110.0000000000000000 ) ;
#12691=ORIENTED_EDGE ( 'NONE', *, *, #10829, .F. ) ;
#12692=CARTESIAN_POINT ( 'NONE',  ( -80.26018450689494443, 75.13699351169597662, 6.137806644758510011 ) ) ;
#12693=DIRECTION ( 'NONE',  ( 2.025474946048326158E-22, -1.000000000000000000, 1.876735158486679638E-22 ) ) ;
#12695=DIRECTION ( 'NONE',  ( 0.01292414190464174703, 0.000000000000000000, 0.9999164797902015955 ) ) ;
#12704=CARTESIAN_POINT ( 'NONE',  ( 89.24560213809748177, 80.14548850073731501, 29.69112557292140053 ) ) ;
#12709=DIRECTION ( 'NONE',  ( 0.9999164797902017066, 0.000000000000000000, -0.01292414190463832269 ) ) ;
#12711=CARTESIAN_POINT ( 'NONE',  ( -91.32446103601363063, 78.00118640252709667, -30.19495016275356747 ) ) ;
#12720=DIRECTION ( 'NONE',  ( 0.9999164797902017066, 2.001050586450178931E-22, -0.01292414190464131508 ) ) ;
#12728=CARTESIAN_POINT ( 'NONE',  ( -91.14374963600238289, 79.10773180776112667, 28.81380175419842615 ) ) ;
#12729=EDGE_LOOP ( 'NONE', ( #8040, #19254, #1729, #7477 ) ) ;
#12731=DIRECTION ( 'NONE',  ( 2.025474946048326158E-22, -1.000000000000000000, 1.876735158486679638E-22 ) ) ;
#12739=EDGE_CURVE ( 'NONE', #13713, #21368, #16645, .T. ) ;
#12741=ORIENTED_EDGE ( 'NONE', *, *, #10784, .F. ) ;
#12749=ORIENTED_EDGE ( 'NONE', *, *, #6764, .F. ) ;
#12755=CARTESIAN_POINT ( 'NONE',  ( -20.14358671158747072, 88.61365832079873428, 77.93650841479222890 ) ) ;
#12759=CARTESIAN_POINT ( 'NONE',  ( 40.65822637310716203, 69.99999999999998579, 84.25167897319536792 ) ) ;
#12762=CARTESIAN_POINT ( 'NONE',  ( -88.18706637290516426, 88.71869973106716145, 50.32066939225187241 ) ) ;
#12765=CARTESIAN_POINT ( 'NONE',  ( -90.83733885584940992, 70.37256007341385100, 62.03708646394351689 ) ) ;
#12766=ADVANCED_FACE ( 'NONE', ( #22373 ), #17242, .F. ) ;
#12770=ORIENTED_EDGE ( 'NONE', *, *, #5912, .T. ) ;
#12771=CARTESIAN_POINT ( 'NONE',  ( -106.1801133998812929, 71.34284122058934940, -28.73649967668641381 ) ) ;
#12773=VERTEX_POINT ( 'NONE', #17034 ) ;
#12775=ORIENTED_EDGE ( 'NONE', *, *, #9347, .F. ) ;
#12790=CARTESIAN_POINT ( 'NONE',  ( -105.1274178938603825, 70.25451017443430146, 32.37651503794364771 ) ) ;
#12792=CARTESIAN_POINT ( 'NONE',  ( -88.16274635857531905, 88.18390162297423274, 52.97334896370593782 ) ) ;
#12796=EDGE_CURVE ( 'NONE', #5654, #12220, #3339, .T. ) ;
#12805=CYLINDRICAL_SURFACE ( 'NONE', #20656, 2.000000000000004885 ) ;
#12810=( BOUNDED_SURFACE ( )  B_SPLINE_SURFACE ( 3, 2, ( 
 ( #4711, #10029, #860 ),
 ( #11409, #16607, #7853 ),
 ( #20110, #18533, #14986 ),
 ( #2895, #4381, #18419 ) ),
 .UNSPECIFIED., .F., .F., .T. ) 
 B_SPLINE_SURFACE_WITH_KNOTS ( ( 4, 4 ),
 ( 3, 3 ),
 ( 0.07609981584028600865, 0.08941542774493665968 ),
 ( 0.000000000000000000, 1.000000000000000000 ),
 .UNSPECIFIED. ) 
 GEOMETRIC_REPRESENTATION_ITEM ( )  RATIONAL_B_SPLINE_SURFACE ( (
 ( 1.000000000000000000, 0.6989529655644959316, 1.000000000000000000),
 ( 1.000000000000000000, 0.6987865376935388229, 1.000000000000000000),
 ( 1.000000000000000000, 0.6986099777012620970, 1.000000000000000000),
 ( 1.000000000000000000, 0.6984211671062240390, 1.000000000000000000) ) ) 
 REPRESENTATION_ITEM ( '' )  SURFACE ( )  );
#12811=CARTESIAN_POINT ( 'NONE',  ( 394.6585245357460963, 69.99999999999997158, -112.1099862245463896 ) ) ;
#12823=CARTESIAN_POINT ( 'NONE',  ( -64.99457118636308905, 169.9999999999999716, 0.8400692238016759239 ) ) ;
#12830=AXIS2_PLACEMENT_3D ( 'NONE', #21369, #12550, #3912 ) ;
#12831=PLANE ( 'NONE',  #10063 ) ;
#12835=CARTESIAN_POINT ( 'NONE',  ( -90.42410873942375815, 78.25489917908669213, 32.91867509261335556 ) ) ;
#12836=CARTESIAN_POINT ( 'NONE',  ( -39.39497909003006981, 69.99999999999998579, 85.51628863845817818 ) ) ;
#12840=B_SPLINE_CURVE_WITH_KNOTS ( 'NONE', 3,
 ( #7571, #22613, #19837, #19721, #21344, #14603, #5830 ),
 .UNSPECIFIED., .F., .F.,
 ( 4, 3, 4 ),
 ( 0.000000000000000000, 0.005203688037432161254, 0.009927031861615774611 ),
 .UNSPECIFIED. ) ;
#12845=DIRECTION ( 'NONE',  ( 0.9999164797902015955, 2.001050586450178695E-22, -0.01292414190464131335 ) ) ;
#12855=ORIENTED_EDGE ( 'NONE', *, *, #5568, .F. ) ;
#12863=CARTESIAN_POINT ( 'NONE',  ( 1.117803423002110774, 45.00000000000000000, 109.6947150755565161 ) ) ;
#12872=AXIS2_PLACEMENT_3D ( 'NONE', #14550, #21185, #17775 ) ;
#12875=CARTESIAN_POINT ( 'NONE',  ( -89.78587645599536415, 88.03336485954913826, 50.76527035810606492 ) ) ;
#12882=VECTOR ( 'NONE', #3265, 1000.000000000000000 ) ;
#12893=DIRECTION ( 'NONE',  ( -2.025474946048326158E-22, 1.000000000000000000, -1.876735158486679638E-22 ) ) ;
#12894=ORIENTED_EDGE ( 'NONE', *, *, #19853, .T. ) ;
#12896=AXIS2_PLACEMENT_3D ( 'NONE', #21318, #19697, #21532 ) ;
#12903=FACE_OUTER_BOUND ( 'NONE', #2071, .T. ) ;
#12907=EDGE_CURVE ( 'NONE', #16500, #13344, #21018, .T. ) ;
#12909=ORIENTED_EDGE ( 'NONE', *, *, #21017, .T. ) ;
#12911=CARTESIAN_POINT ( 'NONE',  ( 397.1141114976279596, 91.17157287525404286, 77.87414493559184336 ) ) ;
#12913=CIRCLE ( 'NONE', #15116, 2.000000000000001776 ) ;
#12918=CARTESIAN_POINT ( 'NONE',  ( -81.38707033994185736, 75.12824275668154428, -3.883447788322965444 ) ) ;
#12919=CARTESIAN_POINT ( 'NONE',  ( -88.16289161317095591, 88.20043279625843979, 52.96119657702186601 ) ) ;
#12921=VERTEX_POINT ( 'NONE', #15164 ) ;
#12926=CIRCLE ( 'NONE', #7409, 2.000000000000001332 ) ;
#12928=AXIS2_PLACEMENT_3D ( 'NONE', #22558, #13657, #8573 ) ;
#12929=CARTESIAN_POINT ( 'NONE',  ( 68.43148148480361215, 69.99999999999998579, 86.12277481476651531 ) ) ;
#12934=CARTESIAN_POINT ( 'NONE',  ( 20.17774460750976928, 88.61083286335994558, -77.93556127472962203 ) ) ;
#12940=EDGE_CURVE ( 'NONE', #15089, #7368, #4133, .T. ) ;
#12943=ORIENTED_EDGE ( 'NONE', *, *, #6764, .T. ) ;
#12944=CARTESIAN_POINT ( 'NONE',  ( 93.23587179807657321, 72.00000000000000000, 30.79757858250317781 ) ) ;
#12951=AXIS2_PLACEMENT_3D ( 'NONE', #1165, #15190, #6542 ) ;
#12953=CARTESIAN_POINT ( 'NONE',  ( 75.13896584913651111, 75.01394013563931651, -2.606578332019783506 ) ) ;
#12954=CARTESIAN_POINT ( 'NONE',  ( -90.01145195396890131, 71.38761518557662100, 62.48983541110989393 ) ) ;
#12958=CARTESIAN_POINT ( 'NONE',  ( -68.71681667565952978, 91.32006346413032816, 85.89527988174788220 ) ) ;
#12965=CARTESIAN_POINT ( 'NONE',  ( -91.18811779502803461, 77.39015272472282447, 31.60719401330432277 ) ) ;
#12967=VERTEX_POINT ( 'NONE', #10187 ) ;
#12969=EDGE_CURVE ( 'NONE', #3481, #7202, #16868, .T. ) ;
#12970=LINE ( 'NONE', #2612, #5136 ) ;
#12977=CARTESIAN_POINT ( 'NONE',  ( -93.23587179807654479, 72.00000000000000000, -30.79757858250321689 ) ) ;
#12979=AXIS2_PLACEMENT_3D ( 'NONE', #13246, #1510, #6555 ) ;
#12989=ORIENTED_EDGE ( 'NONE', *, *, #11680, .T. ) ;
#12999=EDGE_CURVE ( 'NONE', #10113, #4456, #18681, .T. ) ;
#13003=AXIS2_PLACEMENT_3D ( 'NONE', #3098, #1041, #1499 ) ;
#13006=CARTESIAN_POINT ( 'NONE',  ( -89.82557373136849321, 87.98571510324423173, 50.79485365709339106 ) ) ;
#13010=EDGE_LOOP ( 'NONE', ( #14791, #14982, #3101, #16031 ) ) ;
#13019=CARTESIAN_POINT ( 'NONE',  ( -106.1519489938925602, 71.09828217887417168, -28.84036442345827922 ) ) ;
#13020=CARTESIAN_POINT ( 'NONE',  ( 86.79222083800954124, 104.3814432989690602, 67.58039954014910222 ) ) ;
#13023=CARTESIAN_POINT ( 'NONE',  ( 34.61804907780420848, 94.93197183469659706, -82.52232902628021805 ) ) ;
#13025=CARTESIAN_POINT ( 'NONE',  ( -68.71681667565952978, 69.99999999999998579, 85.89527988174785378 ) ) ;
#13037=ORIENTED_EDGE ( 'NONE', *, *, #3904, .T. ) ;
#13044=CARTESIAN_POINT ( 'NONE',  ( -90.14332777612271741, 88.20948563679688448, 52.98067045136929920 ) ) ;
#13050=DIRECTION ( 'NONE',  ( -0.009138748381789112835, -0.7071067811865462405, -0.7070477234798343558 ) ) ;
#13056=CARTESIAN_POINT ( 'NONE',  ( 28.61719497298777526, 91.18493411151780492, -80.66446637815775489 ) ) ;
#13059=CARTESIAN_POINT ( 'NONE',  ( 91.45377919752198181, 96.73472523269998646, 61.12462174243592727 ) ) ;
#13062=CARTESIAN_POINT ( 'NONE',  ( 63.92222308695262711, 94.02752048664900997, -83.80561885825635215 ) ) ;
#13071=AXIS2_PLACEMENT_3D ( 'NONE', #16559, #6429, #8145 ) ;
#13081=CARTESIAN_POINT ( 'NONE',  ( 92.02635692360502162, 79.83422912033846330, -31.21470397902952598 ) ) ;
#13095=ADVANCED_FACE ( 'NONE', ( #6951 ), #8905, .F. ) ;
#13099=CARTESIAN_POINT ( 'NONE',  ( 82.50899511402293740, 104.9527666485724922, -72.74866258673912967 ) ) ;
#13102=FACE_OUTER_BOUND ( 'NONE', #16512, .T. ) ;
#13109=CARTESIAN_POINT ( 'NONE',  ( -88.17103187914774765, 88.81848268355626885, 52.20485361863669027 ) ) ;
#13113=EDGE_CURVE ( 'NONE', #14836, #13307, #8904, .T. ) ;
#13114=CARTESIAN_POINT ( 'NONE',  ( 90.41042953090175160, 78.34730160488619788, -33.05240787946388537 ) ) ;
#13120=CARTESIAN_POINT ( 'NONE',  ( 69.33518156588188219, 92.50622784628018280, -85.39700225480594042 ) ) ;
#13122=CARTESIAN_POINT ( 'NONE',  ( -65.35548625431930247, 98.86074611927202227, 78.99051476369086799 ) ) ;
#13125=DIRECTION ( 'NONE',  ( 0.9999164797902017066, 2.001050586450178931E-22, -0.01292414190464131508 ) ) ;
#13137=CARTESIAN_POINT ( 'NONE',  ( -84.79288518521889273, 75.01682528584525755, -0.6987393684433246266 ) ) ;
#13138=CARTESIAN_POINT ( 'NONE',  ( -88.16204873317377633, 88.10266582584259254, 53.02941603701640361 ) ) ;
#13139=ORIENTED_EDGE ( 'NONE', *, *, #21603, .F. ) ;
#13145=PLANE ( 'NONE',  #1789 ) ;
#13168=ORIENTED_EDGE ( 'NONE', *, *, #7950, .T. ) ;
#13185=CARTESIAN_POINT ( 'NONE',  ( 91.18811779502807724, 77.39015272472096285, -31.60719401330434764 ) ) ;
#13188=ORIENTED_EDGE ( 'NONE', *, *, #16705, .T. ) ;
#13194=ORIENTED_EDGE ( 'NONE', *, *, #13735, .F. ) ;
#13197=CARTESIAN_POINT ( 'NONE',  ( -67.26198047107922662, 70.17996908938924605, 87.03937574298602442 ) ) ;
#13198=CLOSED_SHELL ( 'NONE', ( #14461, #8574, #6053, #16940, #19437, #3993, #6002, #5252, #2755, #16718, #15688, #15205, #4192, #13861, #19914, #8866, #289, #10184, #16949, #6428, #5970, #8810, #3375, #22571, #20413, #19059, #13356, #15300, #9267, #4322, #5743, #22045, #12766, #11775, #2075, #1515, #18222, #19342, #16003, #9814, #7600, #12325, #10916, #21270, #17554, #14446, #13995, #2450, #13095, #22651, #7235, #13549, #6397, #6681, #22528, #16250, #2816, #8229, #22418, #5597, #5390, #18357, #8962, #22119, #14007, #3606, #9498, #7135, #17211, #12600, #6035, #9173, #9087, #4695, #8771, #16871, #11097, #8524, #6821, #8030, #4708, #647, #5988, #1156, #5333, #10505, #4060, #1444, #4312, #21012, #11596, #11737, #7399, #15144, #17833, #14063, #13905, #12306, #14797, #17503, #18101, #2639, #14529, #17747, #3976, #8613, #20340, #18344, #319, #6114, #13409, #15606, #15062, #21960, #20843, #2738, #18511, #12442, #11307, #14656, #21517, #19308, #17713, #9639 ) ) ;
#13199=AXIS2_PLACEMENT_3D ( 'NONE', #3625, #14109, #12491 ) ;
#13203=DIRECTION ( 'NONE',  ( -2.025474946048326158E-22, 1.000000000000000000, -1.876735158486679638E-22 ) ) ;
#13205=ORIENTED_EDGE ( 'NONE', *, *, #16128, .T. ) ;
#13208=ORIENTED_EDGE ( 'NONE', *, *, #510, .T. ) ;
#13210=CARTESIAN_POINT ( 'NONE',  ( -106.4939345422101979, 78.92840590577348792, -27.55192737125463509 ) ) ;
#13212=CARTESIAN_POINT ( 'NONE',  ( -109.0842784177615101, 103.0000000000000000, 71.55850894251706507 ) ) ;
#13214=CARTESIAN_POINT ( 'NONE',  ( 90.02055463237803679, 34.61572286322119396, -63.21629334023821656 ) ) ;
#13219=ORIENTED_EDGE ( 'NONE', *, *, #8083, .F. ) ;
#13222=CARTESIAN_POINT ( 'NONE',  ( -89.48935565494650746, 89.10721938022165034, 51.64438126496267500 ) ) ;
#13224=ORIENTED_EDGE ( 'NONE', *, *, #20185, .F. ) ;
#13230=DIRECTION ( 'NONE',  ( 0.01292414190464133070, 0.000000000000000000, 0.9999164797902015955 ) ) ;
#13233=CARTESIAN_POINT ( 'NONE',  ( 106.8724933792760226, 79.04398536104964990, 26.04362031086705542 ) ) ;
#13240=DIRECTION ( 'NONE',  ( -2.025474946048326158E-22, 1.000000000000000000, -1.876735158486679638E-22 ) ) ;
#13246=CARTESIAN_POINT ( 'NONE',  ( 64.99457118636311748, 169.9999999999999716, -0.8400692238016952418 ) ) ;
#13253=AXIS2_PLACEMENT_3D ( 'NONE', #18188, #2440, #9430 ) ;
#13255=CARTESIAN_POINT ( 'NONE',  ( -88.16211553172512083, 88.11043810238577123, 53.02430440011134039 ) ) ;
#13256=CARTESIAN_POINT ( 'NONE',  ( -88.82263333796718996, 169.9999999999999716, 1.148052203164670715 ) ) ;
#13263=CARTESIAN_POINT ( 'NONE',  ( 41.59208321381912299, 69.99999999999998579, 84.46951292587608862 ) ) ;
#13265=CARTESIAN_POINT ( 'NONE',  ( 70.53865358177317546, 70.91952051830753589, 84.40563445996843939 ) ) ;
#13266=ORIENTED_EDGE ( 'NONE', *, *, #14165, .F. ) ;
#13267=DIRECTION ( 'NONE',  ( 0.9999164797902015955, 2.001050586450178695E-22, -0.01292414190464131335 ) ) ;
#13270=CARTESIAN_POINT ( 'NONE',  ( 31.27336289421850424, 92.26071163157524779, -81.74815335747254608 ) ) ;
#13272=DIRECTION ( 'NONE',  ( -0.01292414190464131335, -1.902755938799530239E-22, -0.9999164797902015955 ) ) ;
#13275=CYLINDRICAL_SURFACE ( 'NONE', #42, 2.000000000000004441 ) ;
#13277=CARTESIAN_POINT ( 'NONE',  ( -105.4334892372614121, 34.61572286322119396, 31.36525700924958926 ) ) ;
#13279=LINE ( 'NONE', #9595, #18292 ) ;
#13289=CARTESIAN_POINT ( 'NONE',  ( 93.23587179807657321, 72.00000000000000000, 30.79757858250317781 ) ) ;
#13291=CARTESIAN_POINT ( 'NONE',  ( -109.9781218937930447, 75.08416348859604739, -3.222660468417803514 ) ) ;
#13297=EDGE_CURVE ( 'NONE', #12076, #16780, #19206, .T. ) ;
#13302=CARTESIAN_POINT ( 'NONE',  ( 89.84434271629412194, 96.73102593143109118, -63.46658414958751848 ) ) ;
#13305=CARTESIAN_POINT ( 'NONE',  ( 88.94497886703048550, 79.67058643966726095, -30.57398350459212821 ) ) ;
#13307=VERTEX_POINT ( 'NONE', #11784 ) ;
#13311=ORIENTED_EDGE ( 'NONE', *, *, #2493, .T. ) ;
#13314=ORIENTED_EDGE ( 'NONE', *, *, #106, .F. ) ;
#13316=VERTEX_POINT ( 'NONE', #9939 ) ;
#13317=EDGE_CURVE ( 'NONE', #3464, #6883, #10470, .T. ) ;
#13321=CIRCLE ( 'NONE', #14427, 6.499999999999998224 ) ;
#13333=FACE_OUTER_BOUND ( 'NONE', #8819, .T. ) ;
#13335=CARTESIAN_POINT ( 'NONE',  ( -88.16117291386304089, 87.99029836822313655, 53.09774323446453081 ) ) ;
#13336=VECTOR ( 'NONE', #6516, 1000.000000000000000 ) ;
#13344=VERTEX_POINT ( 'NONE', #19565 ) ;
#13348=PLANE ( 'NONE',  #4822 ) ;
#13356=ADVANCED_FACE ( 'NONE', ( #176, #15929 ), #3601, .T. ) ;
#13361=CARTESIAN_POINT ( 'NONE',  ( 105.6848962833589809, 69.99999999999998579, 30.50771805806152770 ) ) ;
#13366=ORIENTED_EDGE ( 'NONE', *, *, #21534, .T. ) ;
#13374=CARTESIAN_POINT ( 'NONE',  ( -89.99511487588330283, 88.72984820209772749, 52.48309319825106201 ) ) ;
#13377=VERTEX_POINT ( 'NONE', #2009 ) ;
#13386=EDGE_CURVE ( 'NONE', #9075, #5608, #7052, .T. ) ;
#13391=CARTESIAN_POINT ( 'NONE',  ( -90.02465904577691447, 70.02851260093143537, 63.21045060945284888 ) ) ;
#13408=CARTESIAN_POINT ( 'NONE',  ( 105.8709953322713488, 79.07548657612767329, -29.85559726770835098 ) ) ;
#13409=ADVANCED_FACE ( 'NONE', ( #13843 ), #6822, .T. ) ;
#13410=CARTESIAN_POINT ( 'NONE',  ( -93.18852247616528928, 70.03011042807717956, -58.44685241948167231 ) ) ;
#13419=CARTESIAN_POINT ( 'NONE',  ( 93.38631075262973980, 69.99999999999998579, 58.13036983636535382 ) ) ;
#13421=CARTESIAN_POINT ( 'NONE',  ( 84.07537730384214569, 105.0000000000000000, 70.09082476868245237 ) ) ;
#13426=CARTESIAN_POINT ( 'NONE',  ( -68.58360120290727480, 71.33040186743640731, 86.00170974875814522 ) ) ;
#13438=AXIS2_PLACEMENT_3D ( 'NONE', #16899, #1390, #14857 ) ;
#13439=CYLINDRICAL_SURFACE ( 'NONE', #9971, 2.000000000000004885 ) ;
#13447=ORIENTED_EDGE ( 'NONE', *, *, #16308, .F. ) ;
#13449=CARTESIAN_POINT ( 'NONE',  ( -90.03465221005033925, 70.01281497139055432, 63.19621350536183968 ) ) ;
#13450=EDGE_CURVE ( 'NONE', #495, #21379, #7095, .T. ) ;
#13459=CARTESIAN_POINT ( 'NONE',  ( 88.82263333796723259, 169.9999999999999716, -1.148052203164690033 ) ) ;
#13462=CARTESIAN_POINT ( 'NONE',  ( -72.51438462527775641, 87.23323244114081376, 69.92599951943640235 ) ) ;
#13466=DIRECTION ( 'NONE',  ( 0.01292414190464044946, 1.902755938799528828E-22, 0.9999164797902017066 ) ) ;
#13467=DIRECTION ( 'NONE',  ( 0.01292414190464131335, 0.000000000000000000, 0.9999164797902017066 ) ) ;
#13474=DIRECTION ( 'NONE',  ( 0.01292414190464125957, 0.000000000000000000, 0.9999164797902015955 ) ) ;
#13477=CARTESIAN_POINT ( 'NONE',  ( -90.07216641000893276, 88.57119983275795505, 52.67302757455067308 ) ) ;
#13480=CARTESIAN_POINT ( 'NONE',  ( -75.30975508861040169, 94.90914755154933857, 80.17755788556743823 ) ) ;
#13487=CARTESIAN_POINT ( 'NONE',  ( -71.26616241777601601, 92.22173151023517335, -83.79227730723270895 ) ) ;
#13492=CARTESIAN_POINT ( 'NONE',  ( -109.6363981638670566, 79.04398536104955042, 28.84204567386034057 ) ) ;
#13498=VERTEX_POINT ( 'NONE', #18207 ) ;
#13517=CIRCLE ( 'NONE', #19000, 85.00000000000002842 ) ;
#13518=CARTESIAN_POINT ( 'NONE',  ( 88.55041925573031847, 79.97987315375630146, -31.50236046386200428 ) ) ;
#13529=EDGE_CURVE ( 'NONE', #4193, #18705, #20712, .T. ) ;
#13532=CARTESIAN_POINT ( 'NONE',  ( -66.18268079339598842, 69.99999999999998579, 87.86269266872857031 ) ) ;
#13537=CIRCLE ( 'NONE', #10591, 2.000000000000004885 ) ;
#13538=CYLINDRICAL_SURFACE ( 'NONE', #17623, 112.5000000000000284 ) ;
#13539=CARTESIAN_POINT ( 'NONE',  ( 109.5443584724616670, 75.69229587323870589, 10.26624083857056569 ) ) ;
#13549=ADVANCED_FACE ( 'NONE', ( #16155 ), #17511, .T. ) ;
#13551=CARTESIAN_POINT ( 'NONE',  ( 41.09521125350256909, 91.17157287525387233, 84.47593510598149180 ) ) ;
#13559=ORIENTED_EDGE ( 'NONE', *, *, #9376, .F. ) ;
#13561=CYLINDRICAL_SURFACE ( 'NONE', #13003, 1.999999999999997780 ) ;
#13562=EDGE_CURVE ( 'NONE', #369, #367, #9057, .T. ) ;
#13564=CARTESIAN_POINT ( 'NONE',  ( -88.44870386694205422, 88.71936310223436806, 50.32514765335821494 ) ) ;
#13577=DIRECTION ( 'NONE',  ( -0.9999164797902015955, -2.001050586450178695E-22, 0.01292414190464131335 ) ) ;
#13581=CARTESIAN_POINT ( 'NONE',  ( -64.15090010559214306, 90.56097911118510524, 66.11330928953715613 ) ) ;
#13582=CARTESIAN_POINT ( 'NONE',  ( -90.12303247369654002, 87.40561052298997424, 51.15152651009733376 ) ) ;
#13583=EDGE_CURVE ( 'NONE', #899, #19083, #20358, .T. ) ;
#13588=CARTESIAN_POINT ( 'NONE',  ( -33.82085273160089400, 93.50464841319747222, 82.93470554904384073 ) ) ;
#13589=FACE_OUTER_BOUND ( 'NONE', #19978, .T. ) ;
#13593=CARTESIAN_POINT ( 'NONE',  ( -90.43417961988758691, 79.20545292891345923, 29.12427242046052456 ) ) ;
#13598=DIRECTION ( 'NONE',  ( 0.9999164797902017066, 0.000000000000000000, -0.01292414190464174703 ) ) ;
#13600=DIRECTION ( 'NONE',  ( 5.257943380984030796E-16, -1.000000000000000000, -6.795817950787834712E-18 ) ) ;
#13605=ORIENTED_EDGE ( 'NONE', *, *, #3728, .T. ) ;
#13610=CIRCLE ( 'NONE', #18371, 95.00000000000004263 ) ;
#13617=EDGE_CURVE ( 'NONE', #11404, #21601, #3579, .T. ) ;
#13621=CARTESIAN_POINT ( 'NONE',  ( -85.63433794141032251, 105.0000000000000000, -69.04172771111927887 ) ) ;
#13627=ORIENTED_EDGE ( 'NONE', *, *, #2259, .T. ) ;
#13630=CARTESIAN_POINT ( 'NONE',  ( -41.59208321381909457, 72.00000000000000000, -84.46951292587610283 ) ) ;
#13631=CARTESIAN_POINT ( 'NONE',  ( -1.124400345703740589, 69.99999999999998579, -86.99273374174759965 ) ) ;
#13632=DIRECTION ( 'NONE',  ( -2.025474946048326158E-22, 1.000000000000000000, -1.876735158486679638E-22 ) ) ;
#13634=ORIENTED_EDGE ( 'NONE', *, *, #19061, .F. ) ;
#13636=CARTESIAN_POINT ( 'NONE',  ( -71.83229293602242649, 94.61330589943089819, 83.32202392072876762 ) ) ;
#13640=CARTESIAN_POINT ( 'NONE',  ( 39.39497909003009823, 69.99999999999998579, -85.51628863845822082 ) ) ;
#13641=ORIENTED_EDGE ( 'NONE', *, *, #18112, .T. ) ;
#13644=CIRCLE ( 'NONE', #2629, 1.999999999999998002 ) ;
#13657=DIRECTION ( 'NONE',  ( 2.025474946048326158E-22, -1.000000000000000000, 1.876735158486679638E-22 ) ) ;
#13665=CIRCLE ( 'NONE', #16622, 1.999999999999999112 ) ;
#13685=EDGE_CURVE ( 'NONE', #10904, #9306, #4550, .T. ) ;
#13689=( BOUNDED_SURFACE ( )  B_SPLINE_SURFACE ( 3, 2, ( 
 ( #14319, #12468, #400 ),
 ( #3501, #2014, #9111 ),
 ( #17528, #8758, #12704 ),
 ( #10859, #9003, #9232 ),
 ( #17884, #19671, #19571 ),
 ( #10962, #3605, #16279 ),
 ( #3941, #19456, #7396 ),
 ( #8889, #16160, #17988 ),
 ( #7519, #5435, #10516 ),
 ( #14547, #15935, #19346 ),
 ( #1781, #7059, #284 ),
 ( #14090, #182, #21073 ),
 ( #7177, #21286, #14207 ),
 ( #5326, #12365, #21181 ),
 ( #3722, #10742, #16049 ),
 ( #19903, #18106, #7620 ),
 ( #18546, #14662, #16493 ),
 ( #20119, #9456, #15111 ) ),
 .UNSPECIFIED., .F., .F., .T. ) 
 B_SPLINE_SURFACE_WITH_KNOTS ( ( 4, 2, 2, 2, 2, 2, 2, 2, 4 ),
 ( 3, 3 ),
 ( 0.003005090483489993892, 0.003807341501471060968, 0.004609592519452128043, 0.005411843537433195551, 0.006214094555414263060, 0.007016345573395330569, 0.007818596591376398078, 0.008620847609357464719, 0.009423098627338533095 ),
 ( 0.000000000000000000, 1.000000000000000000 ),
 .UNSPECIFIED. ) 
 GEOMETRIC_REPRESENTATION_ITEM ( )  RATIONAL_B_SPLINE_SURFACE ( (
 ( 1.000000000000000000, 0.7071067811865479058, 1.000000000000000000),
 ( 1.000000000000000000, 0.6996407321458223416, 1.000000000000000000),
 ( 1.000000000000000000, 0.6923367522679467756, 1.000000000000000000),
 ( 1.000000000000000000, 0.6780525511370015801, 1.000000000000000000),
 ( 1.000000000000000000, 0.6710180578253038819, 1.000000000000000000),
 ( 1.000000000000000000, 0.6575437683264738764, 1.000000000000000000),
 ( 1.000000000000000000, 0.6511910073848069525, 1.000000000000000000),
 ( 1.000000000000000000, 0.6392329869082525873, 1.000000000000000000),
 ( 1.000000000000000000, 0.6335699185534187095, 1.000000000000000000),
 ( 1.000000000000000000, 0.6233860397583550483, 1.000000000000000000),
 ( 1.000000000000000000, 0.6188536248677808382, 1.000000000000000000),
 ( 1.000000000000000000, 0.6108845495338327547, 1.000000000000000000),
 ( 1.000000000000000000, 0.6074396204518591746, 1.000000000000000000),
 ( 1.000000000000000000, 0.6019717515917274442, 1.000000000000000000),
 ( 1.000000000000000000, 0.5998961748957651885, 1.000000000000000000),
 ( 1.000000000000000000, 0.5970819659647461641, 1.000000000000000000),
 ( 1.000000000000000000, 0.5963755918898637765, 1.000000000000000000),
 ( 1.000000000000000000, 0.5963808372950819559, 1.000000000000000000) ) ) 
 REPRESENTATION_ITEM ( '' )  SURFACE ( )  );
#13699=DIRECTION ( 'NONE',  ( -0.01292414190464044946, -1.902755938799528593E-22, -0.9999164797902015955 ) ) ;
#13701=CARTESIAN_POINT ( 'NONE',  ( -65.88241411543796744, 104.3814432989690602, -67.85066342192638444 ) ) ;
#13703=CARTESIAN_POINT ( 'NONE',  ( -90.15184476568182959, 87.27496089121102329, 51.23113957728794077 ) ) ;
#13705=VERTEX_POINT ( 'NONE', #8685 ) ;
#13711=CARTESIAN_POINT ( 'NONE',  ( -89.24601225622836864, 80.14389198580502693, -29.68648583522428908 ) ) ;
#13713=VERTEX_POINT ( 'NONE', #12167 ) ;
#13716=DIRECTION ( 'NONE',  ( 0.9999164797902017066, 2.001050586450178931E-22, -0.01292414190464131508 ) ) ;
#13718=CIRCLE ( 'NONE', #3795, 2.000000000000004885 ) ;
#13735=EDGE_CURVE ( 'NONE', #6286, #14017, #3427, .T. ) ;
#13737=DIRECTION ( 'NONE',  ( -2.025474946048326158E-22, 1.000000000000000000, -1.876735158486679638E-22 ) ) ;
#13739=VECTOR ( 'NONE', #10474, 1000.000000000000114 ) ;
#13741=CARTESIAN_POINT ( 'NONE',  ( -93.58499681124557412, 69.99999999999998579, -57.80872228166919058 ) ) ;
#13747=EDGE_CURVE ( 'NONE', #3481, #11404, #521, .T. ) ;
#13749=ORIENTED_EDGE ( 'NONE', *, *, #12469, .F. ) ;
#13751=FACE_BOUND ( 'NONE', #8558, .T. ) ;
#13759=AXIS2_PLACEMENT_3D ( 'NONE', #3586, #15676, #22619 ) ;
#13761=DIRECTION ( 'NONE',  ( 0.9999164797902017066, 2.001050586450178931E-22, -0.01292414190464131508 ) ) ;
#13764=VERTEX_POINT ( 'NONE', #13975 ) ;
#13770=ORIENTED_EDGE ( 'NONE', *, *, #18976, .T. ) ;
#13775=CARTESIAN_POINT ( 'NONE',  ( 1.117803423002105445, 55.00000000000000000, 109.6947150755565161 ) ) ;
#13778=DIRECTION ( 'NONE',  ( -0.01220060921879500236, -0.3298969072164960603, -0.9439381207174974975 ) ) ;
#13780=DIRECTION ( 'NONE',  ( -0.01292414190463830014, 0.000000000000000000, -0.9999164797902017066 ) ) ;
#13784=CARTESIAN_POINT ( 'NONE',  ( -36.93353118839863924, 92.00280690333769940, 84.44237658584599160 ) ) ;
#13787=CARTESIAN_POINT ( 'NONE',  ( -93.21002351426726307, 69.99999999999998579, -28.79774562292281104 ) ) ;
#13790=ORIENTED_EDGE ( 'NONE', *, *, #8058, .F. ) ;
#13808=CARTESIAN_POINT ( 'NONE',  ( 92.05960170301050027, 69.99999999999998579, -60.20821982323567312 ) ) ;
#13809=CARTESIAN_POINT ( 'NONE',  ( -90.09760470754743267, 87.49028989906726395, 51.09979543946362668 ) ) ;
#13810=B_SPLINE_CURVE_WITH_KNOTS ( 'NONE', 3,
 ( #2541, #6094, #16461, #7931, #4134, #19746, #10930, #708, #13120, #4355 ),
 .UNSPECIFIED., .F., .F.,
 ( 4, 2, 2, 2, 4 ),
 ( 0.000000000000000000, 0.0004370559136044528279, 0.0008741118272089056559, 0.001311167740813358375, 0.001748223654417811312 ),
 .UNSPECIFIED. ) ;
#13816=( BOUNDED_SURFACE ( )  B_SPLINE_SURFACE ( 3, 2, ( 
 ( #8934, #218, #7215 ),
 ( #19156, #19500, #14243 ),
 ( #21218, #5476, #17462 ),
 ( #11634, #2561, #2889 ) ),
 .UNSPECIFIED., .F., .F., .T. ) 
 B_SPLINE_SURFACE_WITH_KNOTS ( ( 4, 4 ),
 ( 3, 3 ),
 ( 0.4226013619543070310, 0.4841788640348457240 ),
 ( 0.000000000000000000, 1.000000000000000000 ),
 .UNSPECIFIED. ) 
 GEOMETRIC_REPRESENTATION_ITEM ( )  RATIONAL_B_SPLINE_SURFACE ( (
 ( 1.000000000000000000, 0.9068900557993654354, 1.000000000000000000),
 ( 1.000000000000000000, 0.9052491015987689238, 1.000000000000000000),
 ( 1.000000000000000000, 0.9034913259101540195, 1.000000000000000000),
 ( 1.000000000000000000, 0.9016180287879275168, 1.000000000000000000) ) ) 
 REPRESENTATION_ITEM ( '' )  SURFACE ( )  );
#13817=CARTESIAN_POINT ( 'NONE',  ( -92.43457499998879712, 72.00000000000000000, 31.19724316448926160 ) ) ;
#13829=ORIENTED_EDGE ( 'NONE', *, *, #22130, .T. ) ;
#13834=CARTESIAN_POINT ( 'NONE',  ( -64.01537291612297054, 100.1864212328113979, 76.59879228792688366 ) ) ;
#13835=ORIENTED_EDGE ( 'NONE', *, *, #12969, .F. ) ;
#13843=FACE_OUTER_BOUND ( 'NONE', #14395, .T. ) ;
#13844=CARTESIAN_POINT ( 'NONE',  ( -91.81287659828484493, 71.13119029400843374, -60.58394261007859427 ) ) ;
#13848=DIRECTION ( 'NONE',  ( -2.025474946048326158E-22, 1.000000000000000000, -1.876735158486678933E-22 ) ) ;
#13849=EDGE_CURVE ( 'NONE', #5713, #12267, #8911, .T. ) ;
#13850=CYLINDRICAL_SURFACE ( 'NONE', #9565, 85.00000000000001421 ) ;
#13853=EDGE_CURVE ( 'NONE', #6959, #9437, #17414, .T. ) ;
#13861=ADVANCED_FACE ( 'NONE', ( #19928 ), #12831, .T. ) ;
#13865=DIRECTION ( 'NONE',  ( 0.009985269297341583389, 0.6348858185549669519, 0.7725414498878678815 ) ) ;
#13872=CARTESIAN_POINT ( 'NONE',  ( 107.9412751340845489, 77.72595396897827413, 21.65777188997737213 ) ) ;
#13880=CARTESIAN_POINT ( 'NONE',  ( -79.90518398323658289, 100.1635695855007668, -75.81005614957796013 ) ) ;
#13901=CARTESIAN_POINT ( 'NONE',  ( -89.66113247980429435, 100.6041916471018709, -63.72504470331098503 ) ) ;
#13902=DIRECTION ( 'NONE',  ( -0.9999164797902017066, -2.001050586450180576E-22, 0.01292414190464044946 ) ) ;
#13905=ADVANCED_FACE ( 'NONE', ( #11135 ), #20175, .F. ) ;
#13915=CARTESIAN_POINT ( 'NONE',  ( -88.16898101804537191, 88.70782710634040313, 52.40912332135838625 ) ) ;
#13916=CARTESIAN_POINT ( 'NONE',  ( -66.37745437015971106, 69.99999999999997158, -106.1509941137499595 ) ) ;
#13919=ORIENTED_EDGE ( 'NONE', *, *, #8333, .T. ) ;
#13920=DIRECTION ( 'NONE',  ( 0.4119494117036593406, -0.9111911607883945718, -0.005324537360869059308 ) ) ;
#13922=CARTESIAN_POINT ( 'NONE',  ( -16.24193888600903435, 87.34754884532240737, -76.12214651130867082 ) ) ;
#13923=LINE ( 'NONE', #15330, #16519 ) ;
#13924=CARTESIAN_POINT ( 'NONE',  ( 83.04991721846113251, 75.08645580250137641, -5.130063099084944511 ) ) ;
#13926=LINE ( 'NONE', #10374, #2349 ) ;
#13928=ORIENTED_EDGE ( 'NONE', *, *, #15184, .F. ) ;
#13932=CARTESIAN_POINT ( 'NONE',  ( -79.59455004317675275, 75.13699351169599083, 6.129203171928941707 ) ) ;
#13934=CARTESIAN_POINT ( 'NONE',  ( -105.8287943736951604, 79.03195428549125268, 30.00479353936295368 ) ) ;
#13935=ORIENTED_EDGE ( 'NONE', *, *, #15574, .F. ) ;
#13936=EDGE_CURVE ( 'NONE', #5713, #9934, #6894, .T. ) ;
#13937=CARTESIAN_POINT ( 'NONE',  ( 93.62421092229767794, 69.99999999999998579, 60.84264408248096601 ) ) ;
#13943=ORIENTED_EDGE ( 'NONE', *, *, #20534, .F. ) ;
#13946=VERTEX_POINT ( 'NONE', #19189 ) ;
#13953=CARTESIAN_POINT ( 'NONE',  ( -90.15896375023012865, 69.98053812266098817, 63.28569483684161412 ) ) ;
#13959=CARTESIAN_POINT ( 'NONE',  ( 89.71476837554287442, 79.66528429935014799, 28.24846625074276929 ) ) ;
#13963=VECTOR ( 'NONE', #19396, 1000.000000000000114 ) ;
#13967=VERTEX_POINT ( 'NONE', #15657 ) ;
#13968=CARTESIAN_POINT ( 'NONE',  ( -91.13609774473528091, 79.20914543161394761, -26.78943607724156095 ) ) ;
#13973=EDGE_CURVE ( 'NONE', #7249, #15798, #5051, .T. ) ;
#13975=CARTESIAN_POINT ( 'NONE',  ( 80.05923150692980528, 54.99999999999999289, 4.065642694558706971 ) ) ;
#13976=DIRECTION ( 'NONE',  ( -0.006690748560446689759, 0.8555659502960908380, -0.5176505950712777526 ) ) ;
#13987=ORIENTED_EDGE ( 'NONE', *, *, #6118, .F. ) ;
#13995=ADVANCED_FACE ( 'NONE', ( #10788 ), #14132, .F. ) ;
#13998=CARTESIAN_POINT ( 'NONE',  ( -90.85853474116407824, 77.59429383720566875, 31.92673238494555221 ) ) ;
#14003=VECTOR ( 'NONE', #12731, 1000.000000000000000 ) ;
#14007=ADVANCED_FACE ( 'NONE', ( #10444 ), #13816, .T. ) ;
#14010=CIRCLE ( 'NONE', #5182, 95.00000000000004263 ) ;
#14011=CIRCLE ( 'NONE', #50, 2.000000000000004885 ) ;
#14017=VERTEX_POINT ( 'NONE', #18629 ) ;
#14027=CARTESIAN_POINT ( 'NONE',  ( -88.72067713466817906, 101.8298110126636260, -65.04826529396217438 ) ) ;
#14028=DIRECTION ( 'NONE',  ( -0.01292414190529159179, 1.415534356397187034E-10, -0.9999164797901932689 ) ) ;
#14039=CIRCLE ( 'NONE', #12928, 6.499999999999998224 ) ;
#14043=CARTESIAN_POINT ( 'NONE',  ( -89.85464669586853859, 88.91429508965254058, 52.20121630638777077 ) ) ;
#14053=CARTESIAN_POINT ( 'NONE',  ( 82.15928189060839770, 75.11374352463818127, 3.586303559386837314 ) ) ;
#14054=AXIS2_PLACEMENT_3D ( 'NONE', #954, #14525, #7601 ) ;
#14060=CARTESIAN_POINT ( 'NONE',  ( -74.88934953599625999, 74.99999364505980282, 1.298876317593433916 ) ) ;
#14062=DIRECTION ( 'NONE',  ( 0.01292414190464131682, 0.000000000000000000, 0.9999164797902017066 ) ) ;
#14063=ADVANCED_FACE ( 'NONE', ( #8188 ), #15580, .T. ) ;
#14067=CARTESIAN_POINT ( 'NONE',  ( 104.8611102782643343, 70.00000000000000000, -33.22898942131121913 ) ) ;
#14073=EDGE_LOOP ( 'NONE', ( #20774, #2600, #14475, #1388 ) ) ;
#14090=CARTESIAN_POINT ( 'NONE',  ( 92.18978923775409839, 77.29775901949989247, 29.08785173819693881 ) ) ;
#14092=CARTESIAN_POINT ( 'NONE',  ( 89.33746586332900108, 79.97654757638647993, 29.19326486971733914 ) ) ;
#14093=CARTESIAN_POINT ( 'NONE',  ( 91.62437796271727564, 95.71196945526500599, 60.86849236629024062 ) ) ;
#14094=DIRECTION ( 'NONE',  ( -0.01292414190464130641, 8.584198644008937464E-16, -0.9999164797902015955 ) ) ;
#14098=CARTESIAN_POINT ( 'NONE',  ( -92.30767208729371021, 77.25770192717985196, -29.02102379856271952 ) ) ;
#14100=AXIS2_PLACEMENT_3D ( 'NONE', #17675, #15962, #7197 ) ;
#14102=CARTESIAN_POINT ( 'NONE',  ( -70.44022362938049753, 70.80424004364375890, -84.48783506240401664 ) ) ;
#14109=DIRECTION ( 'NONE',  ( -2.025474946048326158E-22, 1.000000000000000000, -1.876735158486679638E-22 ) ) ;
#14116=CARTESIAN_POINT ( 'NONE',  ( -88.82263333796721838, 169.9999999999999716, 1.148052203164671159 ) ) ;
#14132=PLANE ( 'NONE',  #7499 ) ;
#14134=CIRCLE ( 'NONE', #21081, 2.000000000000001332 ) ;
#14138=CARTESIAN_POINT ( 'NONE',  ( 38.92395541352284738, 91.17157287525387233, -83.51003349877244375 ) ) ;
#14142=DIRECTION ( 'NONE',  ( -0.006350819331213198964, 0.8709385446395360164, -0.4913509118287961996 ) ) ;
#14151=CARTESIAN_POINT ( 'NONE',  ( -93.62421092229762110, 72.00000000000000000, -60.84264408248100864 ) ) ;
#14160=CARTESIAN_POINT ( 'NONE',  ( -89.95235262792742503, 87.80448589959429739, 50.90690957908749681 ) ) ;
#14161=VECTOR ( 'NONE', #12092, 1000.000000000000114 ) ;
#14165=EDGE_CURVE ( 'NONE', #20879, #44, #464, .T. ) ;
#14167=LINE ( 'NONE', #7241, #70 ) ;
#14171=LINE ( 'NONE', #17607, #14161 ) ;
#14175=CARTESIAN_POINT ( 'NONE',  ( 71.61338682171094661, 92.58578643762700722, 83.49564556265194426 ) ) ;
#14177=CARTESIAN_POINT ( 'NONE',  ( -77.49583701682549020, 75.10299918630330751, -3.425180504331486908 ) ) ;
#14200=CARTESIAN_POINT ( 'NONE',  ( -91.00106904273528130, 70.29040131071506892, 61.79648398638329354 ) ) ;
#14201=CARTESIAN_POINT ( 'NONE',  ( 106.1636641531657972, 79.04398536104962147, -28.79715981783310497 ) ) ;
#14207=CARTESIAN_POINT ( 'NONE',  ( 91.37189824458509690, 79.16991425845409935, 26.65847270750105480 ) ) ;
#14214=EDGE_LOOP ( 'NONE', ( #15772, #1476, #6942 ) ) ;
#14215=DIRECTION ( 'NONE',  ( 0.01292414190464131335, 0.000000000000000000, 0.9999164797902017066 ) ) ;
#14217=LINE ( 'NONE', #3270, #1129 ) ;
#14220=DIRECTION ( 'NONE',  ( 0.01292414190464131335, 1.902755938799530239E-22, 0.9999164797902015955 ) ) ;
#14231=CARTESIAN_POINT ( 'NONE',  ( -90.47544334247993447, 78.08471258854567054, 32.66922098773510186 ) ) ;
#14243=CARTESIAN_POINT ( 'NONE',  ( 38.37734285175992710, 94.19957547781432083, 82.31130495470515029 ) ) ;
#14255=DIRECTION ( 'NONE',  ( 0.01292414190464131508, 1.902755938799530474E-22, 0.9999164797902017066 ) ) ;
#14256=DIRECTION ( 'NONE',  ( -0.9999164797902017066, -2.001050586450180576E-22, 0.01292414190464044946 ) ) ;
#14264=EDGE_LOOP ( 'NONE', ( #19441, #11651, #17445 ) ) ;
#14266=CARTESIAN_POINT ( 'NONE',  ( -88.16771777505866226, 88.62629760424535164, 52.53058358910858061 ) ) ;
#14267=ORIENTED_EDGE ( 'NONE', *, *, #10040, .T. ) ;
#14272=PLANE ( 'NONE',  #22053 ) ;
#14274=DIRECTION ( 'NONE',  ( -0.9999164797902015955, -2.001050586450178695E-22, 0.01292414190464131335 ) ) ;
#14279=ORIENTED_EDGE ( 'NONE', *, *, #7356, .F. ) ;
#14280=CARTESIAN_POINT ( 'NONE',  ( 394.9504264446939032, 92.58578643762714933, -89.52608615654102664 ) ) ;
#14286=CARTESIAN_POINT ( 'NONE',  ( -105.4390993001728276, 77.44561610140179653, 31.34641640711149790 ) ) ;
#14291=CARTESIAN_POINT ( 'NONE',  ( 104.9795361740884090, 70.06102247219406820, -32.85291587203231245 ) ) ;
#14297=ORIENTED_EDGE ( 'NONE', *, *, #10409, .T. ) ;
#14300=EDGE_CURVE ( 'NONE', #10951, #6286, #1818, .T. ) ;
#14308=VECTOR ( 'NONE', #20411, 1000.000000000000000 ) ;
#14311=EDGE_CURVE ( 'NONE', #1581, #3464, #21742, .T. ) ;
#14316=CARTESIAN_POINT ( 'NONE',  ( -90.04901853436439296, 75.26362638851092868, 71.79194879392322548 ) ) ;
#14319=CARTESIAN_POINT ( 'NONE',  ( 91.23603883849618512, 78.43035437438882695, 30.82342686631244888 ) ) ;
#14320=CARTESIAN_POINT ( 'NONE',  ( -84.57230515545194294, 104.9999999999999858, -70.33944174062779098 ) ) ;
#14323=EDGE_CURVE ( 'NONE', #15796, #9955, #1099, .T. ) ;
#14325=DIRECTION ( 'NONE',  ( 0.9999164797902017066, 2.001050586450178695E-22, -0.01292414190464131508 ) ) ;
#14331=CARTESIAN_POINT ( 'NONE',  ( -38.46180957136326128, 93.08398165842332617, 84.42015501544445044 ) ) ;
#14342=ORIENTED_EDGE ( 'NONE', *, *, #4262, .F. ) ;
#14348=CARTESIAN_POINT ( 'NONE',  ( -91.47655718793627955, 79.89818662653908632, 31.35069918968696712 ) ) ;
#14349=CARTESIAN_POINT ( 'NONE',  ( -88.18368518054532501, 87.00751446224754204, 51.35601162712541168 ) ) ;
#14350=EDGE_LOOP ( 'NONE', ( #15046, #5723, #3269, #5264 ) ) ;
#14360=AXIS2_PLACEMENT_3D ( 'NONE', #16211, #14368, #19278 ) ;
#14368=DIRECTION ( 'NONE',  ( 0.9999164797902017066, 2.001050586450178695E-22, -0.01292414190464131508 ) ) ;
#14372=CARTESIAN_POINT ( 'NONE',  ( 39.40254987707581336, 92.58578643762697880, -84.93055112583749633 ) ) ;
#14373=CARTESIAN_POINT ( 'NONE',  ( 79.92740525950247843, 75.13699351169599083, -6.133505399301336425 ) ) ;
#14378=CARTESIAN_POINT ( 'NONE',  ( -39.42082737383933733, 91.17157287525387233, 83.51645567887779009 ) ) ;
#14379=CARTESIAN_POINT ( 'NONE',  ( -64.28883878761490678, 83.29019440189556178, 55.44125366118054643 ) ) ;
#14383=DIRECTION ( 'NONE',  ( 0.01292414190464131508, 0.000000000000000000, 0.9999164797902017066 ) ) ;
#14390=LINE ( 'NONE', #19632, #15034 ) ;
#14392=CARTESIAN_POINT ( 'NONE',  ( -90.00743053908078650, 87.70552466312305739, 50.96783830792826109 ) ) ;
#14395=EDGE_LOOP ( 'NONE', ( #5023, #4827, #15445, #19304 ) ) ;
#14405=FACE_OUTER_BOUND ( 'NONE', #65, .T. ) ;
#14407=CARTESIAN_POINT ( 'NONE',  ( 64.99457118636310327, 169.9999999999999716, -0.8400692238016950197 ) ) ;
#14409=CARTESIAN_POINT ( 'NONE',  ( -80.05923150692979107, 75.13699351169597662, -4.065642694558678549 ) ) ;
#14418=ORIENTED_EDGE ( 'NONE', *, *, #12599, .T. ) ;
#14422=ORIENTED_EDGE ( 'NONE', *, *, #15708, .F. ) ;
#14423=CARTESIAN_POINT ( 'NONE',  ( -105.2250167141420576, 70.47859713728956876, 32.05784361718416875 ) ) ;
#14426=ORIENTED_EDGE ( 'NONE', *, *, #13747, .F. ) ;
#14427=AXIS2_PLACEMENT_3D ( 'NONE', #9488, #15146, #6054 ) ;
#14429=CARTESIAN_POINT ( 'NONE',  ( 64.99457118636311748, 169.9999999999999716, -0.8400692238016952418 ) ) ;
#14432=CARTESIAN_POINT ( 'NONE',  ( -90.71810225913505121, 79.29666913609149503, -27.07744225877266331 ) ) ;
#14436=VECTOR ( 'NONE', #15522, 1000.000000000000000 ) ;
#14440=CARTESIAN_POINT ( 'NONE',  ( 83.95054225259531222, 104.7585062753441036, 71.08029813247935635 ) ) ;
#14446=ADVANCED_FACE ( 'NONE', ( #2814 ), #16839, .T. ) ;
#14447=DIRECTION ( 'NONE',  ( 0.009138748381789078140, -0.7071067811865487940, 0.7070477234798315802 ) ) ;
#14451=CARTESIAN_POINT ( 'NONE',  ( -93.21002351426730570, 79.82103140525721585, -28.79774562292282170 ) ) ;
#14459=AXIS2_PLACEMENT_3D ( 'NONE', #3713, #17523, #20825 ) ;
#14461=ADVANCED_FACE ( 'NONE', ( #1667 ), #21446, .F. ) ;
#14469=FACE_OUTER_BOUND ( 'NONE', #14350, .T. ) ;
#14470=FACE_OUTER_BOUND ( 'NONE', #9493, .T. ) ;
#14474=LINE ( 'NONE', #21438, #14003 ) ;
#14475=ORIENTED_EDGE ( 'NONE', *, *, #6493, .T. ) ;
#14476=DIRECTION ( 'NONE',  ( 0.9999164797902015955, 2.001050586450178695E-22, -0.01292414190464131335 ) ) ;
#14478=VERTEX_POINT ( 'NONE', #12000 ) ;
#14487=CARTESIAN_POINT ( 'NONE',  ( -37.83293359760840247, 93.41702043942370892, 84.07896005544418472 ) ) ;
#14488=DIRECTION ( 'NONE',  ( 0.9999164797902015955, 2.001050586450178695E-22, -0.01292414190464131335 ) ) ;
#14492=VERTEX_POINT ( 'NONE', #8313 ) ;
#14498=CARTESIAN_POINT ( 'NONE',  ( -105.4334892372614121, 72.00000000000000000, 31.36525700924958926 ) ) ;
#14504=EDGE_CURVE ( 'NONE', #13316, #10917, #8535, .T. ) ;
#14511=EDGE_LOOP ( 'NONE', ( #5160, #9443, #3372 ) ) ;
#14515=DIRECTION ( 'NONE',  ( -0.9999164797902017066, -2.001050586450178931E-22, 0.01292414190464131508 ) ) ;
#14516=CARTESIAN_POINT ( 'NONE',  ( -90.75111155332035651, 98.75957274858885171, -62.16377225325074818 ) ) ;
#14525=DIRECTION ( 'NONE',  ( -2.025474946048326158E-22, 1.000000000000000000, -1.876735158486679638E-22 ) ) ;
#14529=ADVANCED_FACE ( 'NONE', ( #17073 ), #12113, .F. ) ;
#14534=CARTESIAN_POINT ( 'NONE',  ( -84.80959639660540006, 75.01379216013428675, 2.744183072880618468 ) ) ;
#14536=ORIENTED_EDGE ( 'NONE', *, *, #12120, .T. ) ;
#14540=CARTESIAN_POINT ( 'NONE',  ( -91.00106904273528130, 70.29040131071506892, 61.79648398638329354 ) ) ;
#14542=VERTEX_POINT ( 'NONE', #15246 ) ;
#14547=CARTESIAN_POINT ( 'NONE',  ( 91.87497954589152016, 77.44324451750787830, 29.32612497091767878 ) ) ;
#14550=CARTESIAN_POINT ( 'NONE',  ( -93.23587179807654479, 72.00000000000000000, -30.79757858250321689 ) ) ;
#14557=B_SPLINE_CURVE_WITH_KNOTS ( 'NONE', 3,
 ( #14200, #21174, #16041, #3838, #278, #5427 ),
 .UNSPECIFIED., .F., .F.,
 ( 4, 2, 4 ),
 ( 0.001327491350857572250, 0.002295428894073542163, 0.003263366437289511642 ),
 .UNSPECIFIED. ) ;
#14559=EDGE_CURVE ( 'NONE', #7441, #8239, #1283, .T. ) ;
#14561=CARTESIAN_POINT ( 'NONE',  ( 74.93593926291724472, 75.00181558815791050, -0.2967849484207667476 ) ) ;
#14563=ORIENTED_EDGE ( 'NONE', *, *, #20735, .F. ) ;
#14571=CARTESIAN_POINT ( 'NONE',  ( -68.71681667565952978, 91.17157287525388654, 85.89527988174785378 ) ) ;
#14575=CARTESIAN_POINT ( 'NONE',  ( 68.50871000753478768, 71.18193548034264495, -86.06142760398537916 ) ) ;
#14577=CARTESIAN_POINT ( 'NONE',  ( -89.76942472236369497, 79.35227432041517659, 29.58847612530658111 ) ) ;
#14583=ORIENTED_EDGE ( 'NONE', *, *, #11899, .F. ) ;
#14586=DIRECTION ( 'NONE',  ( 0.01292414190464174703, 0.000000000000000000, 0.9999164797902015955 ) ) ;
#14590=ORIENTED_EDGE ( 'NONE', *, *, #541, .T. ) ;
#14593=CARTESIAN_POINT ( 'NONE',  ( -34.61804907780420137, 94.93197183469658285, 82.52232902628021805 ) ) ;
#14599=EDGE_CURVE ( 'NONE', #2340, #3568, #7873, .T. ) ;
#14602=ORIENTED_EDGE ( 'NONE', *, *, #13562, .T. ) ;
#14603=CARTESIAN_POINT ( 'NONE',  ( -71.30561357180762627, 88.42313952667566923, 69.70915026362466449 ) ) ;
#14607=CARTESIAN_POINT ( 'NONE',  ( 0.2091060127835376314, 86.14731717667953603, 75.00341234062101137 ) ) ;
#14610=EDGE_CURVE ( 'NONE', #14478, #11658, #14134, .T. ) ;
#14612=CARTESIAN_POINT ( 'NONE',  ( -91.62437796271721879, 34.61572286322119396, -60.86849236629028326 ) ) ;
#14613=CARTESIAN_POINT ( 'NONE',  ( -89.27750275332233798, 88.44712234866830158, 50.50536220203945703 ) ) ;
#14617=CARTESIAN_POINT ( 'NONE',  ( 36.55288090549195346, 94.02752048664900997, -83.45186405039071076 ) ) ;
#14619=VERTEX_POINT ( 'NONE', #17973 ) ;
#14623=CARTESIAN_POINT ( 'NONE',  ( -39.75021781620441885, 69.99999999999998579, -86.03367798009510636 ) ) ;
#14625=CARTESIAN_POINT ( 'NONE',  ( -91.26258897903520051, 97.45270810253440175, -61.41003422490167196 ) ) ;
#14630=CARTESIAN_POINT ( 'NONE',  ( -109.6363981638670566, 79.04398536104964990, 28.84204567386064255 ) ) ;
#14631=CARTESIAN_POINT ( 'NONE',  ( -92.13597290369312987, 77.31823782845361848, -29.12178019517726213 ) ) ;
#14636=FACE_OUTER_BOUND ( 'NONE', #1751, .T. ) ;
#14640=ORIENTED_EDGE ( 'NONE', *, *, #8301, .T. ) ;
#14645=CARTESIAN_POINT ( 'NONE',  ( -85.08821190676783885, 75.00001493645879691, 1.440439948039162088 ) ) ;
#14652=CARTESIAN_POINT ( 'NONE',  ( -41.61793149762837629, 72.00000000000000000, -86.46934588545651934 ) ) ;
#14654=CARTESIAN_POINT ( 'NONE',  ( -89.99332827844999372, 79.52815953299852936, -27.82019389467126658 ) ) ;
#14655=CARTESIAN_POINT ( 'NONE',  ( 70.22615711568096231, 70.59893530615325119, 84.66585046671892201 ) ) ;
#14656=ADVANCED_FACE ( 'NONE', ( #4041 ), #2809, .T. ) ;
#14662=CARTESIAN_POINT ( 'NONE',  ( 93.13093775432295729, 79.82103140525535423, 28.79876782389523271 ) ) ;
#14666=CYLINDRICAL_SURFACE ( 'NONE', #9586, 2.000000000000004885 ) ;
#14674=CARTESIAN_POINT ( 'NONE',  ( 78.41260081656773195, 75.12325561942539309, 3.826278609843483114 ) ) ;
#14679=DIRECTION ( 'NONE',  ( -0.01292414190463827932, 0.000000000000000000, -0.9999164797902018176 ) ) ;
#14681=DIRECTION ( 'NONE',  ( 2.025474946048326158E-22, -1.000000000000000000, 1.876735158486679638E-22 ) ) ;
#14687=CARTESIAN_POINT ( 'NONE',  ( 92.35396912051041340, 79.82103140542857034, -31.19620131593210388 ) ) ;
#14690=CARTESIAN_POINT ( 'NONE',  ( -90.40889375659911309, 78.43035437438882695, 33.17122784026039994 ) ) ;
#14697=ORIENTED_EDGE ( 'NONE', *, *, #9581, .F. ) ;
#14698=CARTESIAN_POINT ( 'NONE',  ( 106.2089377515399065, 72.00000000000000000, 28.62973177816241588 ) ) ;
#14705=CARTESIAN_POINT ( 'NONE',  ( -34.11225069749754368, 94.37751527644309135, 83.07029434066950557 ) ) ;
#14709=EDGE_CURVE ( 'NONE', #18446, #4308, #3088, .T. ) ;
#14711=DIRECTION ( 'NONE',  ( 0.8588562297929587253, 0.3902276408394437790, -0.3317956673477015506 ) ) ;
#14714=ORIENTED_EDGE ( 'NONE', *, *, #1131, .F. ) ;
#14723=AXIS2_PLACEMENT_3D ( 'NONE', #22082, #4528, #9470 ) ;
#14725=CARTESIAN_POINT ( 'NONE',  ( -64.14629883989944403, 91.30780077822167584, 66.46930053661340310 ) ) ;
#14729=LINE ( 'NONE', #14612, #20188 ) ;
#14730=CARTESIAN_POINT ( 'NONE',  ( -88.18706637290718220, 88.71869973106700513, 50.32066939225164504 ) ) ;
#14741=CARTESIAN_POINT ( 'NONE',  ( -75.30975508861040169, 94.90914755154933857, 80.17755788556743823 ) ) ;
#14742=CARTESIAN_POINT ( 'NONE',  ( 91.62437796271727564, 95.44063823554748183, 60.86849236629024773 ) ) ;
#14744=CARTESIAN_POINT ( 'NONE',  ( 37.51330139321492396, 72.00000000000000000, -87.03232607370792095 ) ) ;
#14745=CARTESIAN_POINT ( 'NONE',  ( -91.62437796271721879, 95.44063823554751025, -60.86849236629028326 ) ) ;
#14746=ORIENTED_EDGE ( 'NONE', *, *, #18315, .T. ) ;
#14752=CARTESIAN_POINT ( 'NONE',  ( -91.65137210734575035, 77.59584042966187667, -29.57018005965453611 ) ) ;
#14754=CARTESIAN_POINT ( 'NONE',  ( -37.51330139321489554, 69.99999999999998579, 87.03232607370787832 ) ) ;
#14762=ORIENTED_EDGE ( 'NONE', *, *, #8333, .F. ) ;
#14763=CARTESIAN_POINT ( 'NONE',  ( -80.05923150692979107, 75.13699351169597662, -4.065642694558678549 ) ) ;
#14765=EDGE_CURVE ( 'NONE', #11360, #9297, #554, .T. ) ;
#14768=ORIENTED_EDGE ( 'NONE', *, *, #10213, .T. ) ;
#14770=VERTEX_POINT ( 'NONE', #22349 ) ;
#14774=CARTESIAN_POINT ( 'NONE',  ( -39.99341017482546334, 93.41702043935060829, -83.07303732980588507 ) ) ;
#14788=ORIENTED_EDGE ( 'NONE', *, *, #1938, .T. ) ;
#14791=ORIENTED_EDGE ( 'NONE', *, *, #8058, .T. ) ;
#14797=ADVANCED_FACE ( 'NONE', ( #1155 ), #22244, .T. ) ;
#14799=CARTESIAN_POINT ( 'NONE',  ( -63.92582232734818604, 91.13550884953522768, 66.60804284595937474 ) ) ;
#14803=CARTESIAN_POINT ( 'NONE',  ( -69.43142427201328815, 92.58578643762699301, 85.31868097644080251 ) ) ;
#14809=CARTESIAN_POINT ( 'NONE',  ( 91.77247882320288852, 77.19421037201389879, -31.29629296515013692 ) ) ;
#14813=LINE ( 'NONE', #11453, #5559 ) ;
#14814=DIRECTION ( 'NONE',  ( -0.9999164797902015955, -2.001050586450178695E-22, 0.01292414190464131335 ) ) ;
#14819=DIRECTION ( 'NONE',  ( -2.025474946048326158E-22, 1.000000000000000000, -1.876735158486679638E-22 ) ) ;
#14820=AXIS2_PLACEMENT_3D ( 'NONE', #197, #15834, #7078 ) ;
#14821=AXIS2_PLACEMENT_3D ( 'NONE', #19586, #13976, #19472 ) ;
#14822=CYLINDRICAL_SURFACE ( 'NONE', #2671, 1.999999999999997780 ) ;
#14834=CARTESIAN_POINT ( 'NONE',  ( -24.45368655303012417, 89.79783256935353108, 79.21683296045429756 ) ) ;
#14836=VERTEX_POINT ( 'NONE', #20654 ) ;
#14840=ORIENTED_EDGE ( 'NONE', *, *, #13297, .T. ) ;
#14845=CARTESIAN_POINT ( 'NONE',  ( -88.17134115317794851, 88.83281691486382670, 52.17357975332178910 ) ) ;
#14848=CIRCLE ( 'NONE', #3823, 95.00000000000004263 ) ;
#14849=ORIENTED_EDGE ( 'NONE', *, *, #4314, .F. ) ;
#14856=DIRECTION ( 'NONE',  ( 2.025474946048326158E-22, -1.000000000000000000, 1.876735158486679638E-22 ) ) ;
#14857=DIRECTION ( 'NONE',  ( -0.9999164797902015955, 0.000000000000000000, 0.01292414190464218071 ) ) ;
#14859=CARTESIAN_POINT ( 'NONE',  ( -1.163172771417704698, 69.99999999999998579, -89.99248318111816047 ) ) ;
#14862=CARTESIAN_POINT ( 'NONE',  ( 34.23466015841589183, 93.68133903400143936, -83.10361438825003688 ) ) ;
#14863=VERTEX_POINT ( 'NONE', #13449 ) ;
#14869=EDGE_CURVE ( 'NONE', #7249, #9044, #20418, .T. ) ;
#14877=ORIENTED_EDGE ( 'NONE', *, *, #15408, .F. ) ;
#14879=CARTESIAN_POINT ( 'NONE',  ( -105.4334892372614121, 72.00000000000000000, 31.36525700924958926 ) ) ;
#14880=CARTESIAN_POINT ( 'NONE',  ( -90.10851746777733240, 88.45132993515882447, 52.79029924855479550 ) ) ;
#14892=ORIENTED_EDGE ( 'NONE', *, *, #18557, .T. ) ;
#14895=DIRECTION ( 'NONE',  ( 0.01292414190463832269, 0.000000000000000000, 0.9999164797902017066 ) ) ;
#14898=CARTESIAN_POINT ( 'NONE',  ( 73.81922676008082362, 96.21294322789840692, -81.74793453868313975 ) ) ;
#14913=CARTESIAN_POINT ( 'NONE',  ( 76.93439171139391419, 75.08638595516887904, 3.060657608357647774 ) ) ;
#14915=DIRECTION ( 'NONE',  ( -0.8588562297929586142, -0.3902276408394423912, 0.3317956673477029383 ) ) ;
#14918=CARTESIAN_POINT ( 'NONE',  ( -39.39497909003006981, 91.17157287525388654, 85.51628863845817818 ) ) ;
#14924=CARTESIAN_POINT ( 'NONE',  ( 90.65029634199440522, 79.17021053268413766, -29.01211804384235649 ) ) ;
#14930=ORIENTED_EDGE ( 'NONE', *, *, #21843, .T. ) ;
#14947=CARTESIAN_POINT ( 'NONE',  ( 16.25138420224134705, 87.34880441414898655, 76.12342506946350795 ) ) ;
#14953=CARTESIAN_POINT ( 'NONE',  ( -89.44439933878480531, 89.11516110322091322, 51.58556162172175164 ) ) ;
#14955=ORIENTED_EDGE ( 'NONE', *, *, #1948, .F. ) ;
#14958=EDGE_LOOP ( 'NONE', ( #12943, #9801, #11869, #6594 ) ) ;
#14964=CARTESIAN_POINT ( 'NONE',  ( 35.60052562348057137, 93.98891615189143067, -83.40426226564440526 ) ) ;
#14967=CARTESIAN_POINT ( 'NONE',  ( -92.02038759195845330, 72.00000000000000000, 63.24214162404745565 ) ) ;
#14971=AXIS2_PLACEMENT_3D ( 'NONE', #12554, #3476, #21255 ) ;
#14978=EDGE_CURVE ( 'NONE', #9627, #4929, #4835, .T. ) ;
#14979=CARTESIAN_POINT ( 'NONE',  ( -88.16225667628052065, 88.12760352708744449, 53.01283023165030528 ) ) ;
#14982=ORIENTED_EDGE ( 'NONE', *, *, #22384, .F. ) ;
#14986=CARTESIAN_POINT ( 'NONE',  ( -67.76708237988898986, 98.06134765687328070, 76.92491524063726160 ) ) ;
#14992=LINE ( 'NONE', #13492, #10636 ) ;
#14993=DIRECTION ( 'NONE',  ( -0.9999164797902015955, -2.001050586450177755E-22, 0.01292414190464177999 ) ) ;
#15005=EDGE_CURVE ( 'NONE', #12564, #11300, #1820, .T. ) ;
#15009=VECTOR ( 'NONE', #10246, 1000.000000000000000 ) ;
#15011=EDGE_CURVE ( 'NONE', #6632, #22379, #17650, .T. ) ;
#15012=CARTESIAN_POINT ( 'NONE',  ( 77.82328986082669076, 75.11365078037778176, -5.652215941475883909 ) ) ;
#15013=CARTESIAN_POINT ( 'NONE',  ( -91.01151104332689101, 70.28404947875058895, 61.80376916000803789 ) ) ;
#15014=CIRCLE ( 'NONE', #5073, 2.000000000000004441 ) ;
#15022=CARTESIAN_POINT ( 'NONE',  ( 89.99012571735545407, 95.97180966979294681, -63.25964760396028908 ) ) ;
#15025=CARTESIAN_POINT ( 'NONE',  ( 89.23446290093956179, 79.53212074382834373, -30.14913290299190862 ) ) ;
#15027=FACE_OUTER_BOUND ( 'NONE', #2023, .T. ) ;
#15031=ORIENTED_EDGE ( 'NONE', *, *, #21546, .F. ) ;
#15034=VECTOR ( 'NONE', #2078, 1000.000000000000114 ) ;
#15036=ORIENTED_EDGE ( 'NONE', *, *, #16991, .T. ) ;
#15038=CARTESIAN_POINT ( 'NONE',  ( -67.64952533873930918, 70.35418627987228035, 86.73849053056652281 ) ) ;
#15046=ORIENTED_EDGE ( 'NONE', *, *, #13747, .T. ) ;
#15047=CARTESIAN_POINT ( 'NONE',  ( -106.2343493168401949, 77.75544475269062161, -28.53532068555761825 ) ) ;
#15052=TOROIDAL_SURFACE ( 'NONE', #17239, 4.000000000000000000, 2.000000000000000000 ) ;
#15062=ADVANCED_FACE ( 'NONE', ( #21544 ), #3879, .F. ) ;
#15065=CARTESIAN_POINT ( 'NONE',  ( 91.73057767193266443, 77.20311952920094711, -31.31041951043028604 ) ) ;
#15074=DIRECTION ( 'NONE',  ( -0.01292414190464137060, 0.000000000000000000, -0.9999164797902015955 ) ) ;
#15077=EDGE_LOOP ( 'NONE', ( #13749, #316, #6906, #4874 ) ) ;
#15078=DIRECTION ( 'NONE',  ( -0.9999164797902017066, -1.471961700026549794E-14, 0.01292414190464131508 ) ) ;
#15081=CARTESIAN_POINT ( 'NONE',  ( 93.23587179807657321, 34.61572286322119396, 30.79757858250317071 ) ) ;
#15087=DIRECTION ( 'NONE',  ( 2.081668171172166620E-14, 1.000000000000000000, 0.000000000000000000 ) ) ;
#15089=VERTEX_POINT ( 'NONE', #5815 ) ;
#15093=VECTOR ( 'NONE', #15829, 1000.000000000000114 ) ;
#15095=CARTESIAN_POINT ( 'NONE',  ( -88.16354289163604108, 88.27034599685696037, 52.90680319025804579 ) ) ;
#15104=DIRECTION ( 'NONE',  ( 2.025474946048326158E-22, -1.000000000000000000, 1.876735158486679638E-22 ) ) ;
#15105=CARTESIAN_POINT ( 'NONE',  ( -71.06083360305757424, 91.87225009003576304, -83.96645210693647243 ) ) ;
#15108=B_SPLINE_CURVE_WITH_KNOTS ( 'NONE', 3,
 ( #21479, #1981, #8971, #10830, #17854, #21250, #2434, #10933, #21580, #601, #18071, #2090, #2319, #9074, #9318, #7592 ),
 .UNSPECIFIED., .F., .F.,
 ( 4, 2, 2, 2, 2, 2, 2, 4 ),
 ( 0.000000000000000000, 0.0008607555596716533631, 0.001291133339507492730, 0.001721511119343332097, 0.002151888899179171463, 0.002582266679015010613, 0.003012644458850850197, 0.003443022238686689347 ),
 .UNSPECIFIED. ) ;
#15111=CARTESIAN_POINT ( 'NONE',  ( 93.17671387018316409, 79.04398536104953621, 26.22064129356657602 ) ) ;
#15116=AXIS2_PLACEMENT_3D ( 'NONE', #7935, #15078, #1049 ) ;
#15124=ORIENTED_EDGE ( 'NONE', *, *, #20185, .T. ) ;
#15126=DIRECTION ( 'NONE',  ( 2.025474946048326158E-22, -1.000000000000000000, 1.876735158486679638E-22 ) ) ;
#15136=CARTESIAN_POINT ( 'NONE',  ( 105.7487010638476335, 78.91327849199113587, -30.28586431387813960 ) ) ;
#15138=CIRCLE ( 'NONE', #8502, 2.000000000000005773 ) ;
#15140=CARTESIAN_POINT ( 'NONE',  ( -91.23603883849614249, 72.00000000000000000, -30.82342686631250217 ) ) ;
#15144=ADVANCED_FACE ( 'NONE', ( #7784 ), #14822, .T. ) ;
#15145=CARTESIAN_POINT ( 'NONE',  ( 90.81765045018462956, 77.62753381201262926, -31.97827203367606330 ) ) ;
#15146=DIRECTION ( 'NONE',  ( -2.025474946048326158E-22, 1.000000000000000000, -1.876735158486679638E-22 ) ) ;
#15158=CARTESIAN_POINT ( 'NONE',  ( -68.71681667565952978, 72.00000000000000000, 85.89527988174785378 ) ) ;
#15163=AXIS2_PLACEMENT_3D ( 'NONE', #16980, #2607, #16522 ) ;
#15164=CARTESIAN_POINT ( 'NONE',  ( -1.421655609510530827, 45.00000000000000000, -109.9908127769221835 ) ) ;
#15166=DIRECTION ( 'NONE',  ( 0.01292414190464131682, 1.902755938799531179E-22, 0.9999164797902017066 ) ) ;
#15167=ORIENTED_EDGE ( 'NONE', *, *, #240, .T. ) ;
#15172=DIRECTION ( 'NONE',  ( -2.025474946048326393E-22, 1.000000000000000000, -1.876735158486679873E-22 ) ) ;
#15184=EDGE_CURVE ( 'NONE', #2836, #22275, #4396, .T. ) ;
#15189=DIRECTION ( 'NONE',  ( 2.025474946048326158E-22, -1.000000000000000000, 1.876735158486679638E-22 ) ) ;
#15190=DIRECTION ( 'NONE',  ( 2.025474946048326158E-22, -1.000000000000000000, 1.876735158486679638E-22 ) ) ;
#15201=CARTESIAN_POINT ( 'NONE',  ( -65.91440269377939387, 105.0000000000000000, -70.32555938675406537 ) ) ;
#15202=LINE ( 'NONE', #3103, #9301 ) ;
#15203=DIRECTION ( 'NONE',  ( -2.025474946048326158E-22, 1.000000000000000000, -1.876735158486679638E-22 ) ) ;
#15205=ADVANCED_FACE ( 'NONE', ( #16865, #20167 ), #22109, .F. ) ;
#15210=VERTEX_POINT ( 'NONE', #11688 ) ;
#15217=CARTESIAN_POINT ( 'NONE',  ( -88.16559194503513197, 88.46308404799054870, 52.72753900144177663 ) ) ;
#15218=EDGE_LOOP ( 'NONE', ( #14422, #21909 ) ) ;
#15222=CARTESIAN_POINT ( 'NONE',  ( 91.62437796271727564, 72.00000000000000000, 60.86849236629024773 ) ) ;
#15224=ORIENTED_EDGE ( 'NONE', *, *, #6888, .F. ) ;
#15231=LINE ( 'NONE', #22287, #16181 ) ;
#15233=LINE ( 'NONE', #20363, #2107 ) ;
#15234=VECTOR ( 'NONE', #4539, 1000.000000000000114 ) ;
#15236=VECTOR ( 'NONE', #20717, 1000.000000000000000 ) ;
#15241=CARTESIAN_POINT ( 'NONE',  ( -64.03068742478980369, 99.72761617120355027, 75.41393764079656137 ) ) ;
#15246=CARTESIAN_POINT ( 'NONE',  ( -80.05923150692979107, 75.13699351169597662, -4.065642694558678549 ) ) ;
#15248=EDGE_LOOP ( 'NONE', ( #10964, #1033, #12079, #22298 ) ) ;
#15250=CARTESIAN_POINT ( 'NONE',  ( 1.364373935098378649E-14, 105.0000000000000000, -9.836450281572198869E-15 ) ) ;
#15251=CARTESIAN_POINT ( 'NONE',  ( -107.2806549642561436, 77.80407930632172508, 24.41717176243129828 ) ) ;
#15252=CARTESIAN_POINT ( 'NONE',  ( -89.22767861003021039, 80.31838830481383695, -30.18953644180660234 ) ) ;
#15253=CARTESIAN_POINT ( 'NONE',  ( -92.50365291375118204, 70.32755610701403270, -59.52398455131075394 ) ) ;
#15258=CIRCLE ( 'NONE', #13759, 2.000000000000000000 ) ;
#15260=DIRECTION ( 'NONE',  ( 0.9999164797902015955, 2.001050586450179636E-22, -0.01292414190464084844 ) ) ;
#15261=FACE_OUTER_BOUND ( 'NONE', #1171, .T. ) ;
#15262=CARTESIAN_POINT ( 'NONE',  ( 92.89382307712753573, 70.12557134413806637, 58.91325363510484436 ) ) ;
#15265=ORIENTED_EDGE ( 'NONE', *, *, #6112, .F. ) ;
#15273=CARTESIAN_POINT ( 'NONE',  ( -68.50871000753471662, 71.18193548034264495, 86.06142760398536495 ) ) ;
#15275=EDGE_CURVE ( 'NONE', #16549, #19747, #22061, .T. ) ;
#15278=EDGE_CURVE ( 'NONE', #6286, #19552, #9073, .T. ) ;
#15280=FACE_OUTER_BOUND ( 'NONE', #19805, .T. ) ;
#15286=ORIENTED_EDGE ( 'NONE', *, *, #11482, .F. ) ;
#15290=LINE ( 'NONE', #13214, #22193 ) ;
#15293=LINE ( 'NONE', #16779, #5842 ) ;
#15294=CARTESIAN_POINT ( 'NONE',  ( -109.9908127769221693, 169.9999999999999716, 1.421655609510535045 ) ) ;
#15295=DIRECTION ( 'NONE',  ( 0.01292414190464523903, 0.000000000000000000, 0.9999164797902017066 ) ) ;
#15296=EDGE_CURVE ( 'NONE', #9610, #22618, #5220, .T. ) ;
#15300=ADVANCED_FACE ( 'NONE', ( #12138 ), #1792, .F. ) ;
#15307=ORIENTED_EDGE ( 'NONE', *, *, #6118, .T. ) ;
#15312=CARTESIAN_POINT ( 'NONE',  ( -90.82246629754762068, 169.9999999999999716, 1.173900486973953772 ) ) ;
#15315=EDGE_CURVE ( 'NONE', #10332, #17177, #8772, .T. ) ;
#15319=CARTESIAN_POINT ( 'NONE',  ( -63.92222308695259869, 94.02752048664899576, 83.80561885825630952 ) ) ;
#15323=CARTESIAN_POINT ( 'NONE',  ( -90.15472117445577283, 87.25778962232662650, 51.24158970824034043 ) ) ;
#15327=PLANE ( 'NONE',  #21307 ) ;
#15328=DIRECTION ( 'NONE',  ( -0.01292414190464217898, -1.902755938799531885E-22, -0.9999164797902015955 ) ) ;
#15329=DIRECTION ( 'NONE',  ( -0.01292414190464218071, 9.204123485805280727E-39, -0.9999164797902015955 ) ) ;
#15330=CARTESIAN_POINT ( 'NONE',  ( 82.21743679224594814, 104.4142135623730923, -73.65452789938869671 ) ) ;
#15331=CARTESIAN_POINT ( 'NONE',  ( -88.42085790543279700, 80.22997387171260186, 32.23265953185128296 ) ) ;
#15336=CARTESIAN_POINT ( 'NONE',  ( -90.02055463237803679, 72.00000000000000000, 63.21629334023816682 ) ) ;
#15337=CARTESIAN_POINT ( 'NONE',  ( 88.41758806590424058, 80.31838830481383695, -32.48564084813595798 ) ) ;
#15344=VERTEX_POINT ( 'NONE', #6947 ) ;
#15349=CARTESIAN_POINT ( 'NONE',  ( -88.73586072705668926, 70.68102025985758985, 62.80242633408442288 ) ) ;
#15350=EDGE_LOOP ( 'NONE', ( #19353, #20953, #18733, #8219 ) ) ;
#15357=B_SPLINE_CURVE_WITH_KNOTS ( 'NONE', 3,
 ( #59, #7178, #5213, #17885, #3502, #2117, #17773, #17989, #403, #285, #3609, #13959, #8760, #2015, #14092, #17531, #7400, #9112 ),
 .UNSPECIFIED., .F., .F.,
 ( 4, 2, 2, 2, 2, 2, 2, 2, 4 ),
 ( 0.000000000000000000, 0.0008023074076923169054, 0.001604614815384633811, 0.002406922223076950716, 0.003209229630769267622, 0.004011537038461584527, 0.004813844446153901432, 0.005616151853846218338, 0.006418459261538535243 ),
 .UNSPECIFIED. ) ;
#15366=CARTESIAN_POINT ( 'NONE',  ( 90.40889375659914151, 78.43035437438882695, -33.17122784026044258 ) ) ;
#15367=ORIENTED_EDGE ( 'NONE', *, *, #10604, .F. ) ;
#15369=ORIENTED_EDGE ( 'NONE', *, *, #10604, .T. ) ;
#15385=ORIENTED_EDGE ( 'NONE', *, *, #15664, .T. ) ;
#15387=ORIENTED_EDGE ( 'NONE', *, *, #15989, .T. ) ;
#15388=CARTESIAN_POINT ( 'NONE',  ( 107.2806549642561293, 77.80407930632178193, -24.41717176243149723 ) ) ;
#15389=CIRCLE ( 'NONE', #17204, 1.999999999999997780 ) ;
#15401=DIRECTION ( 'NONE',  ( -2.025474946048326158E-22, 1.000000000000000000, -1.876735158486679638E-22 ) ) ;
#15408=EDGE_CURVE ( 'NONE', #14017, #2340, #14217, .T. ) ;
#15419=CARTESIAN_POINT ( 'NONE',  ( 92.46788464407293873, 79.04398536104962147, -28.62013883513330015 ) ) ;
#15420=CARTESIAN_POINT ( 'NONE',  ( 106.1347175484142724, 70.98259407754899541, 28.90376667366504293 ) ) ;
#15426=VECTOR ( 'NONE', #12845, 1000.000000000000114 ) ;
#15433=CARTESIAN_POINT ( 'NONE',  ( -90.04453709701007824, 88.62965799390647703, 52.60395590584802505 ) ) ;
#15436=CARTESIAN_POINT ( 'NONE',  ( -74.05286932419430457, 95.97475531906495405, 81.34035317851895286 ) ) ;
#15439=CARTESIAN_POINT ( 'NONE',  ( 41.61793149762840471, 72.00000000000000000, 86.46934588545650513 ) ) ;
#15441=CARTESIAN_POINT ( 'NONE',  ( -88.16157026904451754, 88.04290212818517602, 53.06700061362226961 ) ) ;
#15443=CARTESIAN_POINT ( 'NONE',  ( -91.15750879531698558, 79.10636023297634267, 28.80946033575589027 ) ) ;
#15444=CARTESIAN_POINT ( 'NONE',  ( -71.51920288841773754, 92.50622980579329635, -83.57642618781949295 ) ) ;
#15445=ORIENTED_EDGE ( 'NONE', *, *, #952, .F. ) ;
#15446=AXIS2_PLACEMENT_3D ( 'NONE', #3874, #3638, #21441 ) ;
#15449=CARTESIAN_POINT ( 'NONE',  ( 1.421655609510571683, 69.99999999999998579, 109.9908127769221409 ) ) ;
#15450=CARTESIAN_POINT ( 'NONE',  ( 91.41602376139165642, 79.08283919787463390, -28.73514828341266281 ) ) ;
#15452=CYLINDRICAL_SURFACE ( 'NONE', #7346, 85.00000000000001421 ) ;
#15460=CARTESIAN_POINT ( 'NONE',  ( -64.01907823019016064, 100.1566401219223081, 76.31211912804367614 ) ) ;
#15461=ORIENTED_EDGE ( 'NONE', *, *, #15275, .F. ) ;
#15462=EDGE_LOOP ( 'NONE', ( #694, #17726, #9217 ) ) ;
#15468=CARTESIAN_POINT ( 'NONE',  ( 78.59956642649036951, 75.12824275668153007, -5.951310493065621543 ) ) ;
#15469=CARTESIAN_POINT ( 'NONE',  ( -85.84563054365271739, 105.0000000000000142, -68.77965573371086805 ) ) ;
#15470=CARTESIAN_POINT ( 'NONE',  ( 105.4334892372614405, 77.28905753105605925, -31.36525700924962834 ) ) ;
#15475=ORIENTED_EDGE ( 'NONE', *, *, #20695, .F. ) ;
#15478=VECTOR ( 'NONE', #1070, 1000.000000000000114 ) ;
#15481=VERTEX_POINT ( 'NONE', #16061 ) ;
#15483=CIRCLE ( 'NONE', #12896, 2.000000000000004885 ) ;
#15489=CARTESIAN_POINT ( 'NONE',  ( -72.50839346369934901, 87.61416393227378308, 70.38952438936911449 ) ) ;
#15498=ORIENTED_EDGE ( 'NONE', *, *, #9930, .F. ) ;
#15500=AXIS2_PLACEMENT_3D ( 'NONE', #5153, #21129, #10460 ) ;
#15501=AXIS2_PLACEMENT_3D ( 'NONE', #14378, #10807, #19622 ) ;
#15505=EDGE_CURVE ( 'NONE', #4929, #12, #5129, .T. ) ;
#15518=EDGE_LOOP ( 'NONE', ( #17957, #913, #12096, #16196 ) ) ;
#15522=DIRECTION ( 'NONE',  ( -2.025474946048326393E-22, 1.000000000000000000, -1.876735158486679873E-22 ) ) ;
#15527=CARTESIAN_POINT ( 'NONE',  ( -90.17340840076944630, 87.01269140061864960, 51.39028561451661403 ) ) ;
#15530=CARTESIAN_POINT ( 'NONE',  ( 106.1801133998813356, 71.34284122058939204, 28.73649967668635696 ) ) ;
#15541=ORIENTED_EDGE ( 'NONE', *, *, #12940, .T. ) ;
#15542=CARTESIAN_POINT ( 'NONE',  ( 90.02753699123907438, 71.81067029327459750, -63.20635338325894281 ) ) ;
#15543=CARTESIAN_POINT ( 'NONE',  ( -89.94245242475622604, 88.81374284693771415, 52.36835579984497002 ) ) ;
#15544=DIRECTION ( 'NONE',  ( -0.01292414190463830014, 0.000000000000000000, -0.9999164797902017066 ) ) ;
#15554=CARTESIAN_POINT ( 'NONE',  ( 82.74584346241131527, 75.09876982897527853, 3.262718563837641472 ) ) ;
#15560=SPHERICAL_SURFACE ( 'NONE', #15501, 2.000000000000000000 ) ;
#15566=CARTESIAN_POINT ( 'NONE',  ( -38.46706438352712354, 91.17157287525387233, 85.27439087629284131 ) ) ;
#15570=EDGE_CURVE ( 'NONE', #3568, #1373, #7352, .T. ) ;
#15574=EDGE_CURVE ( 'NONE', #10247, #1581, #4349, .T. ) ;
#15575=CARTESIAN_POINT ( 'NONE',  ( -88.73541651539278519, 70.70236138404430903, 62.83679415258478684 ) ) ;
#15576=AXIS2_PLACEMENT_3D ( 'NONE', #14967, #13466, #20437 ) ;
#15580=TOROIDAL_SURFACE ( 'NONE', #19212, 97.00000000000004263, 2.000000000000000000 ) ;
#15581=CARTESIAN_POINT ( 'NONE',  ( 63.61168800256650258, 69.99999999999997158, -107.8311325613533285 ) ) ;
#15588=DIRECTION ( 'NONE',  ( -2.025474946048326158E-22, 1.000000000000000000, -1.876735158486679638E-22 ) ) ;
#15599=VECTOR ( 'NONE', #9719, 1000.000000000000000 ) ;
#15606=ADVANCED_FACE ( 'NONE', ( #20815 ), #12345, .T. ) ;
#15607=CARTESIAN_POINT ( 'NONE',  ( -92.43457499998879712, 77.12912189496637438, 31.19724316448926160 ) ) ;
#15610=DIRECTION ( 'NONE',  ( 2.025474946048326158E-22, -1.000000000000000000, 1.876735158486679638E-22 ) ) ;
#15611=CARTESIAN_POINT ( 'NONE',  ( -41.56623493000981284, 91.17157287525390075, -82.46967996629571473 ) ) ;
#15612=ORIENTED_EDGE ( 'NONE', *, *, #8417, .F. ) ;
#15613=CARTESIAN_POINT ( 'NONE',  ( 109.9283388797386039, 75.00188554563108312, -6.129144436280934194 ) ) ;
#15616=ORIENTED_EDGE ( 'NONE', *, *, #16352, .F. ) ;
#15619=B_SPLINE_CURVE_WITH_KNOTS ( 'NONE', 3,
 ( #18483, #22121, #11251, #21888, #6184, #16772, #13210, #18159, #9398, #16436, #1019, #8013, #15047, #11591, #18586, #17002 ),
 .UNSPECIFIED., .F., .F.,
 ( 4, 2, 2, 2, 2, 2, 2, 4 ),
 ( 0.000000000000000000, 0.0004729024035692847407, 0.0009458048071385694814, 0.001891609614277118797, 0.002364512017846376758, 0.002837414421415635369, 0.003310316824984893113, 0.003783219228554151724 ),
 .UNSPECIFIED. ) ;
#15620=CARTESIAN_POINT ( 'NONE',  ( -91.86813470756435152, 77.17527876199571324, 31.26628371047689114 ) ) ;
#15629=ORIENTED_EDGE ( 'NONE', *, *, #17226, .F. ) ;
#15635=DIRECTION ( 'NONE',  ( -0.01292414190463827932, 0.000000000000000000, -0.9999164797902018176 ) ) ;
#15642=CARTESIAN_POINT ( 'NONE',  ( -90.17429160712920577, 87.12561655205337274, 51.32195360449069454 ) ) ;
#15644=CARTESIAN_POINT ( 'NONE',  ( 79.99331838321614896, 55.00000000000000000, -1.033931352371314949 ) ) ;
#15655=CARTESIAN_POINT ( 'NONE',  ( -88.16850593027358229, 88.67837445433117693, 52.45524994280101794 ) ) ;
#15657=CARTESIAN_POINT ( 'NONE',  ( 38.69757710431291287, 94.02752048664899576, 82.47923521851859618 ) ) ;
#15662=PLANE ( 'NONE',  #2524 ) ;
#15663=SURFACE_STYLE_USAGE ( .BOTH. , #11870 ) ;
#15664=EDGE_CURVE ( 'NONE', #11011, #7441, #4668, .T. ) ;
#15665=CARTESIAN_POINT ( 'NONE',  ( 84.85446586230914079, 75.01367125662450519, 0.5443301088886967065 ) ) ;
#15667=ORIENTED_EDGE ( 'NONE', *, *, #496, .F. ) ;
#15671=CARTESIAN_POINT ( 'NONE',  ( 89.24856274066357287, 79.52628152566916242, -30.13108863562650797 ) ) ;
#15674=ORIENTED_EDGE ( 'NONE', *, *, #13685, .T. ) ;
#15676=DIRECTION ( 'NONE',  ( -0.01220060921879500583, -0.3298969072164960048, -0.9439381207174976085 ) ) ;
#15677=DIRECTION ( 'NONE',  ( 0.01292414190465215537, 0.000000000000000000, 0.9999164797902015955 ) ) ;
#15683=CARTESIAN_POINT ( 'NONE',  ( -90.04173173188732449, 70.04085162602899572, 63.25014728254400609 ) ) ;
#15685=ORIENTED_EDGE ( 'NONE', *, *, #2177, .T. ) ;
#15686=CARTESIAN_POINT ( 'NONE',  ( -91.21019055468684655, 34.61572286322119396, -28.82359390673209631 ) ) ;
#15687=CARTESIAN_POINT ( 'NONE',  ( -90.10167664437891233, 70.10962226922626428, 63.10072484710806151 ) ) ;
#15688=ADVANCED_FACE ( 'NONE', ( #7497 ), #12686, .T. ) ;
#15697=CARTESIAN_POINT ( 'NONE',  ( 90.46145803316728973, 80.27058204906826688, -32.37524683357428046 ) ) ;
#15707=B_SPLINE_CURVE_WITH_KNOTS ( 'NONE', 3,
 ( #13901, #14027, #22482, #1506 ),
 .UNSPECIFIED., .F., .F.,
 ( 4, 4 ),
 ( 0.1567379737884350976, 0.1627913398252618382 ),
 .UNSPECIFIED. ) ;
#15708=EDGE_CURVE ( 'NONE', #13344, #16500, #12137, .T. ) ;
#15709=CARTESIAN_POINT ( 'NONE',  ( -70.71197882986197669, 71.18508886668922742, -84.26048200481868378 ) ) ;
#15720=ORIENTED_EDGE ( 'NONE', *, *, #1131, .T. ) ;
#15727=VECTOR ( 'NONE', #7842, 1000.000000000000114 ) ;
#15730=DIRECTION ( 'NONE',  ( 0.009138748381789078140, -0.7071067811865487940, 0.7070477234798315802 ) ) ;
#15768=CARTESIAN_POINT ( 'NONE',  ( 90.73535795930332881, 70.47419434645436809, -62.18621042075483984 ) ) ;
#15769=CARTESIAN_POINT ( 'NONE',  ( -89.58129464662867747, 89.08235497554598226, 51.76997070739610507 ) ) ;
#15772=ORIENTED_EDGE ( 'NONE', *, *, #8901, .T. ) ;
#15776=CARTESIAN_POINT ( 'NONE',  ( -69.43142427201328815, 92.58578643762699301, 85.31868097644080251 ) ) ;
#15778=CARTESIAN_POINT ( 'NONE',  ( 82.31124572168572229, 75.11021523748625839, 3.511968633515443194 ) ) ;
#15781=ORIENTED_EDGE ( 'NONE', *, *, #18112, .F. ) ;
#15784=CARTESIAN_POINT ( 'NONE',  ( 1.421655609510571683, 55.00000000000000000, 109.9908127769221551 ) ) ;
#15785=CARTESIAN_POINT ( 'NONE',  ( -76.10506960740103466, 75.05939835648032954, 4.351290691204203753 ) ) ;
#15789=CARTESIAN_POINT ( 'NONE',  ( -37.74321565662646805, 93.98903676387503481, -82.45639044149366725 ) ) ;
#15791=CARTESIAN_POINT ( 'NONE',  ( 105.0182314695230872, 70.09775045434527385, -32.72898861654378067 ) ) ;
#15795=ORIENTED_EDGE ( 'NONE', *, *, #8937, .T. ) ;
#15796=VERTEX_POINT ( 'NONE', #1481 ) ;
#15798=VERTEX_POINT ( 'NONE', #13775 ) ;
#15803=AXIS2_PLACEMENT_3D ( 'NONE', #20282, #18240, #9840 ) ;
#15805=CARTESIAN_POINT ( 'NONE',  ( 1.364375150383346228E-14, 45.00000000000000000, -9.836439021161248541E-15 ) ) ;
#15818=SPHERICAL_SURFACE ( 'NONE', #8811, 2.000000000000000000 ) ;
#15822=CARTESIAN_POINT ( 'NONE',  ( -91.96840972750146648, 79.95771593962433599, -29.13399816620382055 ) ) ;
#15829=DIRECTION ( 'NONE',  ( 0.01292414190464131335, 1.902755938799530239E-22, 0.9999164797902015955 ) ) ;
#15832=DIRECTION ( 'NONE',  ( -0.01292414190463827932, 0.000000000000000000, -0.9999164797902018176 ) ) ;
#15834=DIRECTION ( 'NONE',  ( -2.025474946048326393E-22, 1.000000000000000000, -1.876735158486679873E-22 ) ) ;
#15849=AXIS2_PLACEMENT_3D ( 'NONE', #9462, #16497, #11313 ) ;
#15853=CARTESIAN_POINT ( 'NONE',  ( -83.58290648752343088, 104.4142135623730780, -71.51152175067954886 ) ) ;
#15856=CARTESIAN_POINT ( 'NONE',  ( -91.62437796271721879, 95.44063823554751025, -60.86849236629028326 ) ) ;
#15863=AXIS2_PLACEMENT_3D ( 'NONE', #1141, #2410, #22003 ) ;
#15867=DIRECTION ( 'NONE',  ( 0.9999164797902017066, 0.000000000000000000, -0.01292414190464174703 ) ) ;
#15870=DIRECTION ( 'NONE',  ( -2.025474946048326158E-22, 1.000000000000000000, -1.876735158486679638E-22 ) ) ;
#15871=ORIENTED_EDGE ( 'NONE', *, *, #21536, .T. ) ;
#15875=EDGE_LOOP ( 'NONE', ( #22197, #22019, #758, #20580 ) ) ;
#15878=DIRECTION ( 'NONE',  ( -0.01292414190464224663, 0.000000000000000000, -0.9999164797902015955 ) ) ;
#15884=VECTOR ( 'NONE', #3740, 1000.000000000000114 ) ;
#15885=AXIS2_PLACEMENT_3D ( 'NONE', #4714, #5683, #419 ) ;
#15888=DIRECTION ( 'NONE',  ( -0.01292414190463827932, 0.000000000000000000, -0.9999164797902018176 ) ) ;
#15889=CARTESIAN_POINT ( 'NONE',  ( -88.16677217749351314, 88.55790908203320555, 52.61947244965261916 ) ) ;
#15892=VERTEX_POINT ( 'NONE', #14742 ) ;
#15897=AXIS2_PLACEMENT_3D ( 'NONE', #17194, #13865, #1469 ) ;
#15900=ORIENTED_EDGE ( 'NONE', *, *, #1223, .F. ) ;
#15903=ORIENTED_EDGE ( 'NONE', *, *, #4152, .F. ) ;
#15907=CARTESIAN_POINT ( 'NONE',  ( -77.79076858216454582, 75.11053174630313833, -3.578068059858031447 ) ) ;
#15914=CARTESIAN_POINT ( 'NONE',  ( 105.2250167141420150, 70.47859713728952613, -32.05784361718419717 ) ) ;
#15920=ORIENTED_EDGE ( 'NONE', *, *, #13113, .F. ) ;
#15929=FACE_BOUND ( 'NONE', #20629, .T. ) ;
#15935=CARTESIAN_POINT ( 'NONE',  ( 92.25740333815001293, 79.89798572914074271, 28.97539206162133141 ) ) ;
#15937=ORIENTED_EDGE ( 'NONE', *, *, #17126, .F. ) ;
#15944=B_SPLINE_CURVE_WITH_KNOTS ( 'NONE', 3,
 ( #4418, #16749, #11445, #15986, #9735, #7328, #18457 ),
 .UNSPECIFIED., .F., .F.,
 ( 4, 3, 4 ),
 ( 0.0004832953973055784786, 0.005203611832036382848, 0.01040722366698936321 ),
 .UNSPECIFIED. ) ;
#15946=CARTESIAN_POINT ( 'NONE',  ( -93.13093775432008670, 79.82103140526460550, -28.79876782389536771 ) ) ;
#15948=B_SPLINE_CURVE_WITH_KNOTS ( 'NONE', 3,
 ( #8194, #6683, #6902, #20692, #17050, #22393, #20801, #1528, #4830, #13922, #5056, #18744, #1197, #12088, #4947, #17146, #19078, #20913 ),
 .UNSPECIFIED., .F., .F.,
 ( 4, 2, 2, 2, 2, 2, 2, 2, 4 ),
 ( 0.006298532399469907589, 0.01549750422645886604, 0.02009699013995334266, 0.02239673309670057316, 0.02469647605344780367, 0.03389544788043670487, 0.03849493379393116588, 0.04079467675067838250, 0.04309441970742561301 ),
 .UNSPECIFIED. ) ;
#15962=DIRECTION ( 'NONE',  ( -2.025474946048326158E-22, 1.000000000000000000, -1.876735158486679638E-22 ) ) ;
#15963=CARTESIAN_POINT ( 'NONE',  ( 71.61338682171094661, 92.58578643762700722, 83.49564556265194426 ) ) ;
#15965=CARTESIAN_POINT ( 'NONE',  ( -92.11140453220255608, 79.82915613195359583, 31.20677464679524604 ) ) ;
#15966=ORIENTED_EDGE ( 'NONE', *, *, #3061, .F. ) ;
#15976=VECTOR ( 'NONE', #8527, 1000.000000000000114 ) ;
#15982=CARTESIAN_POINT ( 'NONE',  ( 80.05923150692980528, 55.00000000000000000, 4.065642694558706971 ) ) ;
#15986=CARTESIAN_POINT ( 'NONE',  ( -68.61029696402175659, 89.27050837028272667, 68.20127528263711270 ) ) ;
#15989=EDGE_CURVE ( 'NONE', #15089, #959, #6834, .T. ) ;
#16002=ORIENTED_EDGE ( 'NONE', *, *, #7116, .T. ) ;
#16003=ADVANCED_FACE ( 'NONE', ( #6728 ), #17305, .T. ) ;
#16004=DIRECTION ( 'NONE',  ( 0.4654428868037414624, 0.8850574712643624053, -0.006015952371159205558 ) ) ;
#16006=CARTESIAN_POINT ( 'NONE',  ( -88.16630077365425677, 88.52135011679131082, 52.66304911287246426 ) ) ;
#16009=ORIENTED_EDGE ( 'NONE', *, *, #14709, .F. ) ;
#16010=ORIENTED_EDGE ( 'NONE', *, *, #15278, .T. ) ;
#16031=ORIENTED_EDGE ( 'NONE', *, *, #18770, .F. ) ;
#16034=EDGE_LOOP ( 'NONE', ( #4123, #13188, #10729, #7480 ) ) ;
#16041=CARTESIAN_POINT ( 'NONE',  ( -91.34835587841297411, 70.11688414259907631, 61.28278498586107759 ) ) ;
#16047=CARTESIAN_POINT ( 'NONE',  ( -88.18706637290659955, 88.71869973106718987, 50.32066939225188662 ) ) ;
#16049=CARTESIAN_POINT ( 'NONE',  ( 92.11236706770203853, 79.08401524093144985, 26.36688770261577375 ) ) ;
#16050=CARTESIAN_POINT ( 'NONE',  ( -83.95054225259529801, 104.7585062753441463, -71.08029813247938478 ) ) ;
#16060=ORIENTED_EDGE ( 'NONE', *, *, #14165, .T. ) ;
#16061=CARTESIAN_POINT ( 'NONE',  ( 41.58451242677340076, 92.58578643762696458, 83.88377541325534992 ) ) ;
#16063=FACE_OUTER_BOUND ( 'NONE', #21798, .T. ) ;
#16076=CARTESIAN_POINT ( 'NONE',  ( 90.40889375659912730, 72.00000000000000000, -33.17122784026042837 ) ) ;
#16080=CARTESIAN_POINT ( 'NONE',  ( -90.40889375659909888, 78.43035437438882695, 33.17122784026039994 ) ) ;
#16084=ORIENTED_EDGE ( 'NONE', *, *, #13617, .F. ) ;
#16090=CARTESIAN_POINT ( 'NONE',  ( 93.21002351426729149, 69.99999999999998579, 28.79774562292276840 ) ) ;
#16094=CARTESIAN_POINT ( 'NONE',  ( 88.47461587451594767, 99.92585618460377361, -65.36342861369395507 ) ) ;
#16095=CARTESIAN_POINT ( 'NONE',  ( 1.717753310876221295, 45.00000000000000000, 109.6869605904137330 ) ) ;
#16098=CARTESIAN_POINT ( 'NONE',  ( 64.05646218218323895, 104.4142135623730780, -73.41979328131711213 ) ) ;
#16101=LINE ( 'NONE', #14379, #11549 ) ;
#16108=EDGE_LOOP ( 'NONE', ( #10356, #8525, #17490, #542, #20098 ) ) ;
#16112=CARTESIAN_POINT ( 'NONE',  ( -90.04909287368641913, 87.61728352428917788, 51.02202590385057590 ) ) ;
#16114=VECTOR ( 'NONE', #14274, 1000.000000000000114 ) ;
#16117=EDGE_LOOP ( 'NONE', ( #20435, #15720, #7610, #1436 ) ) ;
#16128=EDGE_CURVE ( 'NONE', #9044, #19287, #10863, .T. ) ;
#16130=CARTESIAN_POINT ( 'NONE',  ( -79.72222561103433236, 75.13699351169601925, -4.069998570383594583 ) ) ;
#16133=CARTESIAN_POINT ( 'NONE',  ( -105.8709953322713631, 79.07548657612757381, 29.85559726770808808 ) ) ;
#16144=CARTESIAN_POINT ( 'NONE',  ( -85.09746116526416415, 74.99998524847651993, 0.7676313051536899357 ) ) ;
#16152=AXIS2_PLACEMENT_3D ( 'NONE', #8587, #15401, #5133 ) ;
#16155=FACE_OUTER_BOUND ( 'NONE', #15077, .T. ) ;
#16157=CARTESIAN_POINT ( 'NONE',  ( -64.19352405470968392, 87.93458184773491837, 62.81557474972223787 ) ) ;
#16160=CARTESIAN_POINT ( 'NONE',  ( 91.96840972750152332, 79.95771593962619761, 29.13399816620329830 ) ) ;
#16166=DIRECTION ( 'NONE',  ( 0.009138748381789112835, -0.7071067811865462405, 0.7070477234798342447 ) ) ;
#16168=AXIS2_PLACEMENT_3D ( 'NONE', #12977, #5596, #4211 ) ;
#16171=ORIENTED_EDGE ( 'NONE', *, *, #22444, .T. ) ;
#16173=CIRCLE ( 'NONE', #20903, 110.0000000000000000 ) ;
#16181=VECTOR ( 'NONE', #20245, 1000.000000000000114 ) ;
#16187=CARTESIAN_POINT ( 'NONE',  ( -91.34851551837614636, 77.30892464375351381, 31.47853330177474618 ) ) ;
#16189=CARTESIAN_POINT ( 'NONE',  ( 67.64952533873932339, 70.35418627987229456, -86.73849053056652281 ) ) ;
#16193=EDGE_CURVE ( 'NONE', #11876, #20544, #2703, .T. ) ;
#16194=CARTESIAN_POINT ( 'NONE',  ( -92.29888966083511548, 77.12912189587409273, 31.19548940143700833 ) ) ;
#16196=ORIENTED_EDGE ( 'NONE', *, *, #7978, .F. ) ;
#16211=CARTESIAN_POINT ( 'NONE',  ( -64.99457118636308905, 169.9999999999999716, 0.8400692238016759239 ) ) ;
#16232=CARTESIAN_POINT ( 'NONE',  ( -88.18408833530436652, 88.91958178016859904, 50.72524270039643568 ) ) ;
#16239=CARTESIAN_POINT ( 'NONE',  ( 41.56623493000981995, 91.17157287525387233, 82.46967996629568631 ) ) ;
#16240=CARTESIAN_POINT ( 'NONE',  ( -106.2052848363077828, 71.73256685213067385, -28.64329287727204232 ) ) ;
#16243=DIRECTION ( 'NONE',  ( 0.9999164797902017066, 2.001050586450176344E-22, -0.01292414190464270286 ) ) ;
#16244=VERTEX_POINT ( 'NONE', #6251 ) ;
#16245=DIRECTION ( 'NONE',  ( 0.9999164797902017066, 2.001050586450178931E-22, -0.01292414190464131508 ) ) ;
#16246=CARTESIAN_POINT ( 'NONE',  ( -91.23603883849614249, 78.43035437438885538, -30.82342686631250217 ) ) ;
#16247=CARTESIAN_POINT ( 'NONE',  ( -78.60505072113932101, 75.12830914639056346, 5.952647260056409984 ) ) ;
#16250=ADVANCED_FACE ( 'NONE', ( #11088 ), #14666, .F. ) ;
#16259=DIRECTION ( 'NONE',  ( -0.5121193912974635332, 0.6668151060996380108, -0.5413791123920870252 ) ) ;
#16262=CARTESIAN_POINT ( 'NONE',  ( -84.00714561647235712, 75.05057272691709613, 4.197851120138568426 ) ) ;
#16264=CARTESIAN_POINT ( 'NONE',  ( 92.46042328379809305, 77.12912189496645965, -29.19741020490909023 ) ) ;
#16269=DIRECTION ( 'NONE',  ( 2.025474946048326158E-22, -1.000000000000000000, 1.876735158486679638E-22 ) ) ;
#16279=CARTESIAN_POINT ( 'NONE',  ( 89.59156723394411870, 79.74270461908912466, 28.48704982653681483 ) ) ;
#16283=CARTESIAN_POINT ( 'NONE',  ( 1.421655609510571905, 105.0000000000000000, 109.9908127769221693 ) ) ;
#16291=CARTESIAN_POINT ( 'NONE',  ( -89.70716773419725598, 79.66972452536272442, -28.26220109401206315 ) ) ;
#16308=EDGE_CURVE ( 'NONE', #5956, #15892, #10315, .T. ) ;
#16309=CARTESIAN_POINT ( 'NONE',  ( 68.24431907518338392, 70.78648125535664803, -86.27145290589803039 ) ) ;
#16316=LINE ( 'NONE', #5591, #19792 ) ;
#16325=EDGE_CURVE ( 'NONE', #9627, #9437, #11888, .T. ) ;
#16327=CIRCLE ( 'NONE', #18494, 97.00000000000005684 ) ;
#16352=EDGE_CURVE ( 'NONE', #17835, #13946, #7657, .T. ) ;
#16365=DIRECTION ( 'NONE',  ( -0.01292414190464137060, 0.000000000000000000, -0.9999164797902015955 ) ) ;
#16376=ORIENTED_EDGE ( 'NONE', *, *, #2625, .F. ) ;
#16377=CARTESIAN_POINT ( 'NONE',  ( -81.70580161692535626, 75.12313863457445962, -3.781430161579881322 ) ) ;
#16378=CARTESIAN_POINT ( 'NONE',  ( -90.15140406382808180, 88.04290212818831662, 53.09271965600965615 ) ) ;
#16382=CARTESIAN_POINT ( 'NONE',  ( -90.51972003054838467, 79.34791451281842001, -27.24428967784130862 ) ) ;
#16388=CARTESIAN_POINT ( 'NONE',  ( 2.139116399059427742, 86.14745084375786632, -75.03391309205547088 ) ) ;
#16401=CARTESIAN_POINT ( 'NONE',  ( 75.60168123463965628, 75.03402262061140959, 1.580398487289465415 ) ) ;
#16403=DIRECTION ( 'NONE',  ( 0.01292414190463832269, 0.000000000000000000, 0.9999164797902017066 ) ) ;
#16411=CARTESIAN_POINT ( 'NONE',  ( 88.82392706003706451, 79.74373590868249551, -30.79623470077041247 ) ) ;
#16413=CARTESIAN_POINT ( 'NONE',  ( -90.41053243085599433, 78.34173690304781701, 33.04444670410828877 ) ) ;
#16414=SPHERICAL_SURFACE ( 'NONE', #4792, 2.000000000000000000 ) ;
#16431=DIRECTION ( 'NONE',  ( 0.01292414190464131335, 1.902755938799530239E-22, 0.9999164797902015955 ) ) ;
#16433=CARTESIAN_POINT ( 'NONE',  ( 81.88633517683543062, 104.6158228377113204, -73.44862222250269213 ) ) ;
#16436=CARTESIAN_POINT ( 'NONE',  ( -106.3114127004273257, 78.31407127224927933, -28.24702759725638401 ) ) ;
#16439=CARTESIAN_POINT ( 'NONE',  ( 20.71003051272330353, 88.26492295440642977, 77.04224443657528809 ) ) ;
#16440=EDGE_LOOP ( 'NONE', ( #8403, #10025 ) ) ;
#16441=ORIENTED_EDGE ( 'NONE', *, *, #8262, .F. ) ;
#16449=CARTESIAN_POINT ( 'NONE',  ( -89.50624427484768830, 89.10716308766615157, 51.66467930733914926 ) ) ;
#16459=CARTESIAN_POINT ( 'NONE',  ( -105.6473595942261028, 69.99999999999998579, -30.63715735456343126 ) ) ;
#16461=CARTESIAN_POINT ( 'NONE',  ( 68.73688910937092089, 91.46348651515937433, -85.87923151210685546 ) ) ;
#16463=FACE_OUTER_BOUND ( 'NONE', #5186, .T. ) ;
#16465=DIRECTION ( 'NONE',  ( 0.01292414190464131508, 1.902755938799530474E-22, 0.9999164797902017066 ) ) ;
#16466=CARTESIAN_POINT ( 'NONE',  ( -91.57598704441285520, 77.66227243743314546, -29.67486887243845572 ) ) ;
#16472=DIRECTION ( 'NONE',  ( -0.4768814951561130555, 0.000000000000000000, -0.8789675987075236119 ) ) ;
#16481=CARTESIAN_POINT ( 'NONE',  ( -90.11733922844207711, 88.39270497821426886, 52.83690678703658961 ) ) ;
#16493=CARTESIAN_POINT ( 'NONE',  ( 92.91045972105432327, 79.04398536109876261, 26.22408268756185734 ) ) ;
#16496=DIRECTION ( 'NONE',  ( -2.025474946048326158E-22, 1.000000000000000000, -1.876735158486679638E-22 ) ) ;
#16497=DIRECTION ( 'NONE',  ( -0.9999164797902017066, -2.001050586450177285E-22, 0.01292414190464218071 ) ) ;
#16500=VERTEX_POINT ( 'NONE', #19657 ) ;
#16507=CARTESIAN_POINT ( 'NONE',  ( 76.57033985922889485, 75.07731437015505094, -4.829186743783990821 ) ) ;
#16509=DIRECTION ( 'NONE',  ( 0.9999164797902017066, 2.001050586450178931E-22, -0.01292414190464131508 ) ) ;
#16512=EDGE_LOOP ( 'NONE', ( #15387, #10136, #2563, #7220 ) ) ;
#16513=CARTESIAN_POINT ( 'NONE',  ( 1.364374644014609697E-14, 69.99999999999998579, -9.836443712999143722E-15 ) ) ;
#16515=CARTESIAN_POINT ( 'NONE',  ( 89.38692540128420205, 98.12169273169054406, -64.10929978113784955 ) ) ;
#16519=VECTOR ( 'NONE', #3010, 1000.000000000000114 ) ;
#16520=PLANE ( 'NONE',  #20164 ) ;
#16521=LINE ( 'NONE', #19811, #19135 ) ;
#16522=DIRECTION ( 'NONE',  ( -0.01292414190464023262, 0.000000000000000000, -0.9999164797902017066 ) ) ;
#16524=ORIENTED_EDGE ( 'NONE', *, *, #3754, .T. ) ;
#16533=CARTESIAN_POINT ( 'NONE',  ( -74.16669567121724072, 95.38686586275396451, 79.68462973531357818 ) ) ;
#16549=VERTEX_POINT ( 'NONE', #17403 ) ;
#16552=CARTESIAN_POINT ( 'NONE',  ( -17.94552162158367281, 88.10632231613314502, 77.37285291568925061 ) ) ;
#16559=CARTESIAN_POINT ( 'NONE',  ( 1.364375150383346228E-14, 45.00000000000000000, -9.836439021161248541E-15 ) ) ;
#16566=CARTESIAN_POINT ( 'NONE',  ( -89.35684609684774671, 89.12360481520539679, 51.47532503655791913 ) ) ;
#16567=EDGE_CURVE ( 'NONE', #4308, #12773, #13644, .T. ) ;
#16580=CARTESIAN_POINT ( 'NONE',  ( -36.94244151028510004, 91.99797716581188922, 84.44721085690417794 ) ) ;
#16582=CARTESIAN_POINT ( 'NONE',  ( -69.72166291831146623, 97.03531796885383187, 80.87252918713471672 ) ) ;
#16596=CARTESIAN_POINT ( 'NONE',  ( -68.71681667565952978, 91.17157287525388654, 85.89527988174785378 ) ) ;
#16600=CARTESIAN_POINT ( 'NONE',  ( -84.54548942822992785, 75.02649460866172149, 3.357556456965392844 ) ) ;
#16601=CARTESIAN_POINT ( 'NONE',  ( -90.10787854355197624, 88.43547347757348120, 52.79927570075625454 ) ) ;
#16606=EDGE_CURVE ( 'NONE', #5416, #15344, #3701, .T. ) ;
#16607=CARTESIAN_POINT ( 'NONE',  ( -71.57732418163384125, 97.94802198267763060, 79.98373377021528086 ) ) ;
#16610=CARTESIAN_POINT ( 'NONE',  ( -92.90824731599330732, 79.04398536104955042, -26.22411128322386631 ) ) ;
#16612=CARTESIAN_POINT ( 'NONE',  ( 68.70320840996379275, 69.99999999999998579, 85.90686588605385055 ) ) ;
#16621=ORIENTED_EDGE ( 'NONE', *, *, #6144, .T. ) ;
#16622=AXIS2_PLACEMENT_3D ( 'NONE', #2085, #7353, #9066 ) ;
#16625=ORIENTED_EDGE ( 'NONE', *, *, #13317, .F. ) ;
#16639=VERTEX_POINT ( 'NONE', #2333 ) ;
#16642=CARTESIAN_POINT ( 'NONE',  ( 88.91001978040560516, 99.16808946942325065, -64.76993003646445857 ) ) ;
#16645=CIRCLE ( 'NONE', #5223, 3.999999999999995559 ) ;
#16646=CARTESIAN_POINT ( 'NONE',  ( 91.85126960211910330, 79.84876637418037149, -31.24149931482740783 ) ) ;
#16655=CARTESIAN_POINT ( 'NONE',  ( -63.92222308695259869, 94.02752048664899576, 83.80561885825630952 ) ) ;
#16660=CARTESIAN_POINT ( 'NONE',  ( 1.721625266288820955, 45.00000000000000000, 109.9865264768483968 ) ) ;
#16664=CARTESIAN_POINT ( 'NONE',  ( 83.82126922308901840, 105.0000000000000000, -71.23197895489381892 ) ) ;
#16665=VERTEX_POINT ( 'NONE', #7502 ) ;
#16675=CARTESIAN_POINT ( 'NONE',  ( -84.07537730384211727, 105.0000000000000000, -70.09082476868248079 ) ) ;
#16682=CARTESIAN_POINT ( 'NONE',  ( -89.07090003446140258, 88.54756155696802011, 50.44072191361355806 ) ) ;
#16686=ORIENTED_EDGE ( 'NONE', *, *, #5120, .F. ) ;
#16697=CARTESIAN_POINT ( 'NONE',  ( -38.46706438352712354, 91.17157287525387233, 85.27439087629284131 ) ) ;
#16702=CARTESIAN_POINT ( 'NONE',  ( -88.81160319069240927, 71.93448555257867838, 64.93693744786097000 ) ) ;
#16705=EDGE_CURVE ( 'NONE', #21379, #13316, #14011, .T. ) ;
#16714=CARTESIAN_POINT ( 'NONE',  ( -88.16253418885003157, 88.15973640631176522, 52.99065010345115923 ) ) ;
#16718=ADVANCED_FACE ( 'NONE', ( #11738 ), #6461, .F. ) ;
#16728=DIRECTION ( 'NONE',  ( 2.025474946048326158E-22, -1.000000000000000000, 1.876735158486679638E-22 ) ) ;
#16731=CARTESIAN_POINT ( 'NONE',  ( -68.69096839185023384, 72.00000000000000000, 87.89511284132827029 ) ) ;
#16742=CARTESIAN_POINT ( 'NONE',  ( -89.96695160930070756, 69.55454869655315520, 63.52358046848883077 ) ) ;
#16743=AXIS2_PLACEMENT_3D ( 'NONE', #8035, #18836, #2769 ) ;
#16747=CARTESIAN_POINT ( 'NONE',  ( -69.33518156588185377, 92.50622784628016859, 85.39700225480589779 ) ) ;
#16749=CARTESIAN_POINT ( 'NONE',  ( -71.30986567784941599, 88.03842148812331914, 69.24871475584893687 ) ) ;
#16751=CARTESIAN_POINT ( 'NONE',  ( 89.40066202591057731, 79.46807343418986136, -29.95041408108882308 ) ) ;
#16763=CARTESIAN_POINT ( 'NONE',  ( -109.9908127769221693, 169.9999999999999716, 1.421655609510535045 ) ) ;
#16772=CARTESIAN_POINT ( 'NONE',  ( -106.5693380255448517, 79.05027630924986681, -27.25937202119003189 ) ) ;
#16778=DIRECTION ( 'NONE',  ( -0.006350819331213228454, 0.8709385446395345731, -0.4913509118287984201 ) ) ;
#16779=CARTESIAN_POINT ( 'NONE',  ( 38.46706438352716617, 69.99999999999998579, -85.27439087629286973 ) ) ;
#16780=VERTEX_POINT ( 'NONE', #17040 ) ;
#16781=FACE_OUTER_BOUND ( 'NONE', #5132, .T. ) ;
#16787=CARTESIAN_POINT ( 'NONE',  ( 90.42246537646656179, 78.26562148642793204, -32.93420195958647412 ) ) ;
#16790=LINE ( 'NONE', #1038, #5208 ) ;
#16791=DIRECTION ( 'NONE',  ( 0.9999164797902015955, 2.001050586450176109E-22, -0.01292414190464270113 ) ) ;
#16794=CARTESIAN_POINT ( 'NONE',  ( 35.37437755136402018, 92.78536193181560066, -83.65759506009361246 ) ) ;
#16812=CARTESIAN_POINT ( 'NONE',  ( -88.16339405475061142, 88.25449051743922269, 52.91957891188045693 ) ) ;
#16815=EDGE_CURVE ( 'NONE', #984, #10132, #12840, .T. ) ;
#16816=CARTESIAN_POINT ( 'NONE',  ( 65.93268019054301021, 104.4142135623730638, 71.73965483371370055 ) ) ;
#16820=DIRECTION ( 'NONE',  ( 0.01292414190464133070, 0.000000000000000000, 0.9999164797902015955 ) ) ;
#16833=DIRECTION ( 'NONE',  ( 0.01292414190464177652, 1.902755938799532355E-22, 0.9999164797902015955 ) ) ;
#16837=ORIENTED_EDGE ( 'NONE', *, *, #18628, .T. ) ;
#16839=PLANE ( 'NONE',  #8592 ) ;
#16841=EDGE_LOOP ( 'NONE', ( #14930, #7946, #2680, #4783 ) ) ;
#16843=CARTESIAN_POINT ( 'NONE',  ( 79.59047627986713280, 75.13699351169599083, -6.129150517636113626 ) ) ;
#16844=CARTESIAN_POINT ( 'NONE',  ( -86.63143169152132828, 104.5954341936825642, -67.78689798060399596 ) ) ;
#16845=CARTESIAN_POINT ( 'NONE',  ( 105.6047345086702052, 78.54962563481561233, -30.78394349069533575 ) ) ;
#16853=CARTESIAN_POINT ( 'NONE',  ( 91.28310237474674693, 79.93543901797764306, -31.44354501024116999 ) ) ;
#16854=CARTESIAN_POINT ( 'NONE',  ( 91.21019055468687498, 34.61572286322119396, 28.82359390673205723 ) ) ;
#16855=ORIENTED_EDGE ( 'NONE', *, *, #3895, .T. ) ;
#16865=FACE_BOUND ( 'NONE', #9661, .T. ) ;
#16868=LINE ( 'NONE', #12024, #13336 ) ;
#16871=ADVANCED_FACE ( 'NONE', ( #1534 ), #15560, .T. ) ;
#16873=AXIS2_PLACEMENT_3D ( 'NONE', #22131, #2754, #6531 ) ;
#16878=CARTESIAN_POINT ( 'NONE',  ( -79.99331838321612054, 55.00000000000000000, 1.033931352371344481 ) ) ;
#16880=CYLINDRICAL_SURFACE ( 'NONE', #8491, 2.000000000000004441 ) ;
#16881=EDGE_LOOP ( 'NONE', ( #6798, #22462, #3626, #16979, #15286 ) ) ;
#16883=EDGE_LOOP ( 'NONE', ( #5848, #13605, #18651, #11118 ) ) ;
#16884=FACE_BOUND ( 'NONE', #16440, .T. ) ;
#16890=ORIENTED_EDGE ( 'NONE', *, *, #16987, .F. ) ;
#16894=CARTESIAN_POINT ( 'NONE',  ( 90.59090487622921728, 77.87375801460383684, -32.35420311765523849 ) ) ;
#16897=DIRECTION ( 'NONE',  ( -0.9999164797902015955, -2.001050586450178695E-22, 0.01292414190464131335 ) ) ;
#16898=AXIS2_PLACEMENT_3D ( 'NONE', #11083, #16728, #19781 ) ;
#16899=CARTESIAN_POINT ( 'NONE',  ( 92.82229925712802299, 72.00000000000000000, -1.199748770783335861 ) ) ;
#16910=CARTESIAN_POINT ( 'NONE',  ( -87.60134834604855314, 73.86311199051665710, 66.55747971618217207 ) ) ;
#16916=AXIS2_PLACEMENT_3D ( 'NONE', #19239, #8657, #6508 ) ;
#16922=CARTESIAN_POINT ( 'NONE',  ( -41.59208321381909457, 91.17157287525390075, -84.46951292587610283 ) ) ;
#16924=CARTESIAN_POINT ( 'NONE',  ( -88.16535734749170672, 88.44291595549381668, 52.74862968121699680 ) ) ;
#16928=ORIENTED_EDGE ( 'NONE', *, *, #2460, .T. ) ;
#16931=LINE ( 'NONE', #8193, #1543 ) ;
#16937=CARTESIAN_POINT ( 'NONE',  ( -89.22440607450261041, 80.22990097357060790, -29.93634654116231530 ) ) ;
#16940=ADVANCED_FACE ( 'NONE', ( #5955 ), #9857, .F. ) ;
#16942=CARTESIAN_POINT ( 'NONE',  ( -88.04574633781018633, 72.16093070441274904, 62.02807968949604600 ) ) ;
#16949=ADVANCED_FACE ( 'NONE', ( #13102 ), #686, .F. ) ;
#16954=EDGE_LOOP ( 'NONE', ( #356, #21759, #13037, #3683 ) ) ;
#16972=VECTOR ( 'NONE', #15328, 1000.000000000000114 ) ;
#16979=ORIENTED_EDGE ( 'NONE', *, *, #19853, .F. ) ;
#16980=CARTESIAN_POINT ( 'NONE',  ( -79.99331838321612054, 54.99999999999999289, 1.033931352371344481 ) ) ;
#16987=EDGE_CURVE ( 'NONE', #21648, #5580, #11139, .T. ) ;
#16991=EDGE_CURVE ( 'NONE', #16780, #5580, #15619, .T. ) ;
#16993=CARTESIAN_POINT ( 'NONE',  ( -70.91392079944854743, 71.82437938702648239, -84.09052168258642723 ) ) ;
#16996=DIRECTION ( 'NONE',  ( -0.01292414190464174703, 0.000000000000000000, -0.9999164797902015955 ) ) ;
#17000=DIRECTION ( 'NONE',  ( 0.9999164797902017066, -4.906538733281754926E-15, -0.01292414190464131508 ) ) ;
#17002=CARTESIAN_POINT ( 'NONE',  ( -106.2089377515398780, 77.12912189496638860, -28.62973177816246206 ) ) ;
#17004=CARTESIAN_POINT ( 'NONE',  ( 39.42082737383937996, 69.99999999999998579, -83.51645567887783272 ) ) ;
#17005=VERTEX_POINT ( 'NONE', #4776 ) ;
#17009=CIRCLE ( 'NONE', #10758, 2.000000000000004441 ) ;
#17019=ORIENTED_EDGE ( 'NONE', *, *, #8641, .T. ) ;
#17034=CARTESIAN_POINT ( 'NONE',  ( 40.65822637310714782, 91.17157287525387233, 84.25167897319538213 ) ) ;
#17035=TOROIDAL_SURFACE ( 'NONE', #4895, 0.01000000000000002623, 1.989999999999999991 ) ;
#17039=EDGE_CURVE ( 'NONE', #18312, #9274, #14039, .T. ) ;
#17040=CARTESIAN_POINT ( 'NONE',  ( -106.8724933792760652, 79.04398536104956463, -26.04362031086678897 ) ) ;
#17041=EDGE_CURVE ( 'NONE', #6883, #10450, #3799, .T. ) ;
#17045=CARTESIAN_POINT ( 'NONE',  ( -88.16567064151804800, 88.46953439568457611, 52.72066168997965718 ) ) ;
#17046=ORIENTED_EDGE ( 'NONE', *, *, #19791, .T. ) ;
#17050=CARTESIAN_POINT ( 'NONE',  ( -25.07234391868265178, 89.37624705348630982, -78.14501733294019914 ) ) ;
#17057=FACE_OUTER_BOUND ( 'NONE', #1855, .T. ) ;
#17073=FACE_OUTER_BOUND ( 'NONE', #17509, .T. ) ;
#17078=CARTESIAN_POINT ( 'NONE',  ( 105.4390993001727992, 77.44561610140188179, -31.34641640711175015 ) ) ;
#17085=CARTESIAN_POINT ( 'NONE',  ( -79.92740525950245001, 54.99999999999999289, 6.133505399301367511 ) ) ;
#17087=CARTESIAN_POINT ( 'NONE',  ( 2.067862704742617463, 72.00000000000000000, 159.9866367664322979 ) ) ;
#17088=CARTESIAN_POINT ( 'NONE',  ( -36.81271860411143848, 93.81199595286604165, -82.30577144747519469 ) ) ;
#17104=CARTESIAN_POINT ( 'NONE',  ( -64.99457118636308905, 169.9999999999999716, 0.8400692238016759239 ) ) ;
#17106=CARTESIAN_POINT ( 'NONE',  ( 70.91392079944854743, 72.00000000000000000, 84.09052168258639881 ) ) ;
#17108=LINE ( 'NONE', #8678, #6295 ) ;
#17109=DIRECTION ( 'NONE',  ( 1.490566292661454305E-14, 1.000000000000000000, -1.926591840573834312E-16 ) ) ;
#17123=ORIENTED_EDGE ( 'NONE', *, *, #8750, .T. ) ;
#17124=CARTESIAN_POINT ( 'NONE',  ( -41.61793149762837629, 69.99999999999998579, -86.46934588545651934 ) ) ;
#17126=EDGE_CURVE ( 'NONE', #14478, #3464, #16521, .T. ) ;
#17131=CARTESIAN_POINT ( 'NONE',  ( 1.163172771417732010, 45.00000000000000000, 89.99248318111813205 ) ) ;
#17134=DIRECTION ( 'NONE',  ( -0.9999164797902015955, -2.001050586450176109E-22, 0.01292414190464270113 ) ) ;
#17142=CARTESIAN_POINT ( 'NONE',  ( -90.13126742504640276, 87.37348474049055369, 51.17112193263445619 ) ) ;
#17143=ORIENTED_EDGE ( 'NONE', *, *, #5603, .F. ) ;
#17146=CARTESIAN_POINT ( 'NONE',  ( -2.523753925720915614, 86.15700740604867747, -74.98433394420648312 ) ) ;
#17150=EDGE_LOOP ( 'NONE', ( #12543, #11998, #5478, #13770, #8611, #6059 ) ) ;
#17152=EDGE_LOOP ( 'NONE', ( #8328, #5462, #18117, #13634 ) ) ;
#17156=CARTESIAN_POINT ( 'NONE',  ( 90.43417961988760112, 79.20545292891344502, -29.12427242046056008 ) ) ;
#17164=ORIENTED_EDGE ( 'NONE', *, *, #396, .F. ) ;
#17165=AXIS2_PLACEMENT_3D ( 'NONE', #17131, #15203, #13467 ) ;
#17172=CIRCLE ( 'NONE', #22271, 2.000000000000001776 ) ;
#17174=CARTESIAN_POINT ( 'NONE',  ( -93.17671387018313567, 79.04398536104955042, -26.22064129356660800 ) ) ;
#17177=VERTEX_POINT ( 'NONE', #22179 ) ;
#17185=DIRECTION ( 'NONE',  ( 0.9999164797902017066, 2.001050586450178931E-22, -0.01292414190464131508 ) ) ;
#17188=LINE ( 'NONE', #11922, #3949 ) ;
#17191=CARTESIAN_POINT ( 'NONE',  ( -70.91392079944854743, 72.00000000000000000, -84.09052168258642723 ) ) ;
#17194=CARTESIAN_POINT ( 'NONE',  ( -63.91983116576977153, 91.51644034066822542, 67.07156771589210109 ) ) ;
#17199=EDGE_CURVE ( 'NONE', #7316, #7202, #22438, .T. ) ;
#17204=AXIS2_PLACEMENT_3D ( 'NONE', #3931, #16269, #736 ) ;
#17211=ADVANCED_FACE ( 'NONE', ( #4074 ), #20459, .F. ) ;
#17216=CARTESIAN_POINT ( 'NONE',  ( -109.6289368035922536, 77.12912189496637438, 29.41931704363613420 ) ) ;
#17226=EDGE_CURVE ( 'NONE', #984, #17835, #4836, .T. ) ;
#17227=EDGE_LOOP ( 'NONE', ( #11553, #15795, #18230 ) ) ;
#17239=AXIS2_PLACEMENT_3D ( 'NONE', #2062, #7225, #17706 ) ;
#17242=PLANE ( 'NONE',  #12979 ) ;
#17251=CARTESIAN_POINT ( 'NONE',  ( -90.05921627452258349, 88.59350953919012284, 52.64378069695336393 ) ) ;
#17255=AXIS2_PLACEMENT_3D ( 'NONE', #3018, #4840, #11877 ) ;
#17256=ORIENTED_EDGE ( 'NONE', *, *, #11170, .F. ) ;
#17259=CARTESIAN_POINT ( 'NONE',  ( 88.82263333796723259, 169.9999999999999716, -1.148052203164690033 ) ) ;
#17261=CARTESIAN_POINT ( 'NONE',  ( 81.08638132281690503, 75.13007332810629180, -6.018189424661123610 ) ) ;
#17291=CARTESIAN_POINT ( 'NONE',  ( -88.09114847236423884, 72.29207065074294292, 61.95466991546196311 ) ) ;
#17296=CARTESIAN_POINT ( 'NONE',  ( 66.18268079339601684, 69.99999999999998579, -87.86269266872859873 ) ) ;
#17302=DIRECTION ( 'NONE',  ( 2.025474946048326158E-22, -1.000000000000000000, 1.876735158486679638E-22 ) ) ;
#17305=PLANE ( 'NONE',  #17661 ) ;
#17307=CARTESIAN_POINT ( 'NONE',  ( 1.163172771417732010, 69.99999999999998579, 89.99248318111813205 ) ) ;
#17311=AXIS2_PLACEMENT_3D ( 'NONE', #19046, #9997, #20662 ) ;
#17324=AXIS2_PLACEMENT_3D ( 'NONE', #17919, #2154, #11128 ) ;
#17325=AXIS2_PLACEMENT_3D ( 'NONE', #16878, #6305, #20069 ) ;
#17327=CARTESIAN_POINT ( 'NONE',  ( -65.90110554552374822, 105.0000000000000000, -69.29678410920486442 ) ) ;
#17331=CARTESIAN_POINT ( 'NONE',  ( 38.69757710431291287, 94.02752048664899576, 82.47923521851859618 ) ) ;
#17332=CARTESIAN_POINT ( 'NONE',  ( -92.43457499998879712, 77.12912189496637438, 31.19724316448926160 ) ) ;
#17350=CIRCLE ( 'NONE', #7436, 2.000000000000001776 ) ;
#17355=EDGE_CURVE ( 'NONE', #5608, #10157, #13923, .T. ) ;
#17359=CARTESIAN_POINT ( 'NONE',  ( 106.8724933792760226, 79.04398536104964990, 26.04362031086705542 ) ) ;
#17366=ORIENTED_EDGE ( 'NONE', *, *, #2625, .T. ) ;
#17368=VERTEX_POINT ( 'NONE', #15776 ) ;
#17370=DIRECTION ( 'NONE',  ( 2.025474946048326158E-22, -1.000000000000000000, 1.876735158486679638E-22 ) ) ;
#17371=CARTESIAN_POINT ( 'NONE',  ( -90.15853200097006948, 87.23282554233360031, 51.25677079265641112 ) ) ;
#17374=CARTESIAN_POINT ( 'NONE',  ( 1.117803423002105445, 55.00000000000000000, 109.6947150755565161 ) ) ;
#17376=MANIFOLD_SOLID_BREP ( 'Stock-MAS-425-1', #13198 ) ;
#17378=EDGE_LOOP ( 'NONE', ( #7118, #12653, #21322, #5028 ) ) ;
#17383=LINE ( 'NONE', #1638, #15009 ) ;
#17394=CARTESIAN_POINT ( 'NONE',  ( -90.01466456474447853, 70.04421420112709029, 63.22468240810439966 ) ) ;
#17397=EDGE_LOOP ( 'NONE', ( #5758, #19430, #732 ) ) ;
#17401=CARTESIAN_POINT ( 'NONE',  ( 105.3709006619169912, 71.09718787230102066, -31.57492962159256322 ) ) ;
#17403=CARTESIAN_POINT ( 'NONE',  ( -105.6473595942261028, 69.99999999999998579, -30.63715735456343126 ) ) ;
#17406=ORIENTED_EDGE ( 'NONE', *, *, #12907, .T. ) ;
#17408=AXIS2_PLACEMENT_3D ( 'NONE', #20781, #14255, #6773 ) ;
#17414=CIRCLE ( 'NONE', #14100, 2.000000000000004885 ) ;
#17425=VECTOR ( 'NONE', #18587, 1000.000000000000114 ) ;
#17433=CARTESIAN_POINT ( 'NONE',  ( -68.43148148480358373, 69.99999999999998579, -86.12277481476654373 ) ) ;
#17445=ORIENTED_EDGE ( 'NONE', *, *, #5465, .F. ) ;
#17450=DIRECTION ( 'NONE',  ( 0.009985269297354652795, 0.6348858185549770550, 0.7725414498878595548 ) ) ;
#17453=DIRECTION ( 'NONE',  ( -0.01292414190464174703, 0.000000000000000000, -0.9999164797902015955 ) ) ;
#17462=CARTESIAN_POINT ( 'NONE',  ( 39.99341017485146921, 93.41702043937449673, 83.07303732978165556 ) ) ;
#17468=ORIENTED_EDGE ( 'NONE', *, *, #3304, .F. ) ;
#17474=CARTESIAN_POINT ( 'NONE',  ( -89.91407985229524513, 87.87209748402599985, 50.86527297701809402 ) ) ;
#17487=CARTESIAN_POINT ( 'NONE',  ( -89.55253866421617204, 89.09534416471163354, 51.72748700526515364 ) ) ;
#17490=ORIENTED_EDGE ( 'NONE', *, *, #9376, .T. ) ;
#17500=DIRECTION ( 'NONE',  ( -2.025474946048326158E-22, 1.000000000000000000, -1.876735158486679638E-22 ) ) ;
#17501=CARTESIAN_POINT ( 'NONE',  ( -75.17629230947522956, 75.01375443481772720, -0.6738748282868175510 ) ) ;
#17503=ADVANCED_FACE ( 'NONE', ( #8107 ), #20489, .F. ) ;
#17507=CARTESIAN_POINT ( 'NONE',  ( -38.21725235583850377, 94.02752048664900997, -82.48544352224706699 ) ) ;
#17509=EDGE_LOOP ( 'NONE', ( #17046, #19975, #12633, #807 ) ) ;
#17510=ORIENTED_EDGE ( 'NONE', *, *, #4314, .T. ) ;
#17511=( BOUNDED_SURFACE ( )  B_SPLINE_SURFACE ( 3, 2, ( 
 ( #7737, #19774, #393 ),
 ( #4273, #862, #740 ),
 ( #21831, #11075, #14774 ),
 ( #11297, #624, #9577 ) ),
 .UNSPECIFIED., .F., .F., .T. ) 
 B_SPLINE_SURFACE_WITH_KNOTS ( ( 4, 4 ),
 ( 3, 3 ),
 ( 0.4226013619543069755, 0.4841788640348455575 ),
 ( 0.000000000000000000, 1.000000000000000000 ),
 .UNSPECIFIED. ) 
 GEOMETRIC_REPRESENTATION_ITEM ( )  RATIONAL_B_SPLINE_SURFACE ( (
 ( 1.000000000000000000, 0.9068900557993654354, 1.000000000000000000),
 ( 1.000000000000000000, 0.9052491015987682577, 1.000000000000000000),
 ( 1.000000000000000000, 0.9034913259101550187, 1.000000000000000000),
 ( 1.000000000000000000, 0.9016180287879269617, 1.000000000000000000) ) ) 
 REPRESENTATION_ITEM ( '' )  SURFACE ( )  );
#17512=DIRECTION ( 'NONE',  ( -0.9999164797902015955, -6.938893903907235477E-15, 0.01292414190464525985 ) ) ;
#17515=VERTEX_POINT ( 'NONE', #17296 ) ;
#17522=CARTESIAN_POINT ( 'NONE',  ( -90.92043330041786930, 70.33842041176643534, 61.91522761515599882 ) ) ;
#17523=DIRECTION ( 'NONE',  ( -0.9999164797902017066, -2.001050586450178931E-22, 0.01292414190464131508 ) ) ;
#17525=DIRECTION ( 'NONE',  ( -0.01292414190464137060, 0.000000000000000000, -0.9999164797902015955 ) ) ;
#17528=CARTESIAN_POINT ( 'NONE',  ( 91.24493283426487267, 78.25381457448439448, 30.56897831620030459 ) ) ;
#17530=EDGE_CURVE ( 'NONE', #7441, #2301, #6249, .T. ) ;
#17531=CARTESIAN_POINT ( 'NONE',  ( 89.24601225622841127, 80.14389198580501272, 29.68648583522423934 ) ) ;
#17537=VERTEX_POINT ( 'NONE', #21283 ) ;
#17538=CARTESIAN_POINT ( 'NONE',  ( -91.85896106039054132, 79.10764833873336954, -26.44817522613631411 ) ) ;
#17541=CARTESIAN_POINT ( 'NONE',  ( -68.70320840996376432, 69.99999999999998579, -85.90686588605387897 ) ) ;
#17546=FACE_OUTER_BOUND ( 'NONE', #9331, .T. ) ;
#17551=ORIENTED_EDGE ( 'NONE', *, *, #7404, .T. ) ;
#17554=ADVANCED_FACE ( 'NONE', ( #22634 ), #19965, .F. ) ;
#17560=FACE_OUTER_BOUND ( 'NONE', #21069, .T. ) ;
#17561=CARTESIAN_POINT ( 'NONE',  ( -90.46801631146684031, 78.10499069285114615, 32.69910015975905537 ) ) ;
#17585=CARTESIAN_POINT ( 'NONE',  ( -89.40156491642460423, 88.37278921414913668, 50.55266491976622945 ) ) ;
#17587=CARTESIAN_POINT ( 'NONE',  ( 106.3651776870870691, 78.54983655346507021, 28.04389441634570446 ) ) ;
#17588=CARTESIAN_POINT ( 'NONE',  ( -90.17351897532782345, 87.00751446224754204, 51.38173066951565460 ) ) ;
#17597=EDGE_LOOP ( 'NONE', ( #11355, #14849, #17752, #755 ) ) ;
#17600=CARTESIAN_POINT ( 'NONE',  ( -89.87306261084498260, 88.90191489356698185, 52.23091996317439367 ) ) ;
#17603=CARTESIAN_POINT ( 'NONE',  ( -92.46788464407291031, 79.04398536104955042, 28.62013883513304080 ) ) ;
#17604=CARTESIAN_POINT ( 'NONE',  ( -34.68008326079426951, 93.81386119346835528, 83.23154952960750563 ) ) ;
#17607=CARTESIAN_POINT ( 'NONE',  ( -91.21019055468684655, 77.12912189496638860, -28.82359390673209631 ) ) ;
#17611=CARTESIAN_POINT ( 'NONE',  ( -1.247179693797872524, 69.99999999999998579, -96.49194029975447506 ) ) ;
#17613=CARTESIAN_POINT ( 'NONE',  ( 1.717753310876221295, 45.00000000000000000, 109.6869605904137330 ) ) ;
#17614=CARTESIAN_POINT ( 'NONE',  ( -77.24079330402096843, 75.09876982897525011, 5.330581268580301568 ) ) ;
#17616=CARTESIAN_POINT ( 'NONE',  ( -105.4334892372614121, 77.12912189496637438, 31.36525700924958926 ) ) ;
#17623=AXIS2_PLACEMENT_3D ( 'NONE', #17104, #20749, #1366 ) ;
#17625=EDGE_CURVE ( 'NONE', #3455, #17005, #11197, .T. ) ;
#17627=APPLICATION_CONTEXT ( 'automotive_design' ) ;
#17650=( BOUNDED_CURVE ( )  B_SPLINE_CURVE ( 3, ( #2278, #21653, #9277, #12634 ),
 .UNSPECIFIED., .F., .T. ) 
 B_SPLINE_CURVE_WITH_KNOTS ( ( 4, 4 ),
 ( 5.433035758877963417, 5.587168164874065646 ),
 .UNSPECIFIED. ) 
 CURVE ( )  GEOMETRIC_REPRESENTATION_ITEM ( )  RATIONAL_B_SPLINE_CURVE ( ( 1.000000000000000000, 0.9980212464270939998, 0.9980212464270939998, 1.000000000000000000 ) ) 
 REPRESENTATION_ITEM ( '' )  );
#17654=AXIS2_PLACEMENT_3D ( 'NONE', #1351, #22320, #3264 ) ;
#17657=CARTESIAN_POINT ( 'NONE',  ( -91.52774025374972666, 80.10656073859030357, -29.55378794065120474 ) ) ;
#17661=AXIS2_PLACEMENT_3D ( 'NONE', #19119, #14325, #19352 ) ;
#17671=VERTEX_POINT ( 'NONE', #626 ) ;
#17674=DIRECTION ( 'NONE',  ( 0.9999164797902017066, 2.001050586450178931E-22, -0.01292414190464131508 ) ) ;
#17675=CARTESIAN_POINT ( 'NONE',  ( -39.42082737383935154, 72.00000000000000000, 83.51645567887779009 ) ) ;
#17677=CARTESIAN_POINT ( 'NONE',  ( 2.067862704742617463, 72.00000000000000000, 159.9866367664322979 ) ) ;
#17680=DIRECTION ( 'NONE',  ( -0.01292414190464137060, 8.764918615461757854E-16, -0.9999164797902015955 ) ) ;
#17684=VECTOR ( 'NONE', #16259, 999.9999999999998863 ) ;
#17706=DIRECTION ( 'NONE',  ( 0.01292414190464177652, 1.902755938799532355E-22, 0.9999164797902015955 ) ) ;
#17708=ORIENTED_EDGE ( 'NONE', *, *, #11636, .F. ) ;
#17711=PLANE ( 'NONE',  #5564 ) ;
#17712=ORIENTED_EDGE ( 'NONE', *, *, #15505, .F. ) ;
#17713=ADVANCED_FACE ( 'NONE', ( #19900 ), #4170, .F. ) ;
#17720=ORIENTED_EDGE ( 'NONE', *, *, #10468, .F. ) ;
#17721=CARTESIAN_POINT ( 'NONE',  ( 90.45626474936497630, 70.75678324216411852, -62.59145595768703174 ) ) ;
#17722=CARTESIAN_POINT ( 'NONE',  ( -89.69275295551862826, 89.03869477057148174, 51.93053011967995758 ) ) ;
#17724=ORIENTED_EDGE ( 'NONE', *, *, #3050, .F. ) ;
#17726=ORIENTED_EDGE ( 'NONE', *, *, #6704, .T. ) ;
#17731=CARTESIAN_POINT ( 'NONE',  ( 80.72971245143067165, 75.13518351147561702, 4.023615192978592603 ) ) ;
#17733=LINE ( 'NONE', #253, #16114 ) ;
#17737=B_SPLINE_CURVE_WITH_KNOTS ( 'NONE', 3,
 ( #20943, #21173, #5204, #12238, #15065, #20200, #6440, #21797, #20424, #4678, #16894, #7925, #18600, #16787, #13114, #22023 ),
 .UNSPECIFIED., .F., .F.,
 ( 4, 2, 2, 2, 2, 2, 2, 4 ),
 ( 0.000000000000000000, 0.0004291333152394394778, 0.0008582666304788767872, 0.001716533260957743600, 0.002145666576197192889, 0.002574799891436641529, 0.003003933206676090602, 0.003433066521915540108 ),
 .UNSPECIFIED. ) ;
#17746=DIRECTION ( 'NONE',  ( -0.9999164797902017066, -2.001050586450178931E-22, 0.01292414190464131508 ) ) ;
#17747=ADVANCED_FACE ( 'NONE', ( #17057 ), #2211, .T. ) ;
#17750=EDGE_CURVE ( 'NONE', #12076, #21601, #14992, .T. ) ;
#17752=ORIENTED_EDGE ( 'NONE', *, *, #11482, .T. ) ;
#17760=ORIENTED_EDGE ( 'NONE', *, *, #10761, .T. ) ;
#17761=FACE_OUTER_BOUND ( 'NONE', #3590, .T. ) ;
#17763=CARTESIAN_POINT ( 'NONE',  ( -88.05170339851980543, 72.97786998644572520, 61.56719313945616534 ) ) ;
#17771=FACE_OUTER_BOUND ( 'NONE', #778, .T. ) ;
#17773=CARTESIAN_POINT ( 'NONE',  ( 91.14933227754937661, 79.20679280668171884, 26.78161688013026165 ) ) ;
#17774=EDGE_CURVE ( 'NONE', #21224, #567, #15231, .T. ) ;
#17775=DIRECTION ( 'NONE',  ( -0.9999164797902015955, 0.000000000000000000, 0.01292414190464174703 ) ) ;
#17780=CARTESIAN_POINT ( 'NONE',  ( -91.41775219751524162, 77.84255103198131565, -29.95431514105994353 ) ) ;
#17785=CARTESIAN_POINT ( 'NONE',  ( -69.49687660543771983, 70.17287388826144934, -85.26604680535984926 ) ) ;
#17790=FACE_OUTER_BOUND ( 'NONE', #15462, .T. ) ;
#17791=ORIENTED_EDGE ( 'NONE', *, *, #16987, .T. ) ;
#17794=EDGE_LOOP ( 'NONE', ( #2193, #19397, #3624, #10998, #18904, #13168, #1851, #16928, #8167, #10564 ) ) ;
#17797=DIRECTION ( 'NONE',  ( 0.9999164797902015955, 2.001050586450178695E-22, -0.01292414190464131335 ) ) ;
#17798=CARTESIAN_POINT ( 'NONE',  ( 66.18268079339601684, 69.99999999999998579, -87.86269266872859873 ) ) ;
#17800=CARTESIAN_POINT ( 'NONE',  ( -88.44788333809836445, 80.14655074237849419, 31.99095626761631195 ) ) ;
#17809=CARTESIAN_POINT ( 'NONE',  ( -39.75021781620441885, 72.00000000000000000, -86.03367798009510636 ) ) ;
#17819=DIRECTION ( 'NONE',  ( 0.9999164797902017066, 4.653667080246435885E-16, -0.01292414190464085018 ) ) ;
#17826=CARTESIAN_POINT ( 'NONE',  ( 41.56623493000984126, 69.99999999999998579, 82.46967996629570052 ) ) ;
#17832=FACE_OUTER_BOUND ( 'NONE', #1096, .T. ) ;
#17833=ADVANCED_FACE ( 'NONE', ( #6578 ), #4722, .F. ) ;
#17835=VERTEX_POINT ( 'NONE', #1425 ) ;
#17841=CARTESIAN_POINT ( 'NONE',  ( -89.92684002299503732, 87.84535921386273571, 50.88169406451069676 ) ) ;
#17843=CIRCLE ( 'NONE', #4228, 2.000000000000004441 ) ;
#17846=EDGE_CURVE ( 'NONE', #7720, #19552, #21993, .T. ) ;
#17849=DIRECTION ( 'NONE',  ( -2.025474946048326158E-22, 1.000000000000000000, -1.876735158486678933E-22 ) ) ;
#17851=CARTESIAN_POINT ( 'NONE',  ( -105.6848962833589383, 69.99999999999998579, -30.50771805806158454 ) ) ;
#17852=LINE ( 'NONE', #8969, #7094 ) ;
#17854=CARTESIAN_POINT ( 'NONE',  ( 91.44886093103751534, 77.80125034018027463, 29.89077835665231930 ) ) ;
#17860=CARTESIAN_POINT ( 'NONE',  ( -105.9973908263409328, 79.15210294646404066, 29.40494008559752714 ) ) ;
#17866=CARTESIAN_POINT ( 'NONE',  ( -37.54386652542168434, 92.77591188308413450, -82.72434418715882032 ) ) ;
#17867=VERTEX_POINT ( 'NONE', #971 ) ;
#17878=CARTESIAN_POINT ( 'NONE',  ( -91.38403781951991789, 79.16811561863683266, -26.65243986599113768 ) ) ;
#17880=VECTOR ( 'NONE', #10224, 1000.000000000000000 ) ;
#17881=CARTESIAN_POINT ( 'NONE',  ( -64.10659645996310019, 93.47724784606892001, 69.54099877995811596 ) ) ;
#17884=CARTESIAN_POINT ( 'NONE',  ( 91.32446103601381537, 78.00118640252709667, 30.19495016275310917 ) ) ;
#17885=CARTESIAN_POINT ( 'NONE',  ( 92.11907261954644355, 79.08352528315391794, 26.36518256425470241 ) ) ;
#17887=DIRECTION ( 'NONE',  ( 2.025474946048326158E-22, -1.000000000000000000, 1.876735158486679638E-22 ) ) ;
#17896=CARTESIAN_POINT ( 'NONE',  ( -110.8973471360828285, 103.0000000000000000, -68.71519772349600430 ) ) ;
#17897=CYLINDRICAL_SURFACE ( 'NONE', #14820, 6.499999999999998224 ) ;
#17898=ORIENTED_EDGE ( 'NONE', *, *, #15011, .T. ) ;
#17906=CARTESIAN_POINT ( 'NONE',  ( -88.82392706003518867, 79.74373590868249551, 30.79623470077038050 ) ) ;
#17910=B_SPLINE_CURVE_WITH_KNOTS ( 'NONE', 3,
 ( #16246, #9321, #836, #7595, #4360, #16466, #14752, #11277, #18074, #14631, #17959, #10936, #11386, #3915, #9551, #371 ),
 .UNSPECIFIED., .F., .F.,
 ( 4, 2, 2, 2, 2, 2, 2, 4 ),
 ( 0.000000000000000000, 0.0008607555596716879491, 0.001291133339507522654, 0.001721511119343357467, 0.002151888899179192280, 0.002582266679015027093, 0.003012644458850861906, 0.003443022238686696719 ),
 .UNSPECIFIED. ) ;
#17912=FACE_OUTER_BOUND ( 'NONE', #10120, .T. ) ;
#17913=DIRECTION ( 'NONE',  ( 0.4540042784513456109, 0.000000000000000000, -0.8909995034498464639 ) ) ;
#17919=CARTESIAN_POINT ( 'NONE',  ( 1.117803423002105445, 55.00000000000000000, 109.6947150755565161 ) ) ;
#17920=AXIS2_PLACEMENT_3D ( 'NONE', #11641, #10031, #18637 ) ;
#17922=CARTESIAN_POINT ( 'NONE',  ( -35.37437755136378570, 92.78536193180231351, 83.65759506009349877 ) ) ;
#17926=ORIENTED_EDGE ( 'NONE', *, *, #3883, .T. ) ;
#17941=CARTESIAN_POINT ( 'NONE',  ( -90.09632239900712136, 87.49413173051891590, 51.09744761898891596 ) ) ;
#17957=ORIENTED_EDGE ( 'NONE', *, *, #12368, .F. ) ;
#17959=CARTESIAN_POINT ( 'NONE',  ( -92.25563491934029514, 77.27426140725017945, -29.04871113840125219 ) ) ;
#17960=CARTESIAN_POINT ( 'NONE',  ( -78.25644772108614688, 75.12006735377332234, -3.764112139945209989 ) ) ;
#17963=DIRECTION ( 'NONE',  ( 0.01125613334114018010, 0.4913919529878011949, 0.8708658036695671179 ) ) ;
#17972=EDGE_LOOP ( 'NONE', ( #7637, #21669, #4364, #18437, #8606 ) ) ;
#17973=CARTESIAN_POINT ( 'NONE',  ( 86.79222083800954124, 104.3814432989690602, 67.58039954014910222 ) ) ;
#17988=CARTESIAN_POINT ( 'NONE',  ( 89.98285967923904138, 79.53265832318567163, 27.83436926225109431 ) ) ;
#17989=CARTESIAN_POINT ( 'NONE',  ( 90.71810225913510806, 79.29666913609152346, 27.07744225877261712 ) ) ;
#17990=CIRCLE ( 'NONE', #750, 3.999999999999995559 ) ;
#17997=CARTESIAN_POINT ( 'NONE',  ( -92.80269534486276939, 79.83421200779902449, -28.82571798309893651 ) ) ;
#18004=AXIS2_PLACEMENT_3D ( 'NONE', #3261, #17302, #1562 ) ;
#18009=ORIENTED_EDGE ( 'NONE', *, *, #20695, .T. ) ;
#18014=DIRECTION ( 'NONE',  ( 0.01292414190464174703, 0.000000000000000000, 0.9999164797902015955 ) ) ;
#18016=CARTESIAN_POINT ( 'NONE',  ( -89.40066202591053468, 79.46807343419025926, 29.95041408109006653 ) ) ;
#18019=CARTESIAN_POINT ( 'NONE',  ( -39.39497909003006981, 72.00000000000000000, 85.51628863845817818 ) ) ;
#18022=CARTESIAN_POINT ( 'NONE',  ( -90.41042953090172318, 78.34730160488616946, 33.05240787946384984 ) ) ;
#18024=VERTEX_POINT ( 'NONE', #8379 ) ;
#18028=CARTESIAN_POINT ( 'NONE',  ( 105.4334892372614405, 77.12912189496645965, -31.36525700924962834 ) ) ;
#18030=ORIENTED_EDGE ( 'NONE', *, *, #11755, .F. ) ;
#18036=EDGE_LOOP ( 'NONE', ( #15781, #16441, #4781, #5573, #3697 ) ) ;
#18038=VECTOR ( 'NONE', #17887, 1000.000000000000000 ) ;
#18041=ORIENTED_EDGE ( 'NONE', *, *, #8691, .F. ) ;
#18053=CIRCLE ( 'NONE', #15500, 2.000000000000002665 ) ;
#18056=CARTESIAN_POINT ( 'NONE',  ( -88.18034797016093762, 89.00358945086300366, 51.18297751363882497 ) ) ;
#18060=ORIENTED_EDGE ( 'NONE', *, *, #13973, .T. ) ;
#18063=ORIENTED_EDGE ( 'NONE', *, *, #18757, .F. ) ;
#18067=CARTESIAN_POINT ( 'NONE',  ( 65.91440269377942229, 103.0000000000000000, 70.32555938675403695 ) ) ;
#18068=CARTESIAN_POINT ( 'NONE',  ( 396.9612392269590373, 103.0000000000000000, 66.04670572356099001 ) ) ;
#18071=CARTESIAN_POINT ( 'NONE',  ( 92.25563491934033777, 77.27426140725016523, 29.04871113840120600 ) ) ;
#18074=CARTESIAN_POINT ( 'NONE',  ( -91.92156639752093383, 77.41735670888594711, -29.28407961425102002 ) ) ;
#18084=EDGE_CURVE ( 'NONE', #12773, #20154, #1066, .T. ) ;
#18087=EDGE_CURVE ( 'NONE', #21893, #6852, #14010, .T. ) ;
#18091=CARTESIAN_POINT ( 'NONE',  ( -83.88046665555830828, 75.05943625219151727, -2.284324781586978048 ) ) ;
#18092=CARTESIAN_POINT ( 'NONE',  ( -90.14880203183271590, 88.11115007023326484, 53.04766197139571204 ) ) ;
#18101=ADVANCED_FACE ( 'NONE', ( #17832 ), #6881, .F. ) ;
#18106=CARTESIAN_POINT ( 'NONE',  ( 93.05058556066120445, 79.82257531472971834, 28.80218916741394253 ) ) ;
#18112=EDGE_CURVE ( 'NONE', #9516, #11382, #18772, .T. ) ;
#18114=CARTESIAN_POINT ( 'NONE',  ( -1.124400345703781001, 72.00000000000000000, -86.99273374174757123 ) ) ;
#18115=ORIENTED_EDGE ( 'NONE', *, *, #5912, .F. ) ;
#18117=ORIENTED_EDGE ( 'NONE', *, *, #3480, .F. ) ;
#18118=DIRECTION ( 'NONE',  ( 0.006350819331213225852, -0.8709385446395345731, 0.4913509118287982536 ) ) ;
#18121=CARTESIAN_POINT ( 'NONE',  ( 78.73611885933964061, 75.12836414114961769, 3.920034999058580105 ) ) ;
#18122=CARTESIAN_POINT ( 'NONE',  ( -90.73089019026657809, 70.47975153197518239, 61.57984177518897440 ) ) ;
#18134=CARTESIAN_POINT ( 'NONE',  ( 92.27487665213190837, 79.82259189700671698, -31.19759217298441811 ) ) ;
#18136=CARTESIAN_POINT ( 'NONE',  ( -90.99469209931201874, 80.00980328568596178, 31.64094806796596160 ) ) ;
#18148=CARTESIAN_POINT ( 'NONE',  ( -75.30975508861040169, 94.90914755154933857, 80.17755788556743823 ) ) ;
#18154=EDGE_CURVE ( 'NONE', #12564, #3568, #18053, .T. ) ;
#18155=ORIENTED_EDGE ( 'NONE', *, *, #13853, .T. ) ;
#18159=CARTESIAN_POINT ( 'NONE',  ( -106.3959516824314022, 78.65697569891366925, -27.92701496092233882 ) ) ;
#18162=CARTESIAN_POINT ( 'NONE',  ( -11.26897896307171720, 86.89782342943594529, 75.98389258083668096 ) ) ;
#18170=CARTESIAN_POINT ( 'NONE',  ( -88.17241286529819888, 88.87836946248037862, 52.06316210395358723 ) ) ;
#18182=CYLINDRICAL_SURFACE ( 'NONE', #5472, 2.000000000000001332 ) ;
#18183=ORIENTED_EDGE ( 'NONE', *, *, #22047, .T. ) ;
#18184=LINE ( 'NONE', #14280, #18721 ) ;
#18188=CARTESIAN_POINT ( 'NONE',  ( -41.56623493000981284, 91.17157287525390075, -82.46967996629571473 ) ) ;
#18199=CARTESIAN_POINT ( 'NONE',  ( -85.05069750351505320, 75.00181558815789629, 1.771077756321887797 ) ) ;
#18200=CARTESIAN_POINT ( 'NONE',  ( -88.16296040167131309, 88.20774758960868667, 52.95573524961071143 ) ) ;
#18207=CARTESIAN_POINT ( 'NONE',  ( -72.50839346369934901, 87.61416393227378308, 70.38952438936911449 ) ) ;
#18217=DIRECTION ( 'NONE',  ( 0.9999164797902017066, 2.001050586450180576E-22, -0.01292414190464044946 ) ) ;
#18222=ADVANCED_FACE ( 'NONE', ( #5268 ), #17711, .F. ) ;
#18224=CARTESIAN_POINT ( 'NONE',  ( 74.88917560116811956, 74.99998524847650572, -1.300231399588960723 ) ) ;
#18230=ORIENTED_EDGE ( 'NONE', *, *, #4136, .T. ) ;
#18231=CARTESIAN_POINT ( 'NONE',  ( -68.71681667565952978, 91.17157287525388654, 85.89527988174785378 ) ) ;
#18236=DIRECTION ( 'NONE',  ( 0.9999164797902015955, 2.001050586450180341E-22, -0.01292414190464038874 ) ) ;
#18240=DIRECTION ( 'NONE',  ( 0.9999164797902017066, 2.001050586450178931E-22, -0.01292414190464131508 ) ) ;
#18247=EDGE_CURVE ( 'NONE', #12598, #12496, #7462, .T. ) ;
#18250=EDGE_CURVE ( 'NONE', #11360, #14478, #2294, .T. ) ;
#18253=CARTESIAN_POINT ( 'NONE',  ( 82.72602501251986951, 105.0000000000000142, -72.50183911544655757 ) ) ;
#18255=ORIENTED_EDGE ( 'NONE', *, *, #11799, .T. ) ;
#18261=LINE ( 'NONE', #12863, #11451 ) ;
#18266=EDGE_CURVE ( 'NONE', #10332, #784, #18261, .T. ) ;
#18270=CARTESIAN_POINT ( 'NONE',  ( -89.37197774827599517, 89.12559863199479082, 51.49225512938619431 ) ) ;
#18276=ORIENTED_EDGE ( 'NONE', *, *, #3583, .T. ) ;
#18284=CARTESIAN_POINT ( 'NONE',  ( -71.36098783483133445, 96.34992515573605942, 81.57916788671384722 ) ) ;
#18289=CARTESIAN_POINT ( 'NONE',  ( -0.9951589266573748205, 69.99999999999998579, -76.99356894384553129 ) ) ;
#18292=VECTOR ( 'NONE', #7753, 1000.000000000000227 ) ;
#18298=CARTESIAN_POINT ( 'NONE',  ( -88.16317630448737930, 88.23127654838400247, 52.93781122257118454 ) ) ;
#18303=CARTESIAN_POINT ( 'NONE',  ( 70.11017230969866887, 70.50928942481357353, 84.76194619987022350 ) ) ;
#18312=VERTEX_POINT ( 'NONE', #2517 ) ;
#18315=EDGE_CURVE ( 'NONE', #7696, #20154, #6520, .T. ) ;
#18342=EDGE_CURVE ( 'NONE', #16500, #5147, #4664, .T. ) ;
#18343=CARTESIAN_POINT ( 'NONE',  ( -69.26439091410644266, 97.43560758832659019, 77.57060057039426226 ) ) ;
#18344=ADVANCED_FACE ( 'NONE', ( #6423 ), #16880, .T. ) ;
#18350=B_SPLINE_CURVE_WITH_KNOTS ( 'NONE', 3,
 ( #21339, #9040, #16094, #16642, #7768, #16515, #5609, #21753, #7221, #13302, #19926, #15022, #11224, #6276 ),
 .UNSPECIFIED., .F., .F.,
 ( 4, 2, 2, 2, 2, 2, 4 ),
 ( 0.000000000000000000, 0.001584441135952660389, 0.003168882271905320777, 0.003961102839881667885, 0.004753323407858014993, 0.005545543975834362101, 0.006337764543810709209 ),
 .UNSPECIFIED. ) ;
#18355=FACE_OUTER_BOUND ( 'NONE', #7943, .T. ) ;
#18357=ADVANCED_FACE ( 'NONE', ( #13333 ), #13439, .T. ) ;
#18358=VERTEX_POINT ( 'NONE', #11697 ) ;
#18359=CARTESIAN_POINT ( 'NONE',  ( 39.39497909003009823, 91.17157287525387233, -85.51628863845822082 ) ) ;
#18362=ORIENTED_EDGE ( 'NONE', *, *, #17039, .F. ) ;
#18371=AXIS2_PLACEMENT_3D ( 'NONE', #14407, #16245, #16365 ) ;
#18378=PLANE ( 'NONE',  #2159 ) ;
#18379=CARTESIAN_POINT ( 'NONE',  ( -88.17087551971840753, 88.81088884623601132, 52.22087021872155077 ) ) ;
#18394=EDGE_LOOP ( 'NONE', ( #19476, #19702, #18009, #4611 ) ) ;
#18395=EDGE_CURVE ( 'NONE', #1815, #5416, #18588, .T. ) ;
#18397=AXIS2_PLACEMENT_3D ( 'NONE', #2039, #433, #7550 ) ;
#18407=ORIENTED_EDGE ( 'NONE', *, *, #4136, .F. ) ;
#18414=CARTESIAN_POINT ( 'NONE',  ( -90.17346960859786975, 87.02965620341086606, 51.38002018875397425 ) ) ;
#18418=LINE ( 'NONE', #3167, #1061 ) ;
#18419=CARTESIAN_POINT ( 'NONE',  ( -63.96182961141723666, 99.65143692054147095, 75.28401729384056296 ) ) ;
#18421=VECTOR ( 'NONE', #6187, 1000.000000000000000 ) ;
#18422=CARTESIAN_POINT ( 'NONE',  ( -89.33746586332897266, 79.97654757638649414, -29.19326486971738532 ) ) ;
#18426=EDGE_CURVE ( 'NONE', #17671, #8789, #12926, .T. ) ;
#18427=ORIENTED_EDGE ( 'NONE', *, *, #20735, .T. ) ;
#18435=DIRECTION ( 'NONE',  ( -0.01292414190464044772, 0.000000000000000000, -0.9999164797902015955 ) ) ;
#18437=ORIENTED_EDGE ( 'NONE', *, *, #12969, .T. ) ;
#18446=VERTEX_POINT ( 'NONE', #11101 ) ;
#18447=AXIS2_PLACEMENT_3D ( 'NONE', #10559, #1946, #15867 ) ;
#18448=CARTESIAN_POINT ( 'NONE',  ( 77.67389597125436751, 75.11017898543126137, -5.579058506725625755 ) ) ;
#18457=CARTESIAN_POINT ( 'NONE',  ( -64.14629883989944403, 91.30780077822167584, 66.46930053661340310 ) ) ;
#18459=PLANE ( 'NONE',  #3839 ) ;
#18461=CARTESIAN_POINT ( 'NONE',  ( 91.08520856931308174, 77.44390114805533187, -31.69197020849773239 ) ) ;
#18471=AXIS2_PLACEMENT_3D ( 'NONE', #6735, #13761, #16996 ) ;
#18472=CARTESIAN_POINT ( 'NONE',  ( -68.24431907518334128, 70.78648125535667646, 86.27145290589803039 ) ) ;
#18483=CARTESIAN_POINT ( 'NONE',  ( -106.8724933792760652, 79.04398536104956463, -26.04362031086678897 ) ) ;
#18484=CARTESIAN_POINT ( 'NONE',  ( -106.1636641531658398, 79.04398536104955042, 28.79715981783285628 ) ) ;
#18494=AXIS2_PLACEMENT_3D ( 'NONE', #15312, #22368, #11621 ) ;
#18495=DIRECTION ( 'NONE',  ( -0.9999164797902015955, -2.001050586450178695E-22, 0.01292414190464131335 ) ) ;
#18509=FACE_OUTER_BOUND ( 'NONE', #21167, .T. ) ;
#18510=EDGE_LOOP ( 'NONE', ( #1529, #146, #4676 ) ) ;
#18511=ADVANCED_FACE ( 'NONE', ( #9727 ), #5885, .T. ) ;
#18512=CARTESIAN_POINT ( 'NONE',  ( 65.91440269377942229, 105.0000000000000000, 70.32555938675403695 ) ) ;
#18515=( BOUNDED_SURFACE ( )  B_SPLINE_SURFACE ( 3, 2, ( 
 ( #1172, #11273, #2664 ),
 ( #18718, #8165, #6096 ),
 ( #16794, #4688, #1046 ),
 ( #833, #22257, #13023 ) ),
 .UNSPECIFIED., .F., .F., .T. ) 
 B_SPLINE_SURFACE_WITH_KNOTS ( ( 4, 4 ),
 ( 3, 3 ),
 ( 5.799006443144740786, 5.860583945225279479 ),
 ( 0.000000000000000000, 1.000000000000000000 ),
 .UNSPECIFIED. ) 
 GEOMETRIC_REPRESENTATION_ITEM ( )  RATIONAL_B_SPLINE_SURFACE ( (
 ( 1.000000000000000000, 0.9016180287879261845, 1.000000000000000000),
 ( 1.000000000000000000, 0.9034913259101577943, 1.000000000000000000),
 ( 1.000000000000000000, 0.9052491015987668144, 1.000000000000000000),
 ( 1.000000000000000000, 0.9068900557993655465, 1.000000000000000000) ) ) 
 REPRESENTATION_ITEM ( '' )  SURFACE ( )  );
#18520=CARTESIAN_POINT ( 'NONE',  ( 83.82126922308901840, 105.0000000000000000, -71.23197895489381892 ) ) ;
#18529=CARTESIAN_POINT ( 'NONE',  ( -88.16267813286435739, 88.17648390085673782, 52.97871766249971159 ) ) ;
#18532=B_SPLINE_CURVE_WITH_KNOTS ( 'NONE', 3,
 ( #3380, #15687, #5733, #4126, #22629, #1770, #19223, #12765, #17522, #702 ),
 .UNSPECIFIED., .F., .F.,
 ( 4, 2, 2, 2, 4 ),
 ( 0.000000000000000000, 0.0004486304370347037745, 0.0008972608740694075491, 0.001345891311104094410, 0.001794521748138781271 ),
 .UNSPECIFIED. ) ;
#18533=CARTESIAN_POINT ( 'NONE',  ( -67.77252605414460618, 99.53959963624815543, 78.34284531778030214 ) ) ;
#18536=CARTESIAN_POINT ( 'NONE',  ( -88.18246585727159470, 88.96524493581522108, 50.92653801520322787 ) ) ;
#18540=EDGE_CURVE ( 'NONE', #5654, #10387, #9257, .T. ) ;
#18541=ORIENTED_EDGE ( 'NONE', *, *, #20378, .F. ) ;
#18546=CARTESIAN_POINT ( 'NONE',  ( 93.07689643981107963, 77.12912189501255966, 28.79946631983735728 ) ) ;
#18556=EDGE_CURVE ( 'NONE', #22275, #6959, #2923, .T. ) ;
#18557=EDGE_CURVE ( 'NONE', #17537, #19075, #8112, .T. ) ;
#18559=CARTESIAN_POINT ( 'NONE',  ( -86.79222083800951282, 104.3814432989690602, -67.58039954014913064 ) ) ;
#18561=CARTESIAN_POINT ( 'NONE',  ( 105.4610200154982067, 77.75225708752515175, -31.27258767819551721 ) ) ;
#18566=PLANE ( 'NONE',  #3060 ) ;
#18569=FACE_OUTER_BOUND ( 'NONE', #20675, .T. ) ;
#18586=CARTESIAN_POINT ( 'NONE',  ( -106.2089377515398780, 77.28919246392742082, -28.62973177816245496 ) ) ;
#18587=DIRECTION ( 'NONE',  ( 0.9999164797902015955, 2.001050586450181282E-22, -0.01292414190463992731 ) ) ;
#18588=LINE ( 'NONE', #14799, #4817 ) ;
#18589=EDGE_LOOP ( 'NONE', ( #22401, #11342, #21514, #4036 ) ) ;
#18600=CARTESIAN_POINT ( 'NONE',  ( 90.46801631146688294, 78.10499069285118878, -32.69910015975909090 ) ) ;
#18602=CARTESIAN_POINT ( 'NONE',  ( 1.117803423002110774, 45.00000000000000000, 109.6947150755565161 ) ) ;
#18603=DIRECTION ( 'NONE',  ( -0.9999164797902017066, -2.001050586450178931E-22, 0.01292414190464131508 ) ) ;
#18609=DIRECTION ( 'NONE',  ( 0.01292414190464179213, 0.000000000000000000, 0.9999164797902017066 ) ) ;
#18626=CARTESIAN_POINT ( 'NONE',  ( -88.16489327553765065, 88.40164337095862379, 52.78994026756070923 ) ) ;
#18628=EDGE_CURVE ( 'NONE', #14863, #4193, #18532, .T. ) ;
#18629=CARTESIAN_POINT ( 'NONE',  ( -70.91392079944854743, 91.17157287525390075, -84.09052168258642723 ) ) ;
#18637=DIRECTION ( 'NONE',  ( 0.01292414190464130988, 0.000000000000000000, 0.9999164797902017066 ) ) ;
#18640=DIRECTION ( 'NONE',  ( -0.01292414190464131335, -1.358703943142685684E-38, -0.9999164797902015955 ) ) ;
#18642=CARTESIAN_POINT ( 'NONE',  ( 88.95538863342427760, 79.66477516473727860, -30.55627054544669363 ) ) ;
#18645=EDGE_CURVE ( 'NONE', #12921, #17177, #7785, .T. ) ;
#18650=CARTESIAN_POINT ( 'NONE',  ( -64.02091254583170610, 100.1262683277930989, 76.17020158700519517 ) ) ;
#18651=ORIENTED_EDGE ( 'NONE', *, *, #21990, .F. ) ;
#18652=EDGE_LOOP ( 'NONE', ( #2756, #5727, #10540, #22199, #3665 ) ) ;
#18658=CARTESIAN_POINT ( 'NONE',  ( -90.06143632372041452, 71.82810837149287408, 60.05335399799299978 ) ) ;
#18660=CARTESIAN_POINT ( 'NONE',  ( 105.7099399341924766, 78.83711888896351638, -30.42080736548479436 ) ) ;
#18669=CARTESIAN_POINT ( 'NONE',  ( 93.58499681124563097, 69.99999999999998579, 57.80872228166916926 ) ) ;
#18681=LINE ( 'NONE', #19013, #873 ) ;
#18684=AXIS2_PLACEMENT_3D ( 'NONE', #15439, #5239, #17453 ) ;
#18693=CARTESIAN_POINT ( 'NONE',  ( 83.58290648752347352, 104.4142135623730638, 71.51152175067952044 ) ) ;
#18697=CIRCLE ( 'NONE', #1465, 85.00000000000002842 ) ;
#18704=SHAPE_DEFINITION_REPRESENTATION ( #19488, #10922 ) ;
#18705=VERTEX_POINT ( 'NONE', #171 ) ;
#18706=FACE_OUTER_BOUND ( 'NONE', #21, .T. ) ;
#18718=CARTESIAN_POINT ( 'NONE',  ( 36.93353118842156135, 92.00280690338281886, -84.44237658585842610 ) ) ;
#18720=DIRECTION ( 'NONE',  ( 0.01292414190464174703, 0.000000000000000000, 0.9999164797902015955 ) ) ;
#18721=VECTOR ( 'NONE', #3687, 1000.000000000000114 ) ;
#18728=DIRECTION ( 'NONE',  ( -0.01292414190464039048, -1.902755938799529063E-22, -0.9999164797902017066 ) ) ;
#18733=ORIENTED_EDGE ( 'NONE', *, *, #6888, .T. ) ;
#18738=CARTESIAN_POINT ( 'NONE',  ( -90.09747616180477792, 88.49262567217745357, 52.75167656980727315 ) ) ;
#18744=CARTESIAN_POINT ( 'NONE',  ( -8.680576889647097616, 86.44926012997954956, -75.23049865080909626 ) ) ;
#18745=DIRECTION ( 'NONE',  ( 2.025474946048326158E-22, -1.000000000000000000, 1.876735158486679638E-22 ) ) ;
#18746=CARTESIAN_POINT ( 'NONE',  ( -88.16651712116340889, 88.54264735233917349, 52.64450902266127486 ) ) ;
#18751=DIRECTION ( 'NONE',  ( -2.459148776294495979E-24, 1.000000000000000000, -1.902597020224326827E-22 ) ) ;
#18753=CARTESIAN_POINT ( 'NONE',  ( 91.15750879531701401, 79.10636023297638530, -28.80946033575594356 ) ) ;
#18754=PLANE ( 'NONE',  #9212 ) ;
#18757=EDGE_CURVE ( 'NONE', #14478, #18024, #17737, .T. ) ;
#18758=DIRECTION ( 'NONE',  ( 0.9999164797902017066, 2.001050586450178931E-22, -0.01292414190464131508 ) ) ;
#18763=B_SPLINE_CURVE_WITH_KNOTS ( 'NONE', 3,
 ( #15337, #8406, #4724, #20467, #5064, #10379, #18642, #15671, #11760, #10151, #11648, #17156, #1427, #18753, #15450, #4957, #9918, #6696 ),
 .UNSPECIFIED., .F., .F.,
 ( 4, 2, 2, 2, 2, 2, 2, 2, 4 ),
 ( 0.000000000000000000, 0.0007972436847030646423, 0.001594487369406129285, 0.002391731054109193927, 0.003188974738812258569, 0.003986218423515323211, 0.004783462108218387854, 0.005580705792921452496, 0.006377949477624517138 ),
 .UNSPECIFIED. ) ;
#18766=ORIENTED_EDGE ( 'NONE', *, *, #12537, .T. ) ;
#18770=EDGE_CURVE ( 'NONE', #959, #9955, #9875, .T. ) ;
#18772=CIRCLE ( 'NONE', #6668, 110.0000000000000000 ) ;
#18780=AXIS2_PLACEMENT_3D ( 'NONE', #11867, #10481, #10370 ) ;
#18792=ORIENTED_EDGE ( 'NONE', *, *, #3754, .F. ) ;
#18796=FACE_OUTER_BOUND ( 'NONE', #9800, .T. ) ;
#18816=DIRECTION ( 'NONE',  ( 0.01292414190464038701, 0.000000000000000000, 0.9999164797902017066 ) ) ;
#18817=CARTESIAN_POINT ( 'NONE',  ( -39.42082737383935154, 91.17157287525388654, 83.51645567887779009 ) ) ;
#18820=AXIS2_PLACEMENT_3D ( 'NONE', #9129, #12607, #5450 ) ;
#18823=DIRECTION ( 'NONE',  ( -0.9999164797902015955, -4.653667080246435885E-16, 0.01292414190464177999 ) ) ;
#18836=DIRECTION ( 'NONE',  ( -2.025474946048326158E-22, 1.000000000000000000, -1.876735158486679638E-22 ) ) ;
#18837=FACE_OUTER_BOUND ( 'NONE', #11805, .T. ) ;
#18842=CARTESIAN_POINT ( 'NONE',  ( 106.0703656581358558, 70.66226986180332403, 29.13909619158252085 ) ) ;
#18844=CARTESIAN_POINT ( 'NONE',  ( -39.42082737383935154, 69.99999999999998579, 83.51645567887779009 ) ) ;
#18845=PLANE ( 'NONE',  #5289 ) ;
#18849=DIRECTION ( 'NONE',  ( -0.9999164797902017066, -2.001050586450179636E-22, 0.01292414190464131508 ) ) ;
#18850=ORIENTED_EDGE ( 'NONE', *, *, #5824, .F. ) ;
#18854=CARTESIAN_POINT ( 'NONE',  ( -88.16512445317465563, 88.42243553698295955, 52.76943054571153624 ) ) ;
#18857=CARTESIAN_POINT ( 'NONE',  ( -73.00030478232707765, 95.66452290628956234, 82.28581592040848136 ) ) ;
#18858=FACE_OUTER_BOUND ( 'NONE', #271, .T. ) ;
#18859=DIRECTION ( 'NONE',  ( 0.9999164797902017066, 2.001050586450177285E-22, -0.01292414190464218071 ) ) ;
#18861=CARTESIAN_POINT ( 'NONE',  ( -88.16543417756993506, 88.45405585956656580, 52.74322918111940339 ) ) ;
#18862=CARTESIAN_POINT ( 'NONE',  ( -89.99335928417744412, 79.29537036754121004, 29.40900737050176517 ) ) ;
#18868=VECTOR ( 'NONE', #15588, 1000.000000000000000 ) ;
#18874=CARTESIAN_POINT ( 'NONE',  ( -38.46706438352712354, 69.99999999999998579, 85.27439087629282710 ) ) ;
#18878=CARTESIAN_POINT ( 'NONE',  ( -90.04217887881287652, 70.01937035445752144, 63.21555236838661784 ) ) ;
#18885=CARTESIAN_POINT ( 'NONE',  ( -108.7507233931858082, 76.71731347669778245, -17.16766896971221712 ) ) ;
#18888=ORIENTED_EDGE ( 'NONE', *, *, #22239, .F. ) ;
#18893=CARTESIAN_POINT ( 'NONE',  ( 90.51848467603717552, 80.22648697776341464, -32.24949179442774039 ) ) ;
#18899=CARTESIAN_POINT ( 'NONE',  ( 93.21002351426729149, 72.00000000000000000, 28.79774562292276840 ) ) ;
#18904=ORIENTED_EDGE ( 'NONE', *, *, #22371, .T. ) ;
#18909=CARTESIAN_POINT ( 'NONE',  ( -68.71681667565957241, 71.82428002877158235, 85.89527988174788220 ) ) ;
#18912=DIRECTION ( 'NONE',  ( 0.01292414190464131335, 0.000000000000000000, 0.9999164797902017066 ) ) ;
#18922=CARTESIAN_POINT ( 'NONE',  ( -0.4135725409484799497, 72.00000000000000000, -31.99732735328654343 ) ) ;
#18932=CARTESIAN_POINT ( 'NONE',  ( -39.40254987707579915, 92.58578643762696458, 84.93055112583746791 ) ) ;
#18950=CARTESIAN_POINT ( 'NONE',  ( 68.71681667565954399, 91.17157287525390075, -85.89527988174788220 ) ) ;
#18956=CARTESIAN_POINT ( 'NONE',  ( 90.14709923383520618, 71.28417594712831828, -63.03576606772374902 ) ) ;
#18957=CARTESIAN_POINT ( 'NONE',  ( -90.14732535998963669, 87.29974025575781127, 51.21605703091586292 ) ) ;
#18961=CARTESIAN_POINT ( 'NONE',  ( -74.66530369357522545, 95.67986229880271765, 80.77815352928402604 ) ) ;
#18965=CARTESIAN_POINT ( 'NONE',  ( 84.08901704884495132, 75.05050884166001879, 2.023140727569861408 ) ) ;
#18966=DIRECTION ( 'NONE',  ( 2.025474946048326158E-22, -1.000000000000000000, 1.876735158486679638E-22 ) ) ;
#18972=DIRECTION ( 'NONE',  ( -0.008205354412248759208, 0.7726059781012496464, -0.6348327927582039232 ) ) ;
#18975=CARTESIAN_POINT ( 'NONE',  ( -65.90110554552374822, 103.0000000000000000, -69.29678410920486442 ) ) ;
#18976=EDGE_CURVE ( 'NONE', #10639, #9934, #9280, .T. ) ;
#18983=ORIENTED_EDGE ( 'NONE', *, *, #10385, .T. ) ;
#18991=CARTESIAN_POINT ( 'NONE',  ( -90.08121473318537653, 71.65624093448303711, 60.24707949207349600 ) ) ;
#18993=CARTESIAN_POINT ( 'NONE',  ( -108.2112308668079095, 76.78797451630623527, 19.89137302265076457 ) ) ;
#19000=AXIS2_PLACEMENT_3D ( 'NONE', #21626, #4529, #2245 ) ;
#19001=CYLINDRICAL_SURFACE ( 'NONE', #18004, 5.099999999999994316 ) ;
#19006=CARTESIAN_POINT ( 'NONE',  ( -91.23438425464435397, 78.34087653192912626, -30.69541483481172861 ) ) ;
#19011=DIRECTION ( 'NONE',  ( 0.01292414190464131335, 0.000000000000000000, 0.9999164797902017066 ) ) ;
#19013=CARTESIAN_POINT ( 'NONE',  ( -88.04457284303852305, 72.00000000000000000, 62.11887076636494953 ) ) ;
#19023=CARTESIAN_POINT ( 'NONE',  ( 109.7386064778677905, 75.43227853978193309, 7.937952133666850152 ) ) ;
#19033=CARTESIAN_POINT ( 'NONE',  ( -1.163172771417704698, 44.99899999999999523, -89.99248318111816047 ) ) ;
#19046=CARTESIAN_POINT ( 'NONE',  ( -93.18417523045798134, 77.12912189496638860, -26.79791266334240873 ) ) ;
#19053=ORIENTED_EDGE ( 'NONE', *, *, #4476, .F. ) ;
#19054=CARTESIAN_POINT ( 'NONE',  ( 106.2089377515399065, 77.12912189496647386, 28.62973177816241588 ) ) ;
#19055=PLANE ( 'NONE',  #11293 ) ;
#19059=ADVANCED_FACE ( 'NONE', ( #2051 ), #1944, .T. ) ;
#19061=EDGE_CURVE ( 'NONE', #16549, #5690, #7449, .T. ) ;
#19064=ORIENTED_EDGE ( 'NONE', *, *, #1683, .F. ) ;
#19067=ORIENTED_EDGE ( 'NONE', *, *, #20291, .T. ) ;
#19068=CARTESIAN_POINT ( 'NONE',  ( 91.85265939091880227, 69.99999999999998579, -60.52463885842053060 ) ) ;
#19069=CARTESIAN_POINT ( 'NONE',  ( -90.04282273172685791, 88.64429409703403451, 52.59290563217275150 ) ) ;
#19072=ORIENTED_EDGE ( 'NONE', *, *, #22371, .F. ) ;
#19073=VECTOR ( 'NONE', #11302, 1000.000000000000000 ) ;
#19075=VERTEX_POINT ( 'NONE', #677 ) ;
#19078=CARTESIAN_POINT ( 'NONE',  ( -1.745728752920420179, 86.14745084375783790, -74.98370060827653560 ) ) ;
#19080=SURFACE_STYLE_FILL_AREA ( #20574 ) ;
#19081=CARTESIAN_POINT ( 'NONE',  ( 85.06848091764891251, 75.00179123396263492, -0.4306469408276333843 ) ) ;
#19083=VERTEX_POINT ( 'NONE', #4321 ) ;
#19084=TOROIDAL_SURFACE ( 'NONE', #12130, 4.000000000000000000, 2.000000000000000000 ) ;
#19096=( BOUNDED_CURVE ( )  B_SPLINE_CURVE ( 3, ( #21613, #14898, #4174, #629 ),
 .UNSPECIFIED., .F., .T. ) 
 B_SPLINE_CURVE_WITH_KNOTS ( ( 4, 4 ),
 ( 0.6960171423055203643, 0.8501495483016222598 ),
 .UNSPECIFIED. ) 
 CURVE ( )  GEOMETRIC_REPRESENTATION_ITEM ( )  RATIONAL_B_SPLINE_CURVE ( ( 1.000000000000000000, 0.9980212464270939998, 0.9980212464270939998, 1.000000000000000000 ) ) 
 REPRESENTATION_ITEM ( '' )  );
#19098=EDGE_LOOP ( 'NONE', ( #9731, #12372, #12691, #8071 ) ) ;
#19101=CARTESIAN_POINT ( 'NONE',  ( -93.23587179807654479, 34.61572286322119396, -30.79757858250321689 ) ) ;
#19109=CARTESIAN_POINT ( 'NONE',  ( -93.58499681124557412, 69.99999999999998579, -57.80872228166919058 ) ) ;
#19115=CARTESIAN_POINT ( 'NONE',  ( 84.78539177974978713, 105.0000000000000000, 70.08164767436862519 ) ) ;
#19116=FACE_OUTER_BOUND ( 'NONE', #2083, .T. ) ;
#19119=CARTESIAN_POINT ( 'NONE',  ( 90.02055463237803679, 34.61572286322119396, -63.21629334023821656 ) ) ;
#19121=CARTESIAN_POINT ( 'NONE',  ( -89.24560213809745335, 80.14548850073745712, -29.69112557292186949 ) ) ;
#19126=DIRECTION ( 'NONE',  ( -2.025474946048326393E-22, 1.000000000000000000, -1.876735158486679873E-22 ) ) ;
#19135=VECTOR ( 'NONE', #18236, 1000.000000000000114 ) ;
#19141=CARTESIAN_POINT ( 'NONE',  ( 41.58451242677340076, 92.58578643762696458, 83.88377541325534992 ) ) ;
#19144=CARTESIAN_POINT ( 'NONE',  ( -92.28892611776123545, 77.12912189496636017, 31.19536062043662739 ) ) ;
#19145=AXIS2_PLACEMENT_3D ( 'NONE', #9999, #4923, #15635 ) ;
#19156=CARTESIAN_POINT ( 'NONE',  ( 37.52478479852118909, 92.78536193179812130, 82.71535724525615763 ) ) ;
#19170=ORIENTED_EDGE ( 'NONE', *, *, #3184, .F. ) ;
#19172=CARTESIAN_POINT ( 'NONE',  ( 106.7230861007157472, 79.13476608364855736, 26.64972274501352700 ) ) ;
#19181=ORIENTED_EDGE ( 'NONE', *, *, #22537, .T. ) ;
#19187=CARTESIAN_POINT ( 'NONE',  ( 90.64004788018706904, 70.55772556090482794, -62.32501834406217256 ) ) ;
#19188=CARTESIAN_POINT ( 'NONE',  ( -90.04229551167981072, 87.63269930271252406, 51.01256596538104304 ) ) ;
#19189=CARTESIAN_POINT ( 'NONE',  ( -63.99205529224568068, 99.43075776215394512, 78.40283286226222970 ) ) ;
#19196=CARTESIAN_POINT ( 'NONE',  ( -73.09270779449821021, 95.74768611921976458, 82.20384009048147789 ) ) ;
#19198=PRESENTATION_STYLE_ASSIGNMENT (( #15663 ) ) ;
#19199=CARTESIAN_POINT ( 'NONE',  ( 84.59857130917060886, 75.02669947309938436, 1.163726430838213810 ) ) ;
#19202=ORIENTED_EDGE ( 'NONE', *, *, #6832, .F. ) ;
#19205=CARTESIAN_POINT ( 'NONE',  ( -75.43851917653510952, 75.02636992936612614, -1.284289157548322624 ) ) ;
#19206=B_SPLINE_CURVE_WITH_KNOTS ( 'NONE', 3,
 ( #4743, #7976, #15251, #18993, #4863, #22204, #6497, #21967, #13291, #11666, #1107, #18885, #4532, #1338 ),
 .UNSPECIFIED., .F., .F.,
 ( 4, 2, 2, 2, 2, 2, 4 ),
 ( 0.05403846203490995925, 0.06102746434071378012, 0.06801646664651760099, 0.08199447125812525661, 0.08898347356392907748, 0.09597247586973289835, 0.1099504804813405401 ),
 .UNSPECIFIED. ) ;
#19208=CARTESIAN_POINT ( 'NONE',  ( -105.5454984634618114, 78.31265485325657494, 30.98643060412755901 ) ) ;
#19211=CARTESIAN_POINT ( 'NONE',  ( -35.95309506732429128, 93.50464841319750064, -82.03286182426641915 ) ) ;
#19212=AXIS2_PLACEMENT_3D ( 'NONE', #13256, #6863, #20233 ) ;
#19213=EDGE_CURVE ( 'NONE', #15796, #15089, #7790, .T. ) ;
#19218=AXIS2_PLACEMENT_3D ( 'NONE', #10709, #17500, #22508 ) ;
#19223=CARTESIAN_POINT ( 'NONE',  ( -90.66884163116230866, 70.40480925447369032, 62.28309067965741974 ) ) ;
#19225=AXIS2_PLACEMENT_3D ( 'NONE', #1332, #20479, #10391 ) ;
#19227=DIRECTION ( 'NONE',  ( 0.01292414190463136471, 0.000000000000000000, 0.9999164797902019286 ) ) ;
#19229=CARTESIAN_POINT ( 'NONE',  ( -64.02946135753127521, 99.82858438784199961, 75.50879615180311077 ) ) ;
#19237=AXIS2_PLACEMENT_3D ( 'NONE', #19288, #8603, #6879 ) ;
#19239=CARTESIAN_POINT ( 'NONE',  ( -39.42082737383935154, 69.99999999999998579, 83.51645567887779009 ) ) ;
#19243=CARTESIAN_POINT ( 'NONE',  ( -92.25740333814806604, 79.89798572913885266, -28.97539206162185366 ) ) ;
#19254=ORIENTED_EDGE ( 'NONE', *, *, #9033, .T. ) ;
#19258=DIRECTION ( 'NONE',  ( 0.000000000000000000, -1.000000000000000000, 3.469446951953611033E-15 ) ) ;
#19261=CARTESIAN_POINT ( 'NONE',  ( 39.40254987707581336, 92.58578643762697880, -84.93055112583749633 ) ) ;
#19264=CARTESIAN_POINT ( 'NONE',  ( -90.59090487622916044, 77.87375801460382263, 32.35420311765519585 ) ) ;
#19267=CIRCLE ( 'NONE', #578, 83.00000000000002842 ) ;
#19277=DIRECTION ( 'NONE',  ( 0.9999164797902015955, 2.001050586450178695E-22, -0.01292414190464131335 ) ) ;
#19278=DIRECTION ( 'NONE',  ( -0.01292414190464131335, -1.902755938799530239E-22, -0.9999164797902015955 ) ) ;
#19287=VERTEX_POINT ( 'NONE', #16660 ) ;
#19288=CARTESIAN_POINT ( 'NONE',  ( -91.62437796271721879, 34.61572286322119396, -60.86849236629028326 ) ) ;
#19301=CARTESIAN_POINT ( 'NONE',  ( -90.09224011917365260, 87.50613751784533179, 51.09010363202818894 ) ) ;
#19304=ORIENTED_EDGE ( 'NONE', *, *, #17355, .F. ) ;
#19308=ADVANCED_FACE ( 'NONE', ( #11815 ), #11931, .F. ) ;
#19310=CARTESIAN_POINT ( 'NONE',  ( -35.60051853910361075, 93.98889162522327467, 83.40423953877066765 ) ) ;
#19311=CARTESIAN_POINT ( 'NONE',  ( 81.24851531246423519, 75.12795917139311541, -5.979890628633788729 ) ) ;
#19318=CARTESIAN_POINT ( 'NONE',  ( -77.67539104474651879, 75.11021523748624418, 5.579831338258102846 ) ) ;
#19320=CARTESIAN_POINT ( 'NONE',  ( 88.41758806590424058, 80.31838830481383695, -32.48564084813595798 ) ) ;
#19328=VERTEX_POINT ( 'NONE', #5576 ) ;
#19340=CARTESIAN_POINT ( 'NONE',  ( -2.067862704742604141, 69.99999999999998579, -159.9866367664322979 ) ) ;
#19342=ADVANCED_FACE ( 'NONE', ( #17790 ), #12380, .T. ) ;
#19346=CARTESIAN_POINT ( 'NONE',  ( 90.50635355031315044, 79.35163122866354968, 27.25632624755930067 ) ) ;
#19347=LINE ( 'NONE', #16283, #10655 ) ;
#19352=DIRECTION ( 'NONE',  ( -0.01292414190464131335, -1.902755938799530239E-22, -0.9999164797902015955 ) ) ;
#19353=ORIENTED_EDGE ( 'NONE', *, *, #2325, .T. ) ;
#19354=CARTESIAN_POINT ( 'NONE',  ( -89.33542534687488512, 79.97945796766208559, -29.20190675877561759 ) ) ;
#19362=ORIENTED_EDGE ( 'NONE', *, *, #6704, .F. ) ;
#19365=CARTESIAN_POINT ( 'NONE',  ( -66.06691928577359363, 94.02752048664900997, -82.12548041065298321 ) ) ;
#19371=VECTOR ( 'NONE', #1461, 999.9999999999998863 ) ;
#19379=CYLINDRICAL_SURFACE ( 'NONE', #7687, 6.499999999999998224 ) ;
#19383=DIRECTION ( 'NONE',  ( 2.025474946048326158E-22, -1.000000000000000000, 1.876735158486678933E-22 ) ) ;
#19389=FACE_OUTER_BOUND ( 'NONE', #8064, .T. ) ;
#19396=DIRECTION ( 'NONE',  ( -0.01292414190464131335, -1.902755938799530239E-22, -0.9999164797902015955 ) ) ;
#19397=ORIENTED_EDGE ( 'NONE', *, *, #10367, .T. ) ;
#19410=CARTESIAN_POINT ( 'NONE',  ( -89.59931147023513631, 89.08017288857402605, 51.79292875781501948 ) ) ;
#19419=CARTESIAN_POINT ( 'NONE',  ( 83.15649767528586267, 75.08639547911840850, 2.980377557322682502 ) ) ;
#19424=ORIENTED_EDGE ( 'NONE', *, *, #4969, .T. ) ;
#19428=CARTESIAN_POINT ( 'NONE',  ( -77.38242492463166400, 75.10273324658501792, 5.418133580374851377 ) ) ;
#19430=ORIENTED_EDGE ( 'NONE', *, *, #9930, .T. ) ;
#19431=CARTESIAN_POINT ( 'NONE',  ( -105.4610200154982920, 77.75225708752505227, 31.27258767819528984 ) ) ;
#19437=ADVANCED_FACE ( 'NONE', ( #2250 ), #17897, .F. ) ;
#19441=ORIENTED_EDGE ( 'NONE', *, *, #13113, .T. ) ;
#19443=DIRECTION ( 'NONE',  ( 0.01292414190463830014, 0.000000000000000000, 0.9999164797902017066 ) ) ;
#19456=CARTESIAN_POINT ( 'NONE',  ( 91.78322154246586706, 80.00947954930573758, 29.27761720249711530 ) ) ;
#19461=DIRECTION ( 'NONE',  ( -0.009138748381789079875, -0.7071067811865487940, -0.7070477234798316912 ) ) ;
#19465=CARTESIAN_POINT ( 'NONE',  ( -91.69446324238904822, 77.56197482480477845, -29.51646066538620161 ) ) ;
#19466=EDGE_LOOP ( 'NONE', ( #20320, #17406, #13366, #5535 ) ) ;
#19472=DIRECTION ( 'NONE',  ( 0.01105745575040835080, 0.5176938329688192120, 0.8554944932484254139 ) ) ;
#19476=ORIENTED_EDGE ( 'NONE', *, *, #11768, .F. ) ;
#19483=CARTESIAN_POINT ( 'NONE',  ( -91.40888322292894941, 77.29711350638248746, 31.45985873596569959 ) ) ;
#19488=PRODUCT_DEFINITION_SHAPE ( 'NONE', 'NONE',  #12273 ) ;
#19496=VECTOR ( 'NONE', #7511, 1000.000000000000114 ) ;
#19500=CARTESIAN_POINT ( 'NONE',  ( 37.86419661074339871, 93.64690829566114871, 82.87065082833630925 ) ) ;
#19506=LINE ( 'NONE', #8817, #1227 ) ;
#19510=CARTESIAN_POINT ( 'NONE',  ( 38.46180957136368761, 93.08398165842311300, -84.42015501544466360 ) ) ;
#19519=DIRECTION ( 'NONE',  ( -0.9999164797902015955, -2.001050586450181282E-22, 0.01292414190463992731 ) ) ;
#19520=APPLICATION_CONTEXT ( 'automotive_design' ) ;
#19521=CARTESIAN_POINT ( 'NONE',  ( 37.04297230413862962, 93.86474644718838078, 82.35129237346917819 ) ) ;
#19525=AXIS2_PLACEMENT_3D ( 'NONE', #12823, #7539, #16820 ) ;
#19531=CARTESIAN_POINT ( 'NONE',  ( -90.08557003309165623, 87.52532468786372988, 51.07836697400083636 ) ) ;
#19533=ADVANCED_BREP_SHAPE_REPRESENTATION ( '', ( #17376, #6292 ), #8126 ) ;
#19536=ORIENTED_EDGE ( 'NONE', *, *, #1683, .T. ) ;
#19537=CARTESIAN_POINT ( 'NONE',  ( -106.2089377515398780, 72.00000000000000000, -28.62973177816246206 ) ) ;
#19540=CARTESIAN_POINT ( 'NONE',  ( -105.7941983518662852, 70.06152065884128888, -30.12648231254621933 ) ) ;
#19546=CARTESIAN_POINT ( 'NONE',  ( -1.124400345703740589, 72.00000000000000000, -86.99273374174759965 ) ) ;
#19548=CARTESIAN_POINT ( 'NONE',  ( -75.03994275328706465, 75.00864948959272738, 2.293017013057943032 ) ) ;
#19552=VERTEX_POINT ( 'NONE', #11325 ) ;
#19560=ORIENTED_EDGE ( 'NONE', *, *, #17750, .T. ) ;
#19565=CARTESIAN_POINT ( 'NONE',  ( -1.079165849037536207, 45.00000000000000000, -83.49302606248184588 ) ) ;
#19571=CARTESIAN_POINT ( 'NONE',  ( 89.40485731804140812, 79.89806915697582212, 28.95844815008357287 ) ) ;
#19573=FACE_OUTER_BOUND ( 'NONE', #1862, .T. ) ;
#19577=AXIS2_PLACEMENT_3D ( 'NONE', #6099, #13125, #20095 ) ;
#19582=VECTOR ( 'NONE', #17797, 1000.000000000000114 ) ;
#19586=CARTESIAN_POINT ( 'NONE',  ( -88.18357460598782893, 87.01269140057722495, 51.36456657205789611 ) ) ;
#19595=CARTESIAN_POINT ( 'NONE',  ( -91.85126960211907488, 79.84876637418224732, 31.24149931482875786 ) ) ;
#19596=DIRECTION ( 'NONE',  ( 0.9999164797902017066, 2.001050586450180576E-22, -0.01292414190464044946 ) ) ;
#19606=EDGE_CURVE ( 'NONE', #567, #10181, #17009, .T. ) ;
#19616=ORIENTED_EDGE ( 'NONE', *, *, #2935, .F. ) ;
#19622=DIRECTION ( 'NONE',  ( 0.9999164797902017066, 0.000000000000000000, -0.01292414190463832269 ) ) ;
#19626=CARTESIAN_POINT ( 'NONE',  ( 22.19183229621111053, 88.61243608327089305, 77.38960444610528100 ) ) ;
#19631=VERTEX_POINT ( 'NONE', #14918 ) ;
#19632=CARTESIAN_POINT ( 'NONE',  ( -92.82229925712799457, 69.99999999999998579, 1.199748770783155338 ) ) ;
#19633=CARTESIAN_POINT ( 'NONE',  ( -88.16803135499490907, 88.64744638044348335, 52.50087471490518709 ) ) ;
#19639=CARTESIAN_POINT ( 'NONE',  ( 1.364374644014609697E-14, 69.99999999999998579, -9.836443712999143722E-15 ) ) ;
#19642=CARTESIAN_POINT ( 'NONE',  ( -33.82085273160089400, 93.50464841319747222, 82.93470554904384073 ) ) ;
#19651=DIRECTION ( 'NONE',  ( -0.01292414190463830014, 0.000000000000000000, -0.9999164797902017066 ) ) ;
#19656=ORIENTED_EDGE ( 'NONE', *, *, #18540, .F. ) ;
#19657=CARTESIAN_POINT ( 'NONE',  ( -1.247179693797872524, 45.00000000000000000, -96.49194029975447506 ) ) ;
#19658=ORIENTED_EDGE ( 'NONE', *, *, #219, .F. ) ;
#19659=ORIENTED_EDGE ( 'NONE', *, *, #21735, .T. ) ;
#19660=CARTESIAN_POINT ( 'NONE',  ( -84.38495553179255637, 75.03402262061140959, 3.648261192032123734 ) ) ;
#19669=FACE_OUTER_BOUND ( 'NONE', #20556, .T. ) ;
#19671=CARTESIAN_POINT ( 'NONE',  ( 91.52774025374780820, 80.10656073859405524, 29.55378794065032366 ) ) ;
#19678=CARTESIAN_POINT ( 'NONE',  ( -91.78322154246579601, 80.00947954930759920, -29.27761720249670674 ) ) ;
#19696=CARTESIAN_POINT ( 'NONE',  ( -90.41664810497505300, 79.20851322806753103, 29.13399567714558103 ) ) ;
#19697=DIRECTION ( 'NONE',  ( -0.01292414190464131508, -1.902755938799530474E-22, -0.9999164797902017066 ) ) ;
#19698=ORIENTED_EDGE ( 'NONE', *, *, #15011, .F. ) ;
#19702=ORIENTED_EDGE ( 'NONE', *, *, #22444, .F. ) ;
#19721=CARTESIAN_POINT ( 'NONE',  ( -68.60435330951924016, 89.65606824129204711, 68.66099709659675909 ) ) ;
#19734=CARTESIAN_POINT ( 'NONE',  ( -88.18706637290617323, 88.71869973106707619, 50.32066939225175872 ) ) ;
#19735=EDGE_CURVE ( 'NONE', #19747, #12598, #10027, .T. ) ;
#19744=CARTESIAN_POINT ( 'NONE',  ( -106.2089377515398780, 72.00000000000000000, -28.62973177816246206 ) ) ;
#19746=CARTESIAN_POINT ( 'NONE',  ( 68.99891043397283852, 92.11203426037261011, -85.66888312730657162 ) ) ;
#19747=VERTEX_POINT ( 'NONE', #19109 ) ;
#19750=EDGE_LOOP ( 'NONE', ( #15369, #13559, #15920, #4952 ) ) ;
#19762=ORIENTED_EDGE ( 'NONE', *, *, #6832, .T. ) ;
#19764=ORIENTED_EDGE ( 'NONE', *, *, #10367, .F. ) ;
#19765=CARTESIAN_POINT ( 'NONE',  ( -105.0182314695230446, 70.09775045434527385, 32.72898861654373093 ) ) ;
#19774=CARTESIAN_POINT ( 'NONE',  ( -36.24790013166014546, 94.37751527644311977, -82.16087381192814121 ) ) ;
#19778=CARTESIAN_POINT ( 'NONE',  ( 397.1141114976279027, 91.17157287525388654, 77.87414493559199968 ) ) ;
#19781=DIRECTION ( 'NONE',  ( -0.01292414190464131335, 0.000000000000000000, -0.9999164797902017066 ) ) ;
#19782=CIRCLE ( 'NONE', #22665, 2.000000000000001776 ) ;
#19784=LINE ( 'NONE', #2018, #6627 ) ;
#19786=VERTEX_POINT ( 'NONE', #7172 ) ;
#19791=EDGE_CURVE ( 'NONE', #12496, #12459, #12605, .T. ) ;
#19792=VECTOR ( 'NONE', #14476, 1000.000000000000114 ) ;
#19796=CARTESIAN_POINT ( 'NONE',  ( -38.69757710431294839, 94.02752048664900997, -82.47923521851862461 ) ) ;
#19797=CARTESIAN_POINT ( 'NONE',  ( -89.40428028770215008, 69.94497429273697264, 63.29600751891009480 ) ) ;
#19800=B_SPLINE_CURVE_WITH_KNOTS ( 'NONE', 3,
 ( #7236, #5161, #15542, #8841, #1630, #18956, #22493, #12080, #17721, #19187, #15768, #3215, #10240, #20792, #19068, #13808 ),
 .UNSPECIFIED., .F., .F.,
 ( 4, 2, 2, 2, 2, 2, 2, 4 ),
 ( 0.000000000000000000, 0.0002817774770003779266, 0.0005635549540007558532, 0.001127109908001559194, 0.001690664862002362644, 0.002254219816003151348, 0.003381329724004707073, 0.004508439632006262798 ),
 .UNSPECIFIED. ) ;
#19805=EDGE_LOOP ( 'NONE', ( #14746, #14267, #4739, #16002, #20278, #7970, #11309, #21905, #21710, #4927, #661, #600, #10253 ) ) ;
#19810=CARTESIAN_POINT ( 'NONE',  ( 90.90343663577486666, 80.03933989046612396, -31.72203358726163103 ) ) ;
#19811=CARTESIAN_POINT ( 'NONE',  ( 105.4334892372614405, 77.12912189496645965, -31.36525700924962834 ) ) ;
#19813=CARTESIAN_POINT ( 'NONE',  ( -92.43457499998876870, 79.82103140525724427, 31.19724316448927226 ) ) ;
#19815=ORIENTED_EDGE ( 'NONE', *, *, #7112, .F. ) ;
#19821=ORIENTED_EDGE ( 'NONE', *, *, #1301, .T. ) ;
#19824=VECTOR ( 'NONE', #1104, 999.9999999999998863 ) ;
#19837=CARTESIAN_POINT ( 'NONE',  ( -67.11636521215302764, 90.33521852268984276, 68.08362892527694044 ) ) ;
#19842=CARTESIAN_POINT ( 'NONE',  ( -91.62437796271721879, 72.00000000000000000, -60.86849236629028326 ) ) ;
#19843=B_SPLINE_CURVE_WITH_KNOTS ( 'NONE', 3,
 ( #2406, #16433, #4326, #13099, #18253, #9512 ),
 .UNSPECIFIED., .F., .F.,
 ( 4, 2, 4 ),
 ( 0.000000000000000000, 0.0009893175791656075909, 0.001978635158331215182 ),
 .UNSPECIFIED. ) ;
#19852=CARTESIAN_POINT ( 'NONE',  ( -89.87294000974075914, 87.92385784770752366, 50.83317552486207092 ) ) ;
#19853=EDGE_CURVE ( 'NONE', #19287, #12921, #5257, .T. ) ;
#19854=VECTOR ( 'NONE', #11158, 1000.000000000000114 ) ;
#19856=ORIENTED_EDGE ( 'NONE', *, *, #3932, .T. ) ;
#19860=CARTESIAN_POINT ( 'NONE',  ( 1.247179693797900502, 45.00000000000000000, 96.49194029975444664 ) ) ;
#19868=VERTEX_POINT ( 'NONE', #10511 ) ;
#19869=DIRECTION ( 'NONE',  ( 0.9999164797902017066, 2.001050586450179871E-22, -0.01292414190464085018 ) ) ;
#19874=VECTOR ( 'NONE', #8031, 1000.000000000000114 ) ;
#19875=AXIS2_PLACEMENT_3D ( 'NONE', #17216, #4794, #13780 ) ;
#19885=EDGE_LOOP ( 'NONE', ( #11644, #8019, #14714, #11481, #14762, #19923, #19072, #19856, #15667, #4690, #15265, #16171 ) ) ;
#19886=ORIENTED_EDGE ( 'NONE', *, *, #16193, .T. ) ;
#19888=CARTESIAN_POINT ( 'NONE',  ( -80.72910506257878183, 75.13519840835959940, -4.023912070737448055 ) ) ;
#19889=CARTESIAN_POINT ( 'NONE',  ( -88.16232390766455751, 88.13524946876771082, 53.00763616620414354 ) ) ;
#19897=CARTESIAN_POINT ( 'NONE',  ( -89.71476837554281758, 79.66528429935017641, -28.24846625074281548 ) ) ;
#19900=FACE_OUTER_BOUND ( 'NONE', #15248, .T. ) ;
#19903=CARTESIAN_POINT ( 'NONE',  ( 92.94153934368185332, 77.13727434530989058, 28.81475843614362375 ) ) ;
#19914=ADVANCED_FACE ( 'NONE', ( #5893 ), #2222, .F. ) ;
#19918=CARTESIAN_POINT ( 'NONE',  ( -90.39220665717816416, 70.86425073819692955, 61.14263641236500035 ) ) ;
#19923=ORIENTED_EDGE ( 'NONE', *, *, #7824, .T. ) ;
#19926=CARTESIAN_POINT ( 'NONE',  ( 89.90288769592241636, 96.48106732636601635, -63.38356668362104784 ) ) ;
#19928=FACE_OUTER_BOUND ( 'NONE', #17378, .T. ) ;
#19929=EDGE_CURVE ( 'NONE', #9560, #198, #12471, .T. ) ;
#19932=CARTESIAN_POINT ( 'NONE',  ( -90.41742102548464288, 80.31838830481380853, 32.51148913194521839 ) ) ;
#19940=AXIS2_PLACEMENT_3D ( 'NONE', #14859, #12893, #5637 ) ;
#19948=DIRECTION ( 'NONE',  ( 0.9999164797902015955, 2.001050586450177050E-22, -0.01292414190464223796 ) ) ;
#19965=( BOUNDED_SURFACE ( )  B_SPLINE_SURFACE ( 1, 3, ( 
 ( #13953, #14316, #6931, #12362 ),
 ( #8886, #16157, #17881, #19229 ) ),
 .UNSPECIFIED., .F., .F., .T. ) 
 B_SPLINE_SURFACE_WITH_KNOTS ( ( 2, 2 ),
 ( 4, 4 ),
 ( 0.000000000000000000, 1.000000000000000000 ),
 ( 0.000000000000000000, 1.000000000000000000 ),
 .UNSPECIFIED. ) 
 GEOMETRIC_REPRESENTATION_ITEM ( )  RATIONAL_B_SPLINE_SURFACE ( (
 ( 1.000000000000000000, 0.9946110163663458570, 0.9946110163663458570, 1.000000000000000000),
 ( 1.000000000000000000, 0.9946110163663458570, 0.9946110163663458570, 1.000000000000000000) ) ) 
 REPRESENTATION_ITEM ( '' )  SURFACE ( )  );
#19969=VECTOR ( 'NONE', #18823, 1000.000000000000114 ) ;
#19970=DIRECTION ( 'NONE',  ( -2.459148776294495979E-24, 1.000000000000000000, -1.902597020224326827E-22 ) ) ;
#19971=CARTESIAN_POINT ( 'NONE',  ( -89.76563352250762762, 88.05638224443494266, 50.75096294400219676 ) ) ;
#19975=ORIENTED_EDGE ( 'NONE', *, *, #21978, .F. ) ;
#19978=EDGE_LOOP ( 'NONE', ( #3144, #13447, #14697, #6837 ) ) ;
#19984=CARTESIAN_POINT ( 'NONE',  ( 34.02121088943146532, 93.60248310457335208, -83.02802698561426098 ) ) ;
#19997=ORIENTED_EDGE ( 'NONE', *, *, #7824, .F. ) ;
#20000=CARTESIAN_POINT ( 'NONE',  ( -80.59137632606918089, 75.13524200571961842, 6.109821417268855193 ) ) ;
#20002=CARTESIAN_POINT ( 'NONE',  ( -90.16287545800051362, 87.20002246365963572, 51.27670327837432040 ) ) ;
#20008=CARTESIAN_POINT ( 'NONE',  ( 1.364373935098378649E-14, 105.0000000000000000, -9.836450281572198869E-15 ) ) ;
#20010=CARTESIAN_POINT ( 'NONE',  ( -90.05353287048657762, 71.28481833429248127, 60.66482926606789050 ) ) ;
#20015=DIRECTION ( 'NONE',  ( -0.9999164797902017066, -2.001050586450178931E-22, 0.01292414190464131508 ) ) ;
#20034=EDGE_CURVE ( 'NONE', #11300, #14017, #9441, .T. ) ;
#20035=CARTESIAN_POINT ( 'NONE',  ( 75.17704036982685523, 75.01379216013427254, 0.6763203681379648113 ) ) ;
#20041=CARTESIAN_POINT ( 'NONE',  ( -68.73688910937089247, 91.46348651515936012, 85.87923151210681283 ) ) ;
#20042=EDGE_LOOP ( 'NONE', ( #8174, #20415, #5270, #17551 ) ) ;
#20047=FACE_OUTER_BOUND ( 'NONE', #15875, .T. ) ;
#20053=B_SPLINE_CURVE_WITH_KNOTS ( 'NONE', 3,
 ( #7708, #4479, #11510, #11620 ),
 .UNSPECIFIED., .F., .F.,
 ( 4, 4 ),
 ( 0.0002143831494830000448, 0.0008144042056134326562 ),
 .UNSPECIFIED. ) ;
#20058=DIRECTION ( 'NONE',  ( 0.9999164797902017066, 2.001050586450178931E-22, -0.01292414190464131508 ) ) ;
#20069=DIRECTION ( 'NONE',  ( -0.01292414190464023262, 0.000000000000000000, -0.9999164797902017066 ) ) ;
#20072=CARTESIAN_POINT ( 'NONE',  ( 26.51110539662167298, 89.80349391623344957, 78.56384651380399475 ) ) ;
#20074=LINE ( 'NONE', #2753, #2045 ) ;
#20079=CARTESIAN_POINT ( 'NONE',  ( -89.32895058079316186, 89.12709046313005956, 51.43971369372994928 ) ) ;
#20086=CARTESIAN_POINT ( 'NONE',  ( 64.07473967894682687, 105.0000000000000000, -72.00569783435743432 ) ) ;
#20092=CARTESIAN_POINT ( 'NONE',  ( -68.08232934915048418, 97.72070053556842595, 80.16590062297730412 ) ) ;
#20095=DIRECTION ( 'NONE',  ( -0.01292414190463830014, 0.000000000000000000, -0.9999164797902017066 ) ) ;
#20098=ORIENTED_EDGE ( 'NONE', *, *, #14559, .F. ) ;
#20101=CARTESIAN_POINT ( 'NONE',  ( -1.163172771417704698, 45.00000000000000000, -89.99248318111816047 ) ) ;
#20106=CARTESIAN_POINT ( 'NONE',  ( -82.60517719326530539, 75.10270664613311453, -3.349685274425296289 ) ) ;
#20107=CARTESIAN_POINT ( 'NONE',  ( -90.14611826098273184, 88.22591548105474146, 52.97392334573774519 ) ) ;
#20110=CARTESIAN_POINT ( 'NONE',  ( -66.71921353929309362, 98.29062372165722650, 79.57831125914253789 ) ) ;
#20113=CARTESIAN_POINT ( 'NONE',  ( -92.64101326278360204, 79.05197601643141070, -26.25411123107253530 ) ) ;
#20114=CARTESIAN_POINT ( 'NONE',  ( 396.0414077195426898, 177.0000000000003695, -5.118922886994747401 ) ) ;
#20119=CARTESIAN_POINT ( 'NONE',  ( 93.21002351426729149, 77.12912189496637438, 28.79774562292276840 ) ) ;
#20124=B_SPLINE_CURVE_WITH_KNOTS ( 'NONE', 3,
 ( #8067, #21940, #22059, #22180, #18536, #20575, #11535, #6473, #1419, #20460, #11872, #4716, #11752, #18746, #18861, #8396, #6686, #15441 ),
 .UNSPECIFIED., .F., .F.,
 ( 4, 2, 2, 2, 2, 2, 2, 2, 4 ),
 ( -8.963567119963375336E-06, 0.0003869120770741988550, 0.0007827877212683610753, 0.001178663365462523241, 0.001574539009656685407, 0.001970414653850847790, 0.002366290298045010173, 0.002762165942239172122, 0.003158041586433334505 ),
 .UNSPECIFIED. ) ;
#20139=CARTESIAN_POINT ( 'NONE',  ( 76.19828175484278177, 75.05963785504690122, 2.389257670094249164 ) ) ;
#20151=CARTESIAN_POINT ( 'NONE',  ( 89.97519728687149154, 79.29963411167463505, -29.42247391813773660 ) ) ;
#20154=VERTEX_POINT ( 'NONE', #21147 ) ;
#20158=ORIENTED_EDGE ( 'NONE', *, *, #21407, .F. ) ;
#20164=AXIS2_PLACEMENT_3D ( 'NONE', #6051, #4200, #657 ) ;
#20167=FACE_OUTER_BOUND ( 'NONE', #19885, .T. ) ;
#20168=EDGE_CURVE ( 'NONE', #984, #2805, #17852, .T. ) ;
#20173=DIRECTION ( 'NONE',  ( -2.025474946048326158E-22, 1.000000000000000000, -1.876735158486679638E-22 ) ) ;
#20175=CYLINDRICAL_SURFACE ( 'NONE', #906, 2.000000000000001332 ) ;
#20178=ORIENTED_EDGE ( 'NONE', *, *, #13583, .F. ) ;
#20181=DIRECTION ( 'NONE',  ( -0.01292414190463827932, 0.000000000000000000, -0.9999164797902018176 ) ) ;
#20185=EDGE_CURVE ( 'NONE', #1581, #11360, #13926, .T. ) ;
#20188=VECTOR ( 'NONE', #4003, 1000.000000000000000 ) ;
#20190=AXIS2_PLACEMENT_3D ( 'NONE', #20625, #17185, #20836 ) ;
#20192=B_SPLINE_CURVE_WITH_KNOTS ( 'NONE', 3,
 ( #3711, #5545, #10850, #4164 ),
 .UNSPECIFIED., .F., .F.,
 ( 4, 4 ),
 ( 0.000000000000000000, 0.001506161017265817467 ),
 .UNSPECIFIED. ) ;
#20195=CARTESIAN_POINT ( 'NONE',  ( -88.17377687331638469, 88.93069077600954131, 51.92116411951112553 ) ) ;
#20198=VERTEX_POINT ( 'NONE', #3573 ) ;
#20200=CARTESIAN_POINT ( 'NONE',  ( 91.34851551837616057, 77.30892464375352802, -31.47853330177477460 ) ) ;
#20210=CARTESIAN_POINT ( 'NONE',  ( 39.42082737383937996, 69.99999999999998579, -83.51645567887783272 ) ) ;
#20213=CARTESIAN_POINT ( 'NONE',  ( -41.56623493000981284, 69.99999999999998579, -82.46967996629571473 ) ) ;
#20222=DIRECTION ( 'NONE',  ( -0.01292414190464131335, -1.358703943142685684E-38, -0.9999164797902015955 ) ) ;
#20223=ORIENTED_EDGE ( 'NONE', *, *, #18315, .F. ) ;
#20231=CARTESIAN_POINT ( 'NONE',  ( -90.17115648626537450, 87.10657506226966973, 51.33342129164628886 ) ) ;
#20233=DIRECTION ( 'NONE',  ( -0.01292414190464044772, -8.765831891243140473E-39, -0.9999164797902015955 ) ) ;
#20235=VERTEX_POINT ( 'NONE', #5516 ) ;
#20245=DIRECTION ( 'NONE',  ( -0.9999164797902015955, -2.001050586450178695E-22, 0.01292414190464131335 ) ) ;
#20248=DIRECTION ( 'NONE',  ( 0.01292414190464131508, 0.000000000000000000, 0.9999164797902017066 ) ) ;
#20255=DIRECTION ( 'NONE',  ( 0.9999164797902017066, 2.001050586450178931E-22, -0.01292414190464131508 ) ) ;
#20256=EDGE_LOOP ( 'NONE', ( #6179, #11763, #21511, #17164 ) ) ;
#20267=CARTESIAN_POINT ( 'NONE',  ( 74.89842485966445906, 75.00001493645878270, -0.6274227567034913466 ) ) ;
#20278=ORIENTED_EDGE ( 'NONE', *, *, #8501, .F. ) ;
#20280=DIRECTION ( 'NONE',  ( -0.9999164797902015955, -2.001050586450178695E-22, 0.01292414190464131335 ) ) ;
#20282=CARTESIAN_POINT ( 'NONE',  ( -110.3526887502521561, 77.12912189496638860, -26.57600582461509475 ) ) ;
#20287=AXIS2_PLACEMENT_3D ( 'NONE', #10528, #2029, #9130 ) ;
#20290=EDGE_CURVE ( 'NONE', #14492, #5147, #10797, .T. ) ;
#20291=EDGE_CURVE ( 'NONE', #7696, #9627, #8965, .T. ) ;
#20292=DIRECTION ( 'NONE',  ( -0.9999164797902015955, -2.001050586450179636E-22, 0.01292414190464084844 ) ) ;
#20311=DIRECTION ( 'NONE',  ( -2.025474946048326158E-22, 1.000000000000000000, -1.876735158486679638E-22 ) ) ;
#20316=UNCERTAINTY_MEASURE_WITH_UNIT (LENGTH_MEASURE( 1.000000000000000082E-05 ), #12330, 'distance_accuracy_value', 'NONE');
#20320=ORIENTED_EDGE ( 'NONE', *, *, #18342, .F. ) ;
#20324=EDGE_CURVE ( 'NONE', #9955, #1394, #13810, .T. ) ;
#20325=CARTESIAN_POINT ( 'NONE',  ( 38.46706438352715196, 91.17157287525388654, -85.27439087629288395 ) ) ;
#20333=CARTESIAN_POINT ( 'NONE',  ( 36.07212464706828570, 94.02752048664899576, -83.44565016930062029 ) ) ;
#20340=ADVANCED_FACE ( 'NONE', ( #12673 ), #5982, .T. ) ;
#20343=CARTESIAN_POINT ( 'NONE',  ( 41.59208321381912299, 72.00000000000000000, 84.46951292587608862 ) ) ;
#20344=ORIENTED_EDGE ( 'NONE', *, *, #21990, .T. ) ;
#20350=CARTESIAN_POINT ( 'NONE',  ( -88.16383505568140322, 88.29998048453171577, 52.88219642818270216 ) ) ;
#20358=LINE ( 'NONE', #21941, #2716 ) ;
#20360=EDGE_LOOP ( 'NONE', ( #22527, #5984, #17724, #21444 ) ) ;
#20362=CARTESIAN_POINT ( 'NONE',  ( -88.74294073166163344, 70.70905333810220839, 62.85632276041776123 ) ) ;
#20363=CARTESIAN_POINT ( 'NONE',  ( -64.98709011851474315, 170.4756630735863041, 1.418865331364558058 ) ) ;
#20365=FACE_OUTER_BOUND ( 'NONE', #21852, .T. ) ;
#20372=ORIENTED_EDGE ( 'NONE', *, *, #19735, .F. ) ;
#20378=EDGE_CURVE ( 'NONE', #3397, #18358, #7501, .T. ) ;
#20379=CARTESIAN_POINT ( 'NONE',  ( 105.9973908263408902, 79.15210294646411171, -29.40494008559776518 ) ) ;
#20382=CARTESIAN_POINT ( 'NONE',  ( -90.43474204040838060, 77.12912189496637438, 31.17139488067998343 ) ) ;
#20404=CARTESIAN_POINT ( 'NONE',  ( 109.5708359150300168, 75.34617192694389587, -10.75083194752833826 ) ) ;
#20406=DIRECTION ( 'NONE',  ( -2.025474946048326158E-22, 1.000000000000000000, -1.876735158486679638E-22 ) ) ;
#20411=DIRECTION ( 'NONE',  ( 2.025474946048326158E-22, -1.000000000000000000, 1.876735158486679638E-22 ) ) ;
#20413=ADVANCED_FACE ( 'NONE', ( #18509 ), #10309, .F. ) ;
#20415=ORIENTED_EDGE ( 'NONE', *, *, #16308, .T. ) ;
#20416=DIRECTION ( 'NONE',  ( 0.9999164797902017066, 2.001050586450178931E-22, -0.01292414190464131508 ) ) ;
#20418=LINE ( 'NONE', #11837, #84 ) ;
#20424=CARTESIAN_POINT ( 'NONE',  ( 90.77986998051285639, 77.66088650200015309, -32.02971036561883977 ) ) ;
#20427=LINE ( 'NONE', #8160, #1933 ) ;
#20431=DIRECTION ( 'NONE',  ( -2.025474946048326158E-22, 1.000000000000000000, -1.876735158486679638E-22 ) ) ;
#20433=DIRECTION ( 'NONE',  ( -2.025474946048326158E-22, 1.000000000000000000, -1.876735158486679638E-22 ) ) ;
#20435=ORIENTED_EDGE ( 'NONE', *, *, #7661, .T. ) ;
#20437=DIRECTION ( 'NONE',  ( 0.9999164797902018176, 0.000000000000000000, -0.01292414190463827932 ) ) ;
#20445=ORIENTED_EDGE ( 'NONE', *, *, #18247, .T. ) ;
#20451=CARTESIAN_POINT ( 'NONE',  ( -90.14583285889521846, 87.30743587841715225, 51.21137444554536700 ) ) ;
#20457=DIRECTION ( 'NONE',  ( 2.025474946048326158E-22, -1.000000000000000000, 1.876735158486679638E-22 ) ) ;
#20459=CYLINDRICAL_SURFACE ( 'NONE', #15885, 2.000000000000004885 ) ;
#20460=CARTESIAN_POINT ( 'NONE',  ( -88.17341836116958120, 88.91892192788692739, 51.95902595935821466 ) ) ;
#20461=CARTESIAN_POINT ( 'NONE',  ( -88.83250513209149801, 79.73807450349757175, 30.77911165157504314 ) ) ;
#20467=CARTESIAN_POINT ( 'NONE',  ( 88.55404276674168784, 79.97526064827546577, -31.48874835467967870 ) ) ;
#20469=AXIS2_PLACEMENT_3D ( 'NONE', #8898, #7183, #14215 ) ;
#20474=CARTESIAN_POINT ( 'NONE',  ( -64.00269606583552218, 99.99497935025800643, 77.57957628177221920 ) ) ;
#20479=DIRECTION ( 'NONE',  ( 0.9999164797902017066, 2.001050586450178931E-22, -0.01292414190464131508 ) ) ;
#20481=B_SPLINE_CURVE_WITH_KNOTS ( 'NONE', 3,
 ( #7022, #3351, #19310, #3122, #17604, #1854, #22279, #13588 ),
 .UNSPECIFIED., .F., .F.,
 ( 4, 2, 2, 4 ),
 ( 0.000000000000000000, 0.001422162546572855154, 0.002133243819859289344, 0.002844325093145723751 ),
 .UNSPECIFIED. ) ;
#20485=CARTESIAN_POINT ( 'NONE',  ( -86.05176612644825695, 104.9512348145193528, -68.52150138215246500 ) ) ;
#20488=CARTESIAN_POINT ( 'NONE',  ( -92.60113547278139379, 70.26667278203282763, -59.37223626620097150 ) ) ;
#20489=CYLINDRICAL_SURFACE ( 'NONE', #1467, 2.000000000000001332 ) ;
#20493=FACE_OUTER_BOUND ( 'NONE', #214, .T. ) ;
#20494=CARTESIAN_POINT ( 'NONE',  ( 91.74710091628175235, 71.28171241778765932, 60.68341510339265454 ) ) ;
#20521=DIRECTION ( 'NONE',  ( -2.025474946048326158E-22, 1.000000000000000000, -1.876735158486679638E-22 ) ) ;
#20522=B_SPLINE_CURVE_WITH_KNOTS ( 'NONE', 3,
 ( #17798, #7303, #5584, #2138, #12615, #430, #16189, #7428, #16309, #14575, #4421, #21755, #9834, #9616 ),
 .UNSPECIFIED., .F., .F.,
 ( 4, 2, 2, 2, 2, 2, 4 ),
 ( 0.000000000000000000, 0.001026194940722985208, 0.001539292411084444961, 0.002052389881445904497, 0.003078584822168817930, 0.003591682292530273997, 0.004104779762891730931 ),
 .UNSPECIFIED. ) ;
#20525=AXIS2_PLACEMENT_3D ( 'NONE', #17826, #7331, #575 ) ;
#20530=VECTOR ( 'NONE', #10318, 1000.000000000000114 ) ;
#20534=EDGE_CURVE ( 'NONE', #6487, #2857, #14848, .T. ) ;
#20536=DIRECTION ( 'NONE',  ( -2.025474946048326158E-22, 1.000000000000000000, -1.876735158486679638E-22 ) ) ;
#20539=CIRCLE ( 'NONE', #22358, 109.9999999999999858 ) ;
#20544=VERTEX_POINT ( 'NONE', #22031 ) ;
#20547=VECTOR ( 'NONE', #112, 1000.000000000000000 ) ;
#20548=CARTESIAN_POINT ( 'NONE',  ( 86.05176612644827117, 104.9512348145193528, 68.52150138215245079 ) ) ;
#20556=EDGE_LOOP ( 'NONE', ( #16686, #9619, #16524, #5328 ) ) ;
#20560=ORIENTED_EDGE ( 'NONE', *, *, #7083, .T. ) ;
#20565=CARTESIAN_POINT ( 'NONE',  ( -90.15594448151276197, 87.25008185477516065, 51.24627459905987337 ) ) ;
#20568=CARTESIAN_POINT ( 'NONE',  ( -73.19071663825569374, 95.81335214582355775, 82.11661254133679222 ) ) ;
#20574=FILL_AREA_STYLE ('',( #5173 ) ) ;
#20575=CARTESIAN_POINT ( 'NONE',  ( -88.18033096311128816, 89.00450046955621985, 51.18519472437992590 ) ) ;
#20576=CARTESIAN_POINT ( 'NONE',  ( -92.46788464407291031, 79.04398536104955042, 28.62013883513304080 ) ) ;
#20580=ORIENTED_EDGE ( 'NONE', *, *, #15408, .T. ) ;
#20581=ORIENTED_EDGE ( 'NONE', *, *, #21192, .F. ) ;
#20583=CARTESIAN_POINT ( 'NONE',  ( -71.61338682171090397, 92.58578643762702143, -83.49564556265197268 ) ) ;
#20595=CARTESIAN_POINT ( 'NONE',  ( -64.02925735614492453, 99.81835863910170303, 75.52457935425162816 ) ) ;
#20605=CARTESIAN_POINT ( 'NONE',  ( -88.04920282358598627, 72.63494618757752619, 61.76065790490801533 ) ) ;
#20608=CARTESIAN_POINT ( 'NONE',  ( -93.38631075262969716, 70.00000000000000000, -58.13036983636536803 ) ) ;
#20615=DIRECTION ( 'NONE',  ( -2.025474946048326158E-22, 1.000000000000000000, -1.876735158486679638E-22 ) ) ;
#20619=ORIENTED_EDGE ( 'NONE', *, *, #21534, .F. ) ;
#20625=CARTESIAN_POINT ( 'NONE',  ( 92.40872671617952960, 72.00000000000000000, -33.19707612406969588 ) ) ;
#20629=EDGE_LOOP ( 'NONE', ( #16855, #12263 ) ) ;
#20643=ORIENTED_EDGE ( 'NONE', *, *, #18154, .T. ) ;
#20645=EDGE_LOOP ( 'NONE', ( #9218, #12665, #2355, #3859, #562, #12450 ) ) ;
#20648=LINE ( 'NONE', #1149, #14308 ) ;
#20654=CARTESIAN_POINT ( 'NONE',  ( -90.17340840076944630, 87.01269140061864960, 51.39028561451661403 ) ) ;
#20656=AXIS2_PLACEMENT_3D ( 'NONE', #19778, #20015, #11198 ) ;
#20657=ORIENTED_EDGE ( 'NONE', *, *, #672, .T. ) ;
#20662=DIRECTION ( 'NONE',  ( -0.01292414190463830014, 0.000000000000000000, -0.9999164797902017066 ) ) ;
#20666=AXIS2_PLACEMENT_3D ( 'NONE', #19340, #10396, #10613 ) ;
#20671=DIRECTION ( 'NONE',  ( 2.025474946048326158E-22, -1.000000000000000000, 1.876735158486679638E-22 ) ) ;
#20672=CARTESIAN_POINT ( 'NONE',  ( -85.15765475724558087, 77.82445350946629503, 69.65678843057233394 ) ) ;
#20675=EDGE_LOOP ( 'NONE', ( #10682, #19821, #18183, #14297 ) ) ;
#20677=CARTESIAN_POINT ( 'NONE',  ( -65.93268019054298179, 104.4142135623730780, -71.73965483371374319 ) ) ;
#20682=CARTESIAN_POINT ( 'NONE',  ( -0.9951589266573748205, 72.00000000000000000, -76.99356894384553129 ) ) ;
#20684=CIRCLE ( 'NONE', #2367, 2.000000000000001332 ) ;
#20687=CARTESIAN_POINT ( 'NONE',  ( -90.10158855731272354, 87.47818988973786247, 51.10719583609721894 ) ) ;
#20692=CARTESIAN_POINT ( 'NONE',  ( -26.49735288203455497, 89.79919665824762376, -78.55966460526794037 ) ) ;
#20695=EDGE_CURVE ( 'NONE', #19328, #20235, #20684, .T. ) ;
#20701=DIRECTION ( 'NONE',  ( 0.9999164797902017066, 2.001050586450180576E-22, -0.01292414190464044946 ) ) ;
#20710=CARTESIAN_POINT ( 'NONE',  ( 90.13422078941499649, 99.92632882282073581, 63.05520142610588152 ) ) ;
#20712=( BOUNDED_CURVE ( )  B_SPLINE_CURVE ( 3, ( #14540, #2454, #20010, #9449 ),
 .UNSPECIFIED., .F., .T. ) 
 B_SPLINE_CURVE_WITH_KNOTS ( ( 4, 4 ),
 ( 0.5456322604206232940, 1.570796326794899667 ),
 .UNSPECIFIED. ) 
 CURVE ( )  GEOMETRIC_REPRESENTATION_ITEM ( )  RATIONAL_B_SPLINE_CURVE ( ( 1.000000000000000000, 0.9143207399647593769, 0.9143207399647593769, 1.000000000000000000 ) ) 
 REPRESENTATION_ITEM ( '' )  );
#20716=VERTEX_POINT ( 'NONE', #9020 ) ;
#20717=DIRECTION ( 'NONE',  ( -2.025474946048326158E-22, 1.000000000000000000, -1.876735158486679638E-22 ) ) ;
#20721=CARTESIAN_POINT ( 'NONE',  ( -86.44937305384743809, 104.7459436402722446, -68.01917747034278250 ) ) ;
#20726=EDGE_LOOP ( 'NONE', ( #20806, #3391, #19424, #8970, #13829, #17720, #2590, #3673 ) ) ;
#20727=DIRECTION ( 'NONE',  ( -0.9999164797902017066, -2.001050586450177285E-22, 0.01292414190464223969 ) ) ;
#20732=LINE ( 'NONE', #8548, #18868 ) ;
#20734=CARTESIAN_POINT ( 'NONE',  ( 91.23603883849617091, 79.86121811340019860, 30.82342686631245243 ) ) ;
#20735=EDGE_CURVE ( 'NONE', #13713, #2836, #21638, .T. ) ;
#20736=PLANE ( 'NONE',  #17654 ) ;
#20739=CARTESIAN_POINT ( 'NONE',  ( -91.23603883849615670, 78.43035437438882695, -30.82342686631250572 ) ) ;
#20743=CARTESIAN_POINT ( 'NONE',  ( -70.11017230969864045, 70.50928942481357353, -84.76194619987022350 ) ) ;
#20749=DIRECTION ( 'NONE',  ( 0.9999164797902017066, 2.001050586450178931E-22, -0.01292414190464131508 ) ) ;
#20754=DIRECTION ( 'NONE',  ( -0.9999164797902017066, -2.001050586450180576E-22, 0.01292414190464039048 ) ) ;
#20774=ORIENTED_EDGE ( 'NONE', *, *, #6468, .F. ) ;
#20781=CARTESIAN_POINT ( 'NONE',  ( -92.40872671617950118, 72.00000000000000000, 33.19707612406966746 ) ) ;
#20792=CARTESIAN_POINT ( 'NONE',  ( 91.64606417454449172, 70.03008549560414053, -60.83696323298806163 ) ) ;
#20793=B_SPLINE_CURVE_WITH_KNOTS ( 'NONE', 3,
 ( #2713, #21744, #9726, #18121, #14674, #2371, #9364, #14913, #11217, #20139, #6039, #16401, #4409, #20035, #7630, #14561, #20267, #18224, #9247, #5916, #21519, #12953, #989, #11437, #2476, #7974, #9471, #16507, #6265, #760, #7759, #18448, #15012, #21964, #15468, #6713, #16843, #1105 ),
 .UNSPECIFIED., .F., .F.,
 ( 4, 2, 2, 2, 2, 2, 2, 2, 2, 2, 2, 2, 2, 2, 2, 2, 2, 2, 4 ),
 ( 0.01594779277582532295, 0.01694430233486374573, 0.01794081189390216852, 0.01893732145294058783, 0.01993383101197901061, 0.02093034057101743339, 0.02192685013005585271, 0.02292335968909427549, 0.02391986924813269827, 0.02491637880717111758, 0.02541463358669033418, 0.02591288836620954730, 0.02690939792524796315, 0.02790590748428638246, 0.02890241704332479483, 0.02940067182284402530, 0.02989892660236324884, 0.03089543616140169591, 0.03189194572044014991 ),
 .UNSPECIFIED. ) ;
#20794=CARTESIAN_POINT ( 'NONE',  ( -90.14238824705606135, 87.32442042776537505, 51.20102670897820474 ) ) ;
#20800=LINE ( 'NONE', #8620, #16972 ) ;
#20801=CARTESIAN_POINT ( 'NONE',  ( -22.15772835622063042, 88.61525343264318622, -77.39142602527519443 ) ) ;
#20804=CARTESIAN_POINT ( 'NONE',  ( -71.00742074342183230, 91.74173777283634479, -84.01159762260417097 ) ) ;
#20806=ORIENTED_EDGE ( 'NONE', *, *, #5425, .F. ) ;
#20811=FACE_OUTER_BOUND ( 'NONE', #17397, .T. ) ;
#20814=CARTESIAN_POINT ( 'NONE',  ( -89.23620587891574019, 78.43035437438885538, -30.84927515012178389 ) ) ;
#20815=FACE_OUTER_BOUND ( 'NONE', #527, .T. ) ;
#20825=DIRECTION ( 'NONE',  ( 0.01292414190465215537, 0.000000000000000000, 0.9999164797902015955 ) ) ;
#20833=LINE ( 'NONE', #20734, #8080 ) ;
#20836=DIRECTION ( 'NONE',  ( -0.01292414190463832269, 0.000000000000000000, -0.9999164797902017066 ) ) ;
#20843=ADVANCED_FACE ( 'NONE', ( #4419 ), #18459, .F. ) ;
#20849=CARTESIAN_POINT ( 'NONE',  ( -104.9011368644396640, 70.01236949047485325, 33.10239539927072627 ) ) ;
#20862=DIRECTION ( 'NONE',  ( -0.9999164797902017066, -2.001050586450178931E-22, 0.01292414190464131508 ) ) ;
#20864=LINE ( 'NONE', #3419, #4077 ) ;
#20866=CARTESIAN_POINT ( 'NONE',  ( 87.01081826484191595, 101.8285212125953763, -67.31825406265291178 ) ) ;
#20867=CARTESIAN_POINT ( 'NONE',  ( -71.61338682171090397, 92.58578643762702143, -83.49564556265197268 ) ) ;
#20870=CARTESIAN_POINT ( 'NONE',  ( 38.46706438352715196, 91.17157287525388654, -85.27439087629288395 ) ) ;
#20871=ORIENTED_EDGE ( 'NONE', *, *, #19929, .T. ) ;
#20878=ORIENTED_EDGE ( 'NONE', *, *, #11291, .F. ) ;
#20879=VERTEX_POINT ( 'NONE', #1679 ) ;
#20880=B_SPLINE_CURVE_WITH_KNOTS ( 'NONE', 3,
 ( #17359, #5035, #3446, #19172, #1726, #5491, #5151, #1955, #17587, #10457, #12190, #232, #10229, #22589, #12071, #19054 ),
 .UNSPECIFIED., .F., .F.,
 ( 4, 2, 2, 2, 2, 2, 2, 4 ),
 ( 1.040834085586084257E-17, 0.0004729024035692759587, 0.0009458048071385415090, 0.001891609614277086054, 0.002364512017846342063, 0.002837414421415598072, 0.003310316824984853648, 0.003783219228554109657 ),
 .UNSPECIFIED. ) ;
#20892=VERTEX_POINT ( 'NONE', #20951 ) ;
#20896=CIRCLE ( 'NONE', #4751, 2.000000000000001776 ) ;
#20897=AXIS2_PLACEMENT_3D ( 'NONE', #6365, #8200, #18972 ) ;
#20900=EDGE_LOOP ( 'NONE', ( #22198, #8006, #16376, #20445 ) ) ;
#20902=EDGE_CURVE ( 'NONE', #7368, #17515, #1561, .T. ) ;
#20903=AXIS2_PLACEMENT_3D ( 'NONE', #11470, #20173, #7791 ) ;
#20907=CARTESIAN_POINT ( 'NONE',  ( -88.16945660481133018, 88.73583354750662977, 52.36250520916426865 ) ) ;
#20911=LINE ( 'NONE', #8293, #1521 ) ;
#20913=CARTESIAN_POINT ( 'NONE',  ( -0.9693106428480923187, 86.14745084375785211, -74.99373598426512899 ) ) ;
#20916=CARTESIAN_POINT ( 'NONE',  ( 83.31510742684905324, 75.07738311394993502, -4.918051378794431550 ) ) ;
#20926=CARTESIAN_POINT ( 'NONE',  ( -79.92740525950245001, 75.13699351169597662, 6.133505399301365735 ) ) ;
#20937=ORIENTED_EDGE ( 'NONE', *, *, #3304, .T. ) ;
#20943=CARTESIAN_POINT ( 'NONE',  ( 92.43457499998882554, 77.12912189496645965, -31.19724316448930423 ) ) ;
#20951=CARTESIAN_POINT ( 'NONE',  ( -93.21002351426726307, 77.12912189496638860, -28.79774562292281104 ) ) ;
#20953=ORIENTED_EDGE ( 'NONE', *, *, #18395, .T. ) ;
#20959=CARTESIAN_POINT ( 'NONE',  ( -91.69412133380704688, 80.03889463956294037, -29.36066737363279699 ) ) ;
#20971=ORIENTED_EDGE ( 'NONE', *, *, #235, .F. ) ;
#20974=EDGE_CURVE ( 'NONE', #12496, #16244, #20732, .T. ) ;
#20997=EDGE_CURVE ( 'NONE', #11742, #6632, #5283, .T. ) ;
#21000=LINE ( 'NONE', #15982, #20547 ) ;
#21012=ADVANCED_FACE ( 'NONE', ( #17771 ), #13689, .T. ) ;
#21017=EDGE_CURVE ( 'NONE', #11382, #9044, #7872, .T. ) ;
#21018=CIRCLE ( 'NONE', #9667, 6.499999999999998224 ) ;
#21025=ORIENTED_EDGE ( 'NONE', *, *, #16325, .F. ) ;
#21028=CARTESIAN_POINT ( 'NONE',  ( -89.76607547520649177, 88.98826100381097604, 52.04949514552107814 ) ) ;
#21034=ORIENTED_EDGE ( 'NONE', *, *, #14610, .T. ) ;
#21037=CARTESIAN_POINT ( 'NONE',  ( 85.05181457928490829, 75.00176059250011917, -1.764877938563226500 ) ) ;
#21042=ORIENTED_EDGE ( 'NONE', *, *, #12739, .F. ) ;
#21045=CARTESIAN_POINT ( 'NONE',  ( -75.07425674568773388, 75.00865516402794242, -0.3536922578719212118 ) ) ;
#21049=CARTESIAN_POINT ( 'NONE',  ( -37.04307294938801931, 93.86476689679389551, -82.35130986602069925 ) ) ;
#21051=CARTESIAN_POINT ( 'NONE',  ( 105.4334892372614405, 72.00000000000000000, -31.36525700924962834 ) ) ;
#21056=ORIENTED_EDGE ( 'NONE', *, *, #3883, .F. ) ;
#21060=ORIENTED_EDGE ( 'NONE', *, *, #9581, .T. ) ;
#21069=EDGE_LOOP ( 'NONE', ( #13935, #18407, #22015, #13224 ) ) ;
#21070=DIRECTION ( 'NONE',  ( 0.9999164797902017066, 2.001050586450178931E-22, -0.01292414190464131508 ) ) ;
#21073=CARTESIAN_POINT ( 'NONE',  ( 91.13609774473717096, 79.20914543161380550, 26.78943607724107423 ) ) ;
#21074=CARTESIAN_POINT ( 'NONE',  ( -84.78539177974977292, 105.0000000000000000, -70.08164767436865361 ) ) ;
#21075=AXIS2_PLACEMENT_3D ( 'NONE', #493, #5752, #9557 ) ;
#21076=FACE_OUTER_BOUND ( 'NONE', #17150, .T. ) ;
#21079=CARTESIAN_POINT ( 'NONE',  ( -92.06552853299464800, 79.93537922958711306, -29.07356135706641709 ) ) ;
#21081=AXIS2_PLACEMENT_3D ( 'NONE', #16264, #8875, #19443 ) ;
#21093=CARTESIAN_POINT ( 'NONE',  ( 71.06083360305758845, 91.87225009003579146, 83.96645210693642980 ) ) ;
#21096=CARTESIAN_POINT ( 'NONE',  ( -92.40872671617950118, 69.99999999999998579, 33.19707612406966746 ) ) ;
#21109=EDGE_CURVE ( 'NONE', #1394, #10157, #19096, .T. ) ;
#21112=CARTESIAN_POINT ( 'NONE',  ( -74.89374433628610461, 54.99999999999999289, 0.9680182286576737294 ) ) ;
#21113=CARTESIAN_POINT ( 'NONE',  ( -36.23709397917757258, 94.19957547782705376, 83.27571307199862360 ) ) ;
#21116=DIRECTION ( 'NONE',  ( 0.000000000000000000, 1.000000000000000000, 0.000000000000000000 ) ) ;
#21119=ORIENTED_EDGE ( 'NONE', *, *, #5894, .F. ) ;
#21123=EDGE_CURVE ( 'NONE', #10917, #20879, #6900, .T. ) ;
#21126=ORIENTED_EDGE ( 'NONE', *, *, #15505, .T. ) ;
#21129=DIRECTION ( 'NONE',  ( -0.8077751305149004635, -0.4220031449644254806, -0.4115977212786404160 ) ) ;
#21138=DIRECTION ( 'NONE',  ( -0.01292414190464023262, 0.000000000000000000, -0.9999164797902017066 ) ) ;
#21139=CARTESIAN_POINT ( 'NONE',  ( -89.93251366689203508, 88.82716965768310047, 52.34818047611932457 ) ) ;
#21141=PRODUCT ( 'Upper Movable Jaw Swivel Housing', 'Upper Movable Jaw Swivel Housing', '', ( #1279 ) ) ;
#21144=ORIENTED_EDGE ( 'NONE', *, *, #17041, .T. ) ;
#21146=CARTESIAN_POINT ( 'NONE',  ( 79.92740525950247843, 75.13699351169599083, -6.133505399301336425 ) ) ;
#21147=CARTESIAN_POINT ( 'NONE',  ( 35.95309506732430549, 93.50464841319750064, 82.03286182426640494 ) ) ;
#21152=CARTESIAN_POINT ( 'NONE',  ( 39.75021781620444727, 69.99999999999998579, 86.03367798009509215 ) ) ;
#21162=CARTESIAN_POINT ( 'NONE',  ( 105.3515605809559048, 70.97896074530382293, -31.63944816216644185 ) ) ;
#21164=VERTEX_POINT ( 'NONE', #22189 ) ;
#21167=EDGE_LOOP ( 'NONE', ( #10561, #685, #20223, #19067, #3197, #12770 ) ) ;
#21173=CARTESIAN_POINT ( 'NONE',  ( 92.28892611776127808, 77.12912189496647386, -31.19536062043667357 ) ) ;
#21174=CARTESIAN_POINT ( 'NONE',  ( -91.17321230992149594, 70.18788889246519602, 61.54298701807832828 ) ) ;
#21181=CARTESIAN_POINT ( 'NONE',  ( 91.85896106039241715, 79.10764833873324164, 26.44817522613584515 ) ) ;
#21185=DIRECTION ( 'NONE',  ( -0.01292414190464131508, -1.902755938799530474E-22, -0.9999164797902017066 ) ) ;
#21186=AXIS2_PLACEMENT_3D ( 'NONE', #1823, #8815, #6652 ) ;
#21192=EDGE_CURVE ( 'NONE', #9610, #2301, #21666, .T. ) ;
#21193=DIRECTION ( 'NONE',  ( 0.9999164797902015955, 2.001050586450178695E-22, -0.01292414190464131335 ) ) ;
#21202=CARTESIAN_POINT ( 'NONE',  ( 71.00742074342186072, 91.74173777283633058, 84.01159762260415675 ) ) ;
#21206=CARTESIAN_POINT ( 'NONE',  ( -88.41758806590422637, 80.31838830481380853, 32.48564084813593666 ) ) ;
#21218=CARTESIAN_POINT ( 'NONE',  ( 39.10370113529218372, 92.00280690327063837, 83.45957852174062452 ) ) ;
#21221=CARTESIAN_POINT ( 'NONE',  ( -1.124400345703781001, 69.99999999999998579, -86.99273374174757123 ) ) ;
#21224=VERTEX_POINT ( 'NONE', #8629 ) ;
#21230=FACE_OUTER_BOUND ( 'NONE', #20900, .T. ) ;
#21235=CIRCLE ( 'NONE', #4363, 110.0000000000000142 ) ;
#21240=EDGE_CURVE ( 'NONE', #12967, #14863, #10744, .T. ) ;
#21241=CARTESIAN_POINT ( 'NONE',  ( -89.97667839591423444, 87.76279617797230514, 50.93259715458368220 ) ) ;
#21244=DIRECTION ( 'NONE',  ( -2.025474946048326158E-22, 1.000000000000000000, -1.876735158486679638E-22 ) ) ;
#21245=DIRECTION ( 'NONE',  ( 0.01292414190464131335, 1.902755938799530239E-22, 0.9999164797902015955 ) ) ;
#21247=CARTESIAN_POINT ( 'NONE',  ( -106.1909711380429115, 71.47214965576930013, -28.69631340039675749 ) ) ;
#21250=CARTESIAN_POINT ( 'NONE',  ( 91.57598704441285520, 77.66227243743308861, 29.67486887243840954 ) ) ;
#21253=CIRCLE ( 'NONE', #1471, 2.000000000000004885 ) ;
#21255=DIRECTION ( 'NONE',  ( -0.01292414190463830014, 0.000000000000000000, -0.9999164797902017066 ) ) ;
#21258=ORIENTED_EDGE ( 'NONE', *, *, #3442, .T. ) ;
#21270=ADVANCED_FACE ( 'NONE', ( #20811 ), #18754, .T. ) ;
#21282=ORIENTED_EDGE ( 'NONE', *, *, #18540, .T. ) ;
#21283=CARTESIAN_POINT ( 'NONE',  ( -86.79222083800951282, 104.3814432989690602, -67.58039954014913064 ) ) ;
#21286=CARTESIAN_POINT ( 'NONE',  ( 92.62880990220415356, 79.84869560962943069, 28.85690742247621898 ) ) ;
#21291=CARTESIAN_POINT ( 'NONE',  ( -83.58290648752343088, 104.4142135623730780, -71.51152175067954886 ) ) ;
#21296=AXIS2_PLACEMENT_3D ( 'NONE', #11207, #18217, #18435 ) ;
#21299=CARTESIAN_POINT ( 'NONE',  ( -89.59156723394222865, 79.74270461908911045, -28.48704982653686457 ) ) ;
#21307=AXIS2_PLACEMENT_3D ( 'NONE', #10028, #8392, #13920 ) ;
#21317=CARTESIAN_POINT ( 'NONE',  ( -88.94497886703045708, 79.67058643966740306, 30.57398350459251901 ) ) ;
#21318=CARTESIAN_POINT ( 'NONE',  ( 92.40872671617952960, 72.00000000000000000, -33.19707612406970298 ) ) ;
#21322=ORIENTED_EDGE ( 'NONE', *, *, #15296, .T. ) ;
#21328=CARTESIAN_POINT ( 'NONE',  ( -38.90567791675928078, 92.58578643762697880, 84.92412894573205051 ) ) ;
#21329=AXIS2_PLACEMENT_3D ( 'NONE', #14429, #277, #7735 ) ;
#21334=VECTOR ( 'NONE', #10787, 1000.000000000000114 ) ;
#21339=CARTESIAN_POINT ( 'NONE',  ( 87.98413419613014241, 100.6041916471018851, -66.02114910964037620 ) ) ;
#21343=ORIENTED_EDGE ( 'NONE', *, *, #5705, .T. ) ;
#21344=CARTESIAN_POINT ( 'NONE',  ( -69.95498757883834173, 89.03960924830867896, 69.18506932511724017 ) ) ;
#21349=ORIENTED_EDGE ( 'NONE', *, *, #952, .T. ) ;
#21352=AXIS2_PLACEMENT_3D ( 'NONE', #16854, #6162, #11797 ) ;
#21353=LINE ( 'NONE', #16675, #22333 ) ;
#21356=CARTESIAN_POINT ( 'NONE',  ( -89.90957607858042877, 87.87157606449417813, 50.86550588853232568 ) ) ;
#21360=ORIENTED_EDGE ( 'NONE', *, *, #3061, .T. ) ;
#21368=VERTEX_POINT ( 'NONE', #14754 ) ;
#21369=CARTESIAN_POINT ( 'NONE',  ( 1.364373935098378649E-14, 105.0000000000000000, -9.836450281572198869E-15 ) ) ;
#21377=CARTESIAN_POINT ( 'NONE',  ( -70.64248633631808616, 93.58690533528225330, 84.33313170347786070 ) ) ;
#21379=VERTEX_POINT ( 'NONE', #18289 ) ;
#21386=CARTESIAN_POINT ( 'NONE',  ( -105.4334892372614121, 71.72994009789537984, 31.36525700924958926 ) ) ;
#21407=EDGE_CURVE ( 'NONE', #6632, #8624, #9446, .T. ) ;
#21411=CIRCLE ( 'NONE', #17408, 2.000000000000004885 ) ;
#21412=CARTESIAN_POINT ( 'NONE',  ( -92.53737097235195108, 79.85828562204767422, -28.87839056718415875 ) ) ;
#21413=ORIENTED_EDGE ( 'NONE', *, *, #17199, .F. ) ;
#21429=ORIENTED_EDGE ( 'NONE', *, *, #18247, .F. ) ;
#21435=CARTESIAN_POINT ( 'NONE',  ( -92.43457499998878291, 77.12912189496640281, 31.19724316448926871 ) ) ;
#21437=ORIENTED_EDGE ( 'NONE', *, *, #7978, .T. ) ;
#21438=CARTESIAN_POINT ( 'NONE',  ( -41.59208321381909457, 69.99999999999998579, -84.46951292587610283 ) ) ;
#21441=DIRECTION ( 'NONE',  ( -0.9999164797902015955, 0.000000000000000000, 0.01292414190464131335 ) ) ;
#21444=ORIENTED_EDGE ( 'NONE', *, *, #11084, .F. ) ;
#21446=( BOUNDED_SURFACE ( )  B_SPLINE_SURFACE ( 1, 3, ( 
 ( #3244, #18878, #11893, #15683 ),
 ( #15349, #4736, #15575, #8217 ) ),
 .UNSPECIFIED., .F., .F., .T. ) 
 B_SPLINE_SURFACE_WITH_KNOTS ( ( 2, 2 ),
 ( 4, 4 ),
 ( 0.000000000000000000, 1.000000000000000000 ),
 ( 0.000000000000000000, 1.000000000000000000 ),
 .UNSPECIFIED. ) 
 GEOMETRIC_REPRESENTATION_ITEM ( )  RATIONAL_B_SPLINE_SURFACE ( (
 ( 1.000000000000000000, 0.9999999775413713765, 0.9999999775413713765, 1.000000000000000000),
 ( 1.000000000000000000, 0.9999999775413713765, 0.9999999775413713765, 1.000000000000000000) ) ) 
 REPRESENTATION_ITEM ( '' )  SURFACE ( )  );
#21451=CARTESIAN_POINT ( 'NONE',  ( -0.4135725409485391246, 69.99999999999998579, -31.99732735328654343 ) ) ;
#21468=CARTESIAN_POINT ( 'NONE',  ( -88.17722787152888486, 89.00271273184408471, 51.54359545513624141 ) ) ;
#21477=CARTESIAN_POINT ( 'NONE',  ( -90.55526626895678532, 99.16641366430590665, -62.44901868852807070 ) ) ;
#21479=CARTESIAN_POINT ( 'NONE',  ( 91.23603883849617091, 78.43035437438882695, 30.82342686631245243 ) ) ;
#21495=ORIENTED_EDGE ( 'NONE', *, *, #5379, .F. ) ;
#21496=CARTESIAN_POINT ( 'NONE',  ( -84.45439400451301992, 75.03386225069931470, -1.459998722890992529 ) ) ;
#21497=CARTESIAN_POINT ( 'NONE',  ( -90.13473535659075253, 88.31972838967021744, 52.90262112213743251 ) ) ;
#21511=ORIENTED_EDGE ( 'NONE', *, *, #3564, .F. ) ;
#21514=ORIENTED_EDGE ( 'NONE', *, *, #3040, .F. ) ;
#21517=ADVANCED_FACE ( 'NONE', ( #8619 ), #15327, .F. ) ;
#21519=CARTESIAN_POINT ( 'NONE',  ( 75.04638230800617293, 75.00896870829117802, -2.285242870542876670 ) ) ;
#21520=CARTESIAN_POINT ( 'NONE',  ( -90.69261420090155923, 70.46556216177638987, 63.01891427407564095 ) ) ;
#21531=CARTESIAN_POINT ( 'NONE',  ( -90.73345939407629146, 80.10652859373118417, 31.90946778207756651 ) ) ;
#21532=DIRECTION ( 'NONE',  ( -0.9999164797902015955, 0.000000000000000000, 0.01292414190464174703 ) ) ;
#21534=EDGE_CURVE ( 'NONE', #13344, #14492, #20911, .T. ) ;
#21536=EDGE_CURVE ( 'NONE', #11196, #7781, #11022, .T. ) ;
#21537=CYLINDRICAL_SURFACE ( 'NONE', #15446, 2.000000000000004885 ) ;
#21540=ORIENTED_EDGE ( 'NONE', *, *, #5822, .F. ) ;
#21544=FACE_OUTER_BOUND ( 'NONE', #18036, .T. ) ;
#21546=EDGE_CURVE ( 'NONE', #4404, #18312, #5634, .T. ) ;
#21564=EDGE_CURVE ( 'NONE', #7316, #4942, #14167, .T. ) ;
#21567=CARTESIAN_POINT ( 'NONE',  ( -88.17830160593697997, 89.00999716261956962, 51.42151637835925726 ) ) ;
#21577=CARTESIAN_POINT ( 'NONE',  ( 93.58499681124563097, 69.99999999999998579, 57.80872228166916926 ) ) ;
#21578=CARTESIAN_POINT ( 'NONE',  ( -90.13422078941495386, 99.92632882282082107, -63.05520142610598811 ) ) ;
#21579=ORIENTED_EDGE ( 'NONE', *, *, #2179, .T. ) ;
#21580=CARTESIAN_POINT ( 'NONE',  ( 91.92156639752096225, 77.41735670888593290, 29.28407961425095962 ) ) ;
#21581=ORIENTED_EDGE ( 'NONE', *, *, #12030, .T. ) ;
#21590=CARTESIAN_POINT ( 'NONE',  ( -91.62437796271721879, 72.00000000000000000, -60.86849236629028326 ) ) ;
#21598=CARTESIAN_POINT ( 'NONE',  ( -81.25051790709260047, 75.12836414114961769, 5.987897703801240645 ) ) ;
#21599=CARTESIAN_POINT ( 'NONE',  ( -90.16949869353247493, 87.13201789581339085, 51.31799079330890123 ) ) ;
#21601=VERTEX_POINT ( 'NONE', #17603 ) ;
#21603=EDGE_CURVE ( 'NONE', #21849, #19075, #7780, .T. ) ;
#21606=CARTESIAN_POINT ( 'NONE',  ( -90.40889375659909888, 72.00000000000000000, 33.17122784026039284 ) ) ;
#21607=DIRECTION ( 'NONE',  ( -2.025474946048326158E-22, 1.000000000000000000, -1.876735158486678933E-22 ) ) ;
#21613=CARTESIAN_POINT ( 'NONE',  ( 69.43142427201327394, 92.58578643762697880, -85.31868097644085935 ) ) ;
#21620=SPHERICAL_SURFACE ( 'NONE', #12052, 2.000000000000000000 ) ;
#21623=CARTESIAN_POINT ( 'NONE',  ( -79.99331838321612054, 54.99999999999999289, 1.033931352371344481 ) ) ;
#21626=CARTESIAN_POINT ( 'NONE',  ( -2.067862704742604141, 72.00000000000000000, -159.9866367664322979 ) ) ;
#21627=CARTESIAN_POINT ( 'NONE',  ( -88.72304114575449319, 70.71205020914676709, 62.85437454899338405 ) ) ;
#21633=AXIS2_PLACEMENT_3D ( 'NONE', #19546, #19869, #5866 ) ;
#21635=DIRECTION ( 'NONE',  ( 0.01292414190464131508, 0.000000000000000000, 0.9999164797902017066 ) ) ;
#21638=LINE ( 'NONE', #6396, #15234 ) ;
#21641=CARTESIAN_POINT ( 'NONE',  ( -89.23446290093953337, 79.53212074382820163, 30.14913290299145388 ) ) ;
#21648=VERTEX_POINT ( 'NONE', #19537 ) ;
#21653=CARTESIAN_POINT ( 'NONE',  ( 79.90518398323666815, 100.1635695855008095, 75.81005614957788907 ) ) ;
#21661=ORIENTED_EDGE ( 'NONE', *, *, #1489, .F. ) ;
#21666=CIRCLE ( 'NONE', #5166, 2.000000000000004441 ) ;
#21669=ORIENTED_EDGE ( 'NONE', *, *, #1542, .T. ) ;
#21697=CARTESIAN_POINT ( 'NONE',  ( 89.66113247980437961, 100.6041916471017856, 63.72504470331089266 ) ) ;
#21698=CARTESIAN_POINT ( 'NONE',  ( -89.90836385050330648, 100.2819950034555205, -63.37719018575656094 ) ) ;
#21707=ORIENTED_EDGE ( 'NONE', *, *, #5822, .T. ) ;
#21710=ORIENTED_EDGE ( 'NONE', *, *, #12469, .T. ) ;
#21718=CARTESIAN_POINT ( 'NONE',  ( -79.92740525950245001, 75.13699351169597662, 6.133505399301365735 ) ) ;
#21721=VECTOR ( 'NONE', #19948, 1000.000000000000114 ) ;
#21735=EDGE_CURVE ( 'NONE', #10387, #12053, #9537, .T. ) ;
#21738=EDGE_LOOP ( 'NONE', ( #7591, #11162, #17510, #18060 ) ) ;
#21739=CARTESIAN_POINT ( 'NONE',  ( 37.51330139321492396, 69.99999999999998579, -87.03232607370792095 ) ) ;
#21742=LINE ( 'NONE', #2588, #4559 ) ;
#21744=CARTESIAN_POINT ( 'NONE',  ( 79.72645225953733927, 75.13699351169597662, 4.069943940015851247 ) ) ;
#21753=CARTESIAN_POINT ( 'NONE',  ( 89.63665673671270895, 97.44507682733028275, -63.75962087488073848 ) ) ;
#21755=CARTESIAN_POINT ( 'NONE',  ( 68.68766895589033084, 71.65104882840748246, -85.91861595181279654 ) ) ;
#21756=CARTESIAN_POINT ( 'NONE',  ( 91.65210746689167820, 71.62127171602892872, 60.82679172889523045 ) ) ;
#21759=ORIENTED_EDGE ( 'NONE', *, *, #880, .F. ) ;
#21767=ORIENTED_EDGE ( 'NONE', *, *, #14311, .T. ) ;
#21771=VECTOR ( 'NONE', #22004, 1000.000000000000114 ) ;
#21776=ORIENTED_EDGE ( 'NONE', *, *, #15275, .T. ) ;
#21780=LINE ( 'NONE', #6067, #5380 ) ;
#21785=CARTESIAN_POINT ( 'NONE',  ( -0.5690403138955768547, 86.15674685880075856, 75.02401767694439627 ) ) ;
#21787=ORIENTED_EDGE ( 'NONE', *, *, #12940, .F. ) ;
#21793=CARTESIAN_POINT ( 'NONE',  ( -88.90404157702997168, 89.05586475019977399, 50.97367400307179963 ) ) ;
#21797=CARTESIAN_POINT ( 'NONE',  ( 90.85853474116410666, 77.59429383720569717, -31.92673238494557353 ) ) ;
#21798=EDGE_LOOP ( 'NONE', ( #3717, #9685, #21282, #19659 ) ) ;
#21811=VERTEX_POINT ( 'NONE', #19860 ) ;
#21813=DIRECTION ( 'NONE',  ( -0.9999164797902015955, -2.001050586450180341E-22, 0.01292414190464038874 ) ) ;
#21823=CARTESIAN_POINT ( 'NONE',  ( -82.48914589713568546, 75.10304909037272125, 5.494148405572993887 ) ) ;
#21824=CARTESIAN_POINT ( 'NONE',  ( -90.17266153500538906, 87.07308075466939101, 51.35371910215589253 ) ) ;
#21826=ORIENTED_EDGE ( 'NONE', *, *, #16705, .F. ) ;
#21831=CARTESIAN_POINT ( 'NONE',  ( -39.10370113527942237, 92.00280690324824207, -83.45957852173413016 ) ) ;
#21839=CARTESIAN_POINT ( 'NONE',  ( 23.05638568958544710, 89.37982582623894245, -78.77076284602109979 ) ) ;
#21843=EDGE_CURVE ( 'NONE', #369, #20892, #11080, .T. ) ;
#21849=VERTEX_POINT ( 'NONE', #11843 ) ;
#21852=EDGE_LOOP ( 'NONE', ( #1122, #2800, #12612, #14877 ) ) ;
#21864=CARTESIAN_POINT ( 'NONE',  ( 91.76144944056427732, 79.85812038789160283, -31.26012496009718333 ) ) ;
#21888=CARTESIAN_POINT ( 'NONE',  ( -106.7230861007157756, 79.13476608364851472, -26.64972274501326055 ) ) ;
#21890=CARTESIAN_POINT ( 'NONE',  ( 64.07473967894682687, 105.0000000000000000, -72.00569783435743432 ) ) ;
#21891=CARTESIAN_POINT ( 'NONE',  ( -2.888085112683865585, 86.22276635713151904, 75.12774216256403292 ) ) ;
#21893=VERTEX_POINT ( 'NONE', #11612 ) ;
#21902=CARTESIAN_POINT ( 'NONE',  ( -89.81568892019076600, 87.99790937754146114, 50.78728647262676787 ) ) ;
#21904=CIRCLE ( 'NONE', #2127, 6.499999999999998224 ) ;
#21905=ORIENTED_EDGE ( 'NONE', *, *, #4286, .F. ) ;
#21909=ORIENTED_EDGE ( 'NONE', *, *, #12907, .F. ) ;
#21912=EDGE_LOOP ( 'NONE', ( #5061, #15224, #2077, #572 ) ) ;
#21916=ORIENTED_EDGE ( 'NONE', *, *, #5894, .T. ) ;
#21920=CARTESIAN_POINT ( 'NONE',  ( 85.84563054365274581, 105.0000000000000142, 68.77965573371083963 ) ) ;
#21931=CARTESIAN_POINT ( 'NONE',  ( -90.16809648441123670, 87.14955667014993423, 51.30734591929146404 ) ) ;
#21936=CARTESIAN_POINT ( 'NONE',  ( 1.717753310876226625, 55.00000000000000000, 109.6869605904137330 ) ) ;
#21940=CARTESIAN_POINT ( 'NONE',  ( -88.18626700604421842, 88.78700735547668899, 50.43357012433555298 ) ) ;
#21941=CARTESIAN_POINT ( 'NONE',  ( 79.92740525950247843, 55.00000000000000000, -6.133505399301337313 ) ) ;
#21942=DIRECTION ( 'NONE',  ( -0.009138748381789078140, 0.7071067811865487940, -0.7070477234798315802 ) ) ;
#21948=CARTESIAN_POINT ( 'NONE',  ( -70.91392079944854743, 72.00000000000000000, -84.09052168258642723 ) ) ;
#21959=DIRECTION ( 'NONE',  ( -2.025474946048326158E-22, 1.000000000000000000, -1.876735158486679638E-22 ) ) ;
#21960=ADVANCED_FACE ( 'NONE', ( #4799 ), #13348, .F. ) ;
#21964=CARTESIAN_POINT ( 'NONE',  ( 78.28083514950689903, 75.12313863457447383, -5.849292866322538309 ) ) ;
#21965=CARTESIAN_POINT ( 'NONE',  ( -89.67405064417086180, 69.73069950987664356, 63.42040036413745696 ) ) ;
#21967=CARTESIAN_POINT ( 'NONE',  ( -110.0212991616528768, 74.99906874937914836, -0.8747890471060359996 ) ) ;
#21974=CARTESIAN_POINT ( 'NONE',  ( -68.71681667565952978, 72.00000000000000000, 85.89527988174785378 ) ) ;
#21978=EDGE_CURVE ( 'NONE', #20892, #12459, #6765, .T. ) ;
#21979=CARTESIAN_POINT ( 'NONE',  ( 90.67285013207080624, 77.76891457534604513, -32.19520807900808279 ) ) ;
#21980=CIRCLE ( 'NONE', #12114, 2.000000000000004885 ) ;
#21981=CARTESIAN_POINT ( 'NONE',  ( -88.23797876370683468, 94.47357722488187903, 47.15541951427123024 ) ) ;
#21990=EDGE_CURVE ( 'NONE', #22275, #5033, #5026, .T. ) ;
#21991=VECTOR ( 'NONE', #13272, 1000.000000000000114 ) ;
#21993=CIRCLE ( 'NONE', #17255, 109.9999999999999858 ) ;
#21998=CARTESIAN_POINT ( 'NONE',  ( -64.32311159746099349, 87.99029836822310813, 52.78963101368245248 ) ) ;
#22003=DIRECTION ( 'NONE',  ( 0.9999164797902015955, 2.001050586450179636E-22, -0.01292414190464084844 ) ) ;
#22004=DIRECTION ( 'NONE',  ( 0.9999164797902015955, 2.001050586450177755E-22, -0.01292414190464177999 ) ) ;
#22008=AXIS2_PLACEMENT_3D ( 'NONE', #6840, #19126, #19011 ) ;
#22015=ORIENTED_EDGE ( 'NONE', *, *, #8750, .F. ) ;
#22019=ORIENTED_EDGE ( 'NONE', *, *, #14300, .T. ) ;
#22023=CARTESIAN_POINT ( 'NONE',  ( 90.40889375659912730, 78.43035437438885538, -33.17122784026042837 ) ) ;
#22031=CARTESIAN_POINT ( 'NONE',  ( -105.4334892372614121, 77.12912189496637438, 31.36525700924958926 ) ) ;
#22038=DIRECTION ( 'NONE',  ( -2.025474946048326158E-22, 1.000000000000000000, -1.876735158486678933E-22 ) ) ;
#22045=ADVANCED_FACE ( 'NONE', ( #19389 ), #1945, .T. ) ;
#22047=EDGE_CURVE ( 'NONE', #20235, #8789, #12178, .T. ) ;
#22052=CARTESIAN_POINT ( 'NONE',  ( -88.16496929303228569, 88.40829394340927649, 52.78344489490578439 ) ) ;
#22053=AXIS2_PLACEMENT_3D ( 'NONE', #19639, #17849, #21245 ) ;
#22059=CARTESIAN_POINT ( 'NONE',  ( -88.18538491329667295, 88.84369698205085797, 50.55255461122708027 ) ) ;
#22060=CARTESIAN_POINT ( 'NONE',  ( -91.93574473583122142, 79.05185923607193388, 28.63941780214905108 ) ) ;
#22061=CIRCLE ( 'NONE', #2280, 110.0000000000000000 ) ;
#22067=CARTESIAN_POINT ( 'NONE',  ( 1.364374947835851710E-14, 55.00000000000000000, -9.836440897896405351E-15 ) ) ;
#22082=CARTESIAN_POINT ( 'NONE',  ( -2.067862704742604141, 72.00000000000000000, -159.9866367664322979 ) ) ;
#22085=CARTESIAN_POINT ( 'NONE',  ( 105.8287943736950609, 79.03195428549129531, -30.00479353936319882 ) ) ;
#22097=CARTESIAN_POINT ( 'NONE',  ( 92.19651396575548574, 79.04398536194628377, -28.61663131200300469 ) ) ;
#22109=CYLINDRICAL_SURFACE ( 'NONE', #4463, 95.00000000000004263 ) ;
#22112=EDGE_CURVE ( 'NONE', #20716, #13764, #21000, .T. ) ;
#22119=ADVANCED_FACE ( 'NONE', ( #7106 ), #222, .T. ) ;
#22121=CARTESIAN_POINT ( 'NONE',  ( -106.8361484267444723, 79.08880628745897923, -26.19276530885237975 ) ) ;
#22130=EDGE_CURVE ( 'NONE', #19552, #591, #5366, .T. ) ;
#22131=CARTESIAN_POINT ( 'NONE',  ( 79.99331838321614896, 54.99999999999999289, -1.033931352371314949 ) ) ;
#22135=VECTOR ( 'NONE', #2801, 1000.000000000000114 ) ;
#22146=DIRECTION ( 'NONE',  ( -2.025474946048326158E-22, 1.000000000000000000, -1.876735158486679638E-22 ) ) ;
#22160=CARTESIAN_POINT ( 'NONE',  ( 106.2089377515399491, 71.86507807689919503, 28.62973177816241588 ) ) ;
#22171=CARTESIAN_POINT ( 'NONE',  ( -88.16451018535700257, 88.36589127631114593, 52.82384857957035251 ) ) ;
#22179=CARTESIAN_POINT ( 'NONE',  ( 1.121675378414710433, 45.00000000000000000, 109.9942809619911799 ) ) ;
#22180=CARTESIAN_POINT ( 'NONE',  ( -88.18349247326855789, 88.93254284115897690, 50.79801752376152990 ) ) ;
#22181=CARTESIAN_POINT ( 'NONE',  ( -89.41602473586596034, 79.46258270018842040, 29.93333348547115236 ) ) ;
#22187=CARTESIAN_POINT ( 'NONE',  ( -88.05170339851980543, 72.97786998644572520, 61.56719313945616534 ) ) ;
#22189=CARTESIAN_POINT ( 'NONE',  ( -92.05960170301050027, 69.99999999999998579, 60.20821982323565180 ) ) ;
#22192=CARTESIAN_POINT ( 'NONE',  ( 90.55526626895685638, 99.16641366430587823, 62.44901868852801385 ) ) ;
#22193=VECTOR ( 'NONE', #1272, 1000.000000000000000 ) ;
#22196=CARTESIAN_POINT ( 'NONE',  ( -64.00797876747101611, 100.1288551967107310, 77.17086362122255139 ) ) ;
#22197=ORIENTED_EDGE ( 'NONE', *, *, #6946, .T. ) ;
#22198=ORIENTED_EDGE ( 'NONE', *, *, #20974, .T. ) ;
#22199=ORIENTED_EDGE ( 'NONE', *, *, #15570, .T. ) ;
#22202=CARTESIAN_POINT ( 'NONE',  ( -38.89810712971357987, 72.00000000000000000, 85.50986645835278921 ) ) ;
#22204=CARTESIAN_POINT ( 'NONE',  ( -109.5708359150299742, 75.34617192694386745, 10.75083194752825477 ) ) ;
#22206=CARTESIAN_POINT ( 'NONE',  ( -91.65210746689160715, 71.62127171602891451, -60.82679172889525177 ) ) ;
#22212=CARTESIAN_POINT ( 'NONE',  ( 92.50365291375123888, 70.32755610701406113, 59.52398455131074684 ) ) ;
#22218=CARTESIAN_POINT ( 'NONE',  ( -1.163172771417704698, 69.99999999999998579, -89.99248318111816047 ) ) ;
#22223=EDGE_CURVE ( 'NONE', #13316, #6274, #4415, .T. ) ;
#22233=ORIENTED_EDGE ( 'NONE', *, *, #13685, .F. ) ;
#22234=CARTESIAN_POINT ( 'NONE',  ( 0.4135725409484927173, 69.99999999999998579, 31.99732735328655053 ) ) ;
#22239=EDGE_CURVE ( 'NONE', #10097, #13377, #11557, .T. ) ;
#22242=DIRECTION ( 'NONE',  ( 0.8909995034498461308, 2.656742962652179567E-22, 0.4540042784513463880 ) ) ;
#22244=CYLINDRICAL_SURFACE ( 'NONE', #19875, 2.000000000000001332 ) ;
#22255=ORIENTED_EDGE ( 'NONE', *, *, #2325, .F. ) ;
#22257=CARTESIAN_POINT ( 'NONE',  ( 34.11225069749755079, 94.37751527644310556, -83.07029434066950557 ) ) ;
#22261=CARTESIAN_POINT ( 'NONE',  ( 106.1519489938926029, 71.09828217887417168, 28.84036442345823303 ) ) ;
#22271=AXIS2_PLACEMENT_3D ( 'NONE', #10130, #11628, #15087 ) ;
#22272=LINE ( 'NONE', #13581, #8386 ) ;
#22273=CARTESIAN_POINT ( 'NONE',  ( -88.16376355711264523, 88.29301322969513421, 52.88806878750047247 ) ) ;
#22275=VERTEX_POINT ( 'NONE', #21974 ) ;
#22279=CARTESIAN_POINT ( 'NONE',  ( -34.02129075419646398, 93.60252210245951687, 83.02806418447188719 ) ) ;
#22280=FACE_OUTER_BOUND ( 'NONE', #20645, .T. ) ;
#22287=CARTESIAN_POINT ( 'NONE',  ( 65.90110554552376243, 105.0000000000000000, 69.29678410920483600 ) ) ;
#22290=CARTESIAN_POINT ( 'NONE',  ( 1.364374644014609697E-14, 69.99999999999998579, -9.836443712999143722E-15 ) ) ;
#22298=ORIENTED_EDGE ( 'NONE', *, *, #18395, .F. ) ;
#22299=DIRECTION ( 'NONE',  ( -0.01292414190463832269, 0.000000000000000000, -0.9999164797902017066 ) ) ;
#22300=EDGE_CURVE ( 'NONE', #4942, #20544, #4979, .T. ) ;
#22303=ORIENTED_EDGE ( 'NONE', *, *, #14765, .F. ) ;
#22316=CARTESIAN_POINT ( 'NONE',  ( -41.58451242677338655, 92.58578643762699301, -83.88377541325537834 ) ) ;
#22320=DIRECTION ( 'NONE',  ( -2.025474946048326158E-22, 1.000000000000000000, -1.876735158486678933E-22 ) ) ;
#22332=ORIENTED_EDGE ( 'NONE', *, *, #496, .T. ) ;
#22333=VECTOR ( 'NONE', #692, 1000.000000000000114 ) ;
#22335=LINE ( 'NONE', #17327, #3663 ) ;
#22349=CARTESIAN_POINT ( 'NONE',  ( 92.05960170301050027, 69.99999999999998579, -60.20821982323567312 ) ) ;
#22350=TOROIDAL_SURFACE ( 'NONE', #6966, 83.00000000000001421, 2.000000000000000000 ) ;
#22353=CARTESIAN_POINT ( 'NONE',  ( -38.46706438352714486, 91.17157287525387233, 85.27439087629285552 ) ) ;
#22355=DIRECTION ( 'NONE',  ( 0.01292414190464131508, 0.000000000000000000, 0.9999164797902017066 ) ) ;
#22358=AXIS2_PLACEMENT_3D ( 'NONE', #1898, #1783, #9233 ) ;
#22363=CARTESIAN_POINT ( 'NONE',  ( -90.11270991033710231, 87.45691446470777919, 51.12027952437478717 ) ) ;
#22368=DIRECTION ( 'NONE',  ( 0.9999164797902017066, 2.001050586450178931E-22, -0.01292414190464131508 ) ) ;
#22371=EDGE_CURVE ( 'NONE', #10181, #19868, #13610, .T. ) ;
#22373=FACE_OUTER_BOUND ( 'NONE', #17794, .T. ) ;
#22376=VERTEX_POINT ( 'NONE', #21152 ) ;
#22379=VERTEX_POINT ( 'NONE', #14175 ) ;
#22383=CARTESIAN_POINT ( 'NONE',  ( -88.16473883906751041, 88.38724588659185599, 52.80379687237449815 ) ) ;
#22384=EDGE_CURVE ( 'NONE', #1394, #9371, #18184, .T. ) ;
#22390=CARTESIAN_POINT ( 'NONE',  ( -74.93579704394247187, 95.43814120535131451, 80.52726847798278698 ) ) ;
#22392=CARTESIAN_POINT ( 'NONE',  ( 39.36913080622081651, 69.99999999999998579, -87.51612159803863733 ) ) ;
#22393=CARTESIAN_POINT ( 'NONE',  ( -22.89256597249752545, 88.79858284056908246, -77.57367698057866789 ) ) ;
#22394=( NAMED_UNIT ( * ) SI_UNIT ( $, .STERADIAN. ) SOLID_ANGLE_UNIT ( ) );
#22397=CARTESIAN_POINT ( 'NONE',  ( -71.18985671402974447, 92.11167198312699611, -83.85708946072359993 ) ) ;
#22401=ORIENTED_EDGE ( 'NONE', *, *, #4262, .T. ) ;
#22405=CARTESIAN_POINT ( 'NONE',  ( -90.03465221005033925, 70.01281497139055432, 63.19621350536183968 ) ) ;
#22407=CARTESIAN_POINT ( 'NONE',  ( -2.067862704742604141, 69.99999999999998579, -159.9866367664322979 ) ) ;
#22413=CIRCLE ( 'NONE', #21329, 112.5000000000000284 ) ;
#22414=CARTESIAN_POINT ( 'NONE',  ( -64.00442900045042904, 100.0478588994083964, 77.44550239952441473 ) ) ;
#22418=ADVANCED_FACE ( 'NONE', ( #8973 ), #3812, .F. ) ;
#22423=CARTESIAN_POINT ( 'NONE',  ( -90.22705529645503475, 71.16332133347465572, 60.80384032246523418 ) ) ;
#22431=DIRECTION ( 'NONE',  ( 0.01292414190464174703, 0.000000000000000000, 0.9999164797902015955 ) ) ;
#22436=( BOUNDED_CURVE ( )  B_SPLINE_CURVE ( 3, ( #17331, #1588, #5237, #19141 ),
 .UNSPECIFIED., .F., .T. ) 
 B_SPLINE_CURVE_WITH_KNOTS ( ( 4, 4 ),
 ( 0.4472747960204455087, 0.4841788640348455020 ),
 .UNSPECIFIED. ) 
 CURVE ( )  GEOMETRIC_REPRESENTATION_ITEM ( )  RATIONAL_B_SPLINE_CURVE ( ( 1.000000000000000000, 0.9998865107004337727, 0.9998865107004337727, 1.000000000000000000 ) ) 
 REPRESENTATION_ITEM ( '' )  );
#22438=CIRCLE ( 'NONE', #10731, 1.999999999999997780 ) ;
#22444=EDGE_CURVE ( 'NONE', #19328, #10450, #4139, .T. ) ;
#22448=ORIENTED_EDGE ( 'NONE', *, *, #2258, .T. ) ;
#22462=ORIENTED_EDGE ( 'NONE', *, *, #15315, .T. ) ;
#22463=DIRECTION ( 'NONE',  ( -2.025474946048326158E-22, 1.000000000000000000, -1.876735158486679638E-22 ) ) ;
#22482=CARTESIAN_POINT ( 'NONE',  ( -87.76353177753581747, 103.0887459898907821, -66.33296338796036196 ) ) ;
#22493=CARTESIAN_POINT ( 'NONE',  ( 90.21557837424575155, 71.13279352004266798, -62.93780832164412686 ) ) ;
#22495=CARTESIAN_POINT ( 'NONE',  ( -90.07292945398545214, 88.55600042780055503, 52.68328250211072827 ) ) ;
#22503=CARTESIAN_POINT ( 'NONE',  ( 80.05923150692980528, 75.13699351169597662, 4.065642694558706083 ) ) ;
#22508=DIRECTION ( 'NONE',  ( 0.01292414190464131508, 0.000000000000000000, 0.9999164797902017066 ) ) ;
#22509=DIRECTION ( 'NONE',  ( -0.008205354412248759208, 0.7726059781012496464, -0.6348327927582039232 ) ) ;
#22527=ORIENTED_EDGE ( 'NONE', *, *, #19929, .F. ) ;
#22528=ADVANCED_FACE ( 'NONE', ( #11724 ), #2666, .T. ) ;
#22530=CARTESIAN_POINT ( 'NONE',  ( -89.87368547071935154, 72.07415593028026990, 62.10066946404283783 ) ) ;
#22537=EDGE_CURVE ( 'NONE', #10132, #15344, #20053, .T. ) ;
#22543=CARTESIAN_POINT ( 'NONE',  ( -91.24493283426484425, 78.25381457448439448, -30.56897831620035788 ) ) ;
#22553=CARTESIAN_POINT ( 'NONE',  ( 89.66113247980437961, 100.6041916471017856, 63.72504470331089266 ) ) ;
#22558=CARTESIAN_POINT ( 'NONE',  ( 1.163172771417732010, 69.99999999999998579, 89.99248318111813205 ) ) ;
#22561=CARTESIAN_POINT ( 'NONE',  ( 106.1636641531657972, 79.04398536104962147, -28.79715981783310497 ) ) ;
#22563=CARTESIAN_POINT ( 'NONE',  ( -75.90743353164272378, 96.21294322789842113, -79.81268430165903283 ) ) ;
#22567=CARTESIAN_POINT ( 'NONE',  ( 35.39322062607229213, 92.77591188308413450, -83.66707218845637328 ) ) ;
#22571=ADVANCED_FACE ( 'NONE', ( #4254 ), #4691, .T. ) ;
#22578=CARTESIAN_POINT ( 'NONE',  ( 68.43148148480361215, 69.99999999999998579, 86.12277481476651531 ) ) ;
#22586=CARTESIAN_POINT ( 'NONE',  ( -89.07320425719680657, 88.54727852611058836, 50.44093601027914531 ) ) ;
#22588=SHAPE_REPRESENTATION_RELATIONSHIP ( 'NONE' , 'NONE' ,  #10922, #19533 ) ;
#22589=CARTESIAN_POINT ( 'NONE',  ( 106.2142196127746132, 77.44923501812733946, 28.61015647369538684 ) ) ;
#22591=CARTESIAN_POINT ( 'NONE',  ( 40.65822637310714782, 91.17157287525387233, 84.25167897319538213 ) ) ;
#22600=CARTESIAN_POINT ( 'NONE',  ( -89.96085446817751574, 87.79024195230550731, 50.91569201083114393 ) ) ;
#22606=DIRECTION ( 'NONE',  ( 0.009138748381789112835, -0.7071067811865462405, 0.7070477234798342447 ) ) ;
#22608=CARTESIAN_POINT ( 'NONE',  ( 84.66884248357162335, 75.02317907734844482, 1.009935179570716546 ) ) ;
#22613=CARTESIAN_POINT ( 'NONE',  ( -65.62836707099317834, 91.01435578462051978, 67.50627132372665073 ) ) ;
#22618=VERTEX_POINT ( 'NONE', #15201 ) ;
#22619=DIRECTION ( 'NONE',  ( -0.004263634442766561783, 0.9440169652124852373, -0.3298693541575938859 ) ) ;
#22624=AXIS2_PLACEMENT_3D ( 'NONE', #17588, #13902, #14028 ) ;
#22625=DIRECTION ( 'NONE',  ( 2.025474946048326158E-22, -1.000000000000000000, 1.876735158486679638E-22 ) ) ;
#22629=CARTESIAN_POINT ( 'NONE',  ( -90.41395131934733342, 70.35743632279135795, 62.65252801945162275 ) ) ;
#22634=FACE_OUTER_BOUND ( 'NONE', #10179, .T. ) ;
#22640=DIRECTION ( 'NONE',  ( 0.01292414190464131682, 0.000000000000000000, 0.9999164797902017066 ) ) ;
#22642=EDGE_CURVE ( 'NONE', #4308, #15481, #12913, .T. ) ;
#22645=ORIENTED_EDGE ( 'NONE', *, *, #6175, .F. ) ;
#22651=ADVANCED_FACE ( 'NONE', ( #6339 ), #4594, .F. ) ;
#22660=ORIENTED_EDGE ( 'NONE', *, *, #3050, .T. ) ;
#22665=AXIS2_PLACEMENT_3D ( 'NONE', #5231, #12274, #19258 ) ;
ENDSEC;
END-ISO-10303-21;
